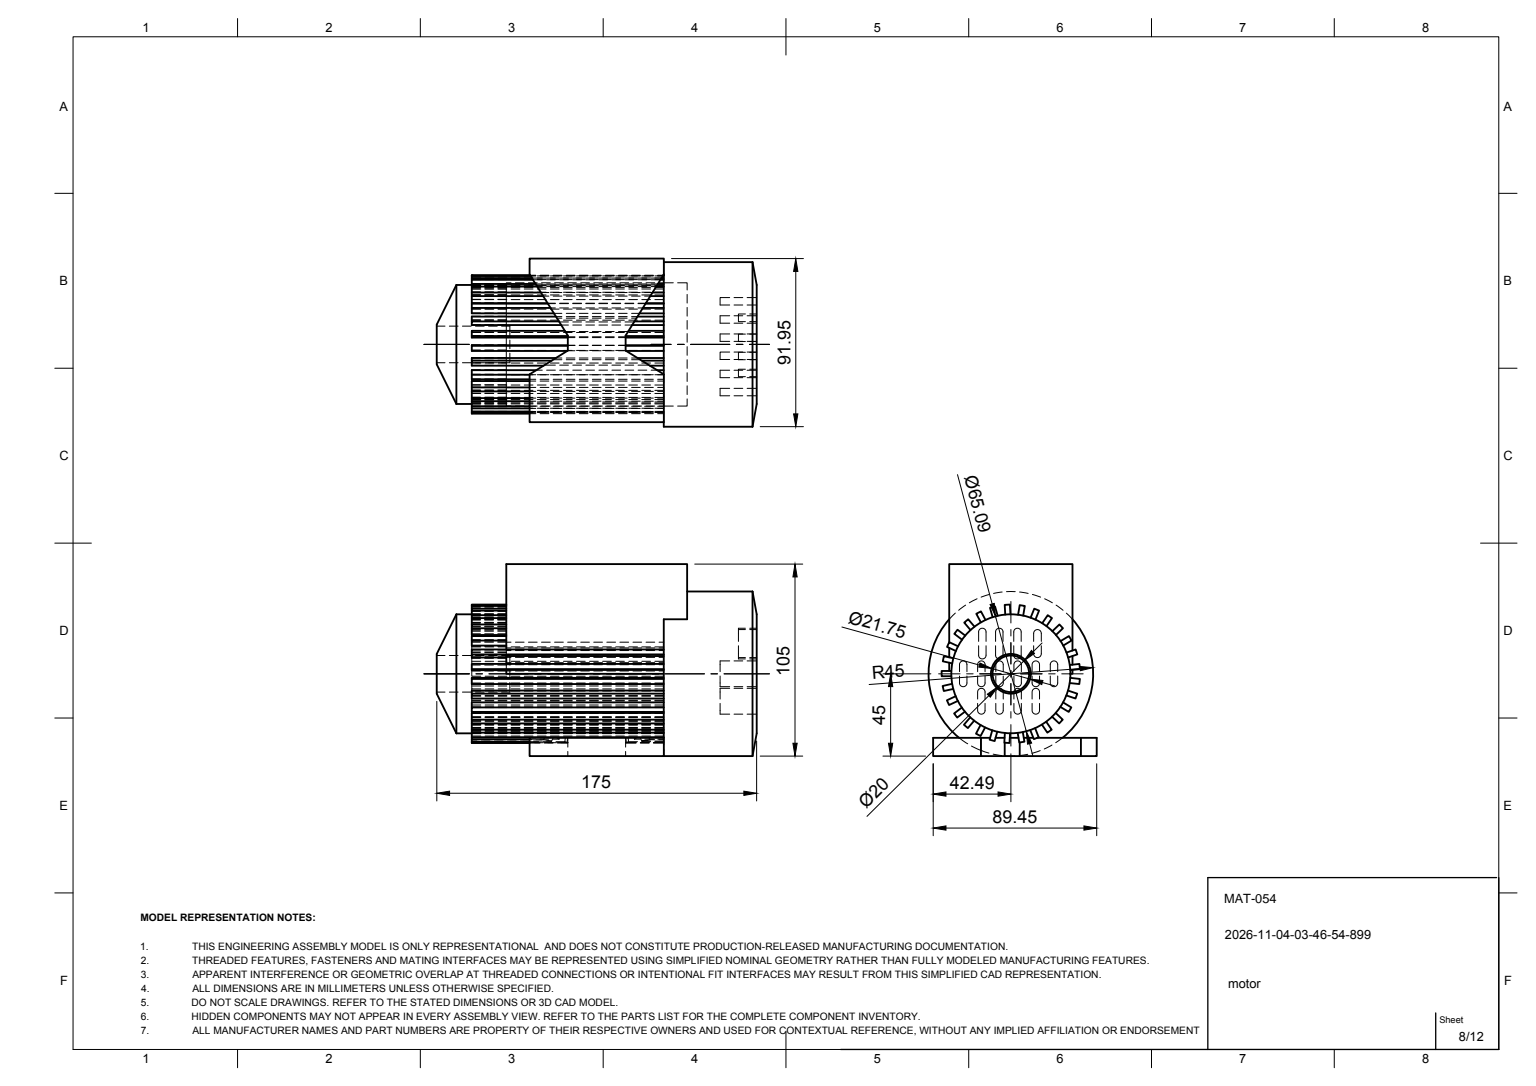
ISO-10303-21;
HEADER;
FILE_DESCRIPTION (('STEP AP214'),
    '1' );
FILE_NAME ('motor.step',
    '2026-10-21T17:50:41',
    ( '' ),
    ( '' ),
    'SwSTEP 2.0',
    'SolidWorks 2026',
    '' );
FILE_SCHEMA (( 'AUTOMOTIVE_DESIGN' ));
ENDSEC;

DATA;
#2=ORIENTED_EDGE ( 'NONE', *, *, #27963, .F. ) ;
#5=CARTESIAN_POINT ( 'NONE',  ( 15.44711578872680846, -28.64595934308655956, 68.31122994652405112 ) ) ;
#24=ADVANCED_FACE ( 'NONE', ( #3974 ), #8982, .F. ) ;
#30=CARTESIAN_POINT ( 'NONE',  ( -23.78520691327551972, 22.21414650552148728, 68.31122994652405112 ) ) ;
#31=EDGE_CURVE ( 'NONE', #27481, #20981, #20374, .T. ) ;
#32=LINE ( 'NONE', #10895, #9078 ) ;
#36=DIRECTION ( 'NONE',  ( -0.4198891015602645438, 0.9075754196709571175, 0.000000000000000000 ) ) ;
#44=CARTESIAN_POINT ( 'NONE',  ( -5.021133111225092982, -15.68591377522703745, -67.50000000000000000 ) ) ;
#46=LINE ( 'NONE', #29597, #32142 ) ;
#59=ORIENTED_EDGE ( 'NONE', *, *, #18290, .T. ) ;
#62=ORIENTED_EDGE ( 'NONE', *, *, #19345, .T. ) ;
#65=PLANE ( 'NONE',  #4223 ) ;
#67=AXIS2_PLACEMENT_3D ( 'NONE', #32973, #22315, #1132 ) ;
#69=ADVANCED_FACE ( 'NONE', ( #20027 ), #30867, .F. ) ;
#70=DIRECTION ( 'NONE',  ( -0.9766205557100867685, 0.2149704402110236834, 3.948942922735914076E-17 ) ) ;
#75=FACE_OUTER_BOUND ( 'NONE', #24485, .T. ) ;
#77=CARTESIAN_POINT ( 'NONE',  ( 3.235562306570555532E-30, -1.691831803474588058, -87.50000000000000000 ) ) ;
#85=AXIS2_PLACEMENT_3D ( 'NONE', #752, #27973, #1103 ) ;
#86=CARTESIAN_POINT ( 'NONE',  ( -20.02113311122498729, -5.758675521474015291, -67.50000000000000000 ) ) ;
#92=ORIENTED_EDGE ( 'NONE', *, *, #10815, .F. ) ;
#99=CARTESIAN_POINT ( 'NONE',  ( -45.00000000000000000, 16.36947364650383818, 36.69637551990492597 ) ) ;
#110=VECTOR ( 'NONE', #12286, 1000.000000000000227 ) ;
#121=EDGE_CURVE ( 'NONE', #19542, #7373, #4262, .T. ) ;
#122=CARTESIAN_POINT ( 'NONE',  ( -35.00000000000000000, -46.95407462254104303, -36.69637551990492597 ) ) ;
#126=LINE ( 'NONE', #30027, #31126 ) ;
#133=ORIENTED_EDGE ( 'NONE', *, *, #21122, .F. ) ;
#136=EDGE_LOOP ( 'NONE', ( #10690, #4855, #133, #33486, #30185, #13307, #10749, #25225 ) ) ;
#141=CARTESIAN_POINT ( 'NONE',  ( 28.11866956577618382, 16.38733641342591696, 68.31122994652405112 ) ) ;
#142=DIRECTION ( 'NONE',  ( 0.05413890858541774848, -0.9985334138511239299, -1.834276123671687566E-16 ) ) ;
#146=CARTESIAN_POINT ( 'NONE',  ( -9.978866888775527855, 8.235406450278430768, -87.50000000000000000 ) ) ;
#149=CARTESIAN_POINT ( 'NONE',  ( 3.235562306570555532E-30, 28.08988295778447508, -67.50000000000000000 ) ) ;
#150=EDGE_CURVE ( 'NONE', #25913, #33864, #29280, .T. ) ;
#158=VECTOR ( 'NONE', #14520, 1000.000000000000000 ) ;
#167=DIRECTION ( 'NONE',  ( 0.000000000000000000, 1.000000000000000000, 0.000000000000000000 ) ) ;
#177=ORIENTED_EDGE ( 'NONE', *, *, #24168, .F. ) ;
#180=FACE_OUTER_BOUND ( 'NONE', #24704, .T. ) ;
#189=AXIS2_PLACEMENT_3D ( 'NONE', #223, #13410, #11088 ) ;
#197=VECTOR ( 'NONE', #17016, 1000.000000000000000 ) ;
#200=CARTESIAN_POINT ( 'NONE',  ( -35.71762877834949990, -12.58147180936565057, -36.68877005347593467 ) ) ;
#214=CARTESIAN_POINT ( 'NONE',  ( -20.02113311122498729, -3.725253662474303784, -67.50000000000000000 ) ) ;
#215=LINE ( 'NONE', #29415, #4585 ) ;
#222=EDGE_CURVE ( 'NONE', #22062, #30310, #29769, .T. ) ;
#223=CARTESIAN_POINT ( 'NONE',  ( 0.000000000000000000, 3.524919873834583163E-15, 68.31122994652405112 ) ) ;
#232=EDGE_CURVE ( 'NONE', #29036, #32413, #15921, .T. ) ;
#243=CARTESIAN_POINT ( 'NONE',  ( 22.89764159710611224, 17.63622956525712127, -77.50000000000000000 ) ) ;
#244=ORIENTED_EDGE ( 'NONE', *, *, #13986, .T. ) ;
#252=ORIENTED_EDGE ( 'NONE', *, *, #16950, .T. ) ;
#253=EDGE_CURVE ( 'NONE', #5102, #23161, #21417, .T. ) ;
#254=CARTESIAN_POINT ( 'NONE',  ( 32.30227131129396412, -3.970848902647437395, 68.31122994652405112 ) ) ;
#255=DIRECTION ( 'NONE',  ( -0.3701381553399132329, -0.9289767198167918627, 0.000000000000000000 ) ) ;
#261=LINE ( 'NONE', #33170, #9980 ) ;
#268=CARTESIAN_POINT ( 'NONE',  ( 5.021133111224369117, -1.691831803474588058, -87.50000000000000000 ) ) ;
#269=CARTESIAN_POINT ( 'NONE',  ( 0.000000000000000000, 6.992329373473909019E-15, 49.43553178847298568 ) ) ;
#271=FACE_OUTER_BOUND ( 'NONE', #6766, .T. ) ;
#282=CARTESIAN_POINT ( 'NONE',  ( -35.00000000000000000, 0.000000000000000000, 0.000000000000000000 ) ) ;
#286=ORIENTED_EDGE ( 'NONE', *, *, #4793, .F. ) ;
#288=AXIS2_PLACEMENT_3D ( 'NONE', #34150, #4414, #26138 ) ;
#298=ORIENTED_EDGE ( 'NONE', *, *, #4872, .T. ) ;
#303=DIRECTION ( 'NONE',  ( -0.9985334138511239299, -0.05413890858541774848, -0.000000000000000000 ) ) ;
#308=ORIENTED_EDGE ( 'NONE', *, *, #21108, .F. ) ;
#311=DIRECTION ( 'NONE',  ( 0.000000000000000000, -0.000000000000000000, -1.000000000000000000 ) ) ;
#318=CARTESIAN_POINT ( 'NONE',  ( 32.40067729534749219, 3.066020821660472517, 68.31122994652405112 ) ) ;
#319=VERTEX_POINT ( 'NONE', #27272 ) ;
#323=EDGE_CURVE ( 'NONE', #17531, #2097, #46, .T. ) ;
#324=EDGE_CURVE ( 'NONE', #31410, #8890, #5192, .T. ) ;
#327=DIRECTION ( 'NONE',  ( -0.000000000000000000, -1.000000000000000000, -0.000000000000000000 ) ) ;
#331=ORIENTED_EDGE ( 'NONE', *, *, #24983, .F. ) ;
#336=ORIENTED_EDGE ( 'NONE', *, *, #6534, .F. ) ;
#340=CARTESIAN_POINT ( 'NONE',  ( 3.235562306570555532E-30, -1.691831803474591833, -67.50000000000000000 ) ) ;
#346=ORIENTED_EDGE ( 'NONE', *, *, #29604, .F. ) ;
#353=CARTESIAN_POINT ( 'NONE',  ( 5.021133111224679091, 26.05646109878476224, -67.50000000000000000 ) ) ;
#357=ORIENTED_EDGE ( 'NONE', *, *, #28689, .F. ) ;
#360=CYLINDRICAL_SURFACE ( 'NONE', #25416, 2.033421858999710619 ) ;
#361=EDGE_CURVE ( 'NONE', #12124, #30243, #11090, .T. ) ;
#363=ORIENTED_EDGE ( 'NONE', *, *, #34633, .T. ) ;
#369=CARTESIAN_POINT ( 'NONE',  ( 22.89764159710613001, 8.346743312457581609, -87.50000000000000000 ) ) ;
#371=PLANE ( 'NONE',  #32639 ) ;
#374=AXIS2_PLACEMENT_3D ( 'NONE', #31781, #29476, #5070 ) ;
#383=VECTOR ( 'NONE', #16250, 1000.000000000000114 ) ;
#394=CARTESIAN_POINT ( 'NONE',  ( -36.80830595996284416, 8.862931941313791029, -36.68877005347593467 ) ) ;
#399=DIRECTION ( 'NONE',  ( 0.000000000000000000, 1.836970198721029934E-16, -1.000000000000000000 ) ) ;
#409=CARTESIAN_POINT ( 'NONE',  ( -2.216215597024039141, -32.46987467335852529, 68.31122994652405112 ) ) ;
#410=AXIS2_PLACEMENT_3D ( 'NONE', #353, #702, #3357 ) ;
#412=ORIENTED_EDGE ( 'NONE', *, *, #6672, .F. ) ;
#415=EDGE_CURVE ( 'NONE', #2863, #31849, #8577, .T. ) ;
#419=VECTOR ( 'NONE', #14183, 1000.000000000000000 ) ;
#420=ORIENTED_EDGE ( 'NONE', *, *, #12622, .F. ) ;
#424=ORIENTED_EDGE ( 'NONE', *, *, #23285, .T. ) ;
#425=CARTESIAN_POINT ( 'NONE',  ( -18.45373714011839539, 26.80790850550480897, 68.31122994652405112 ) ) ;
#427=CIRCLE ( 'NONE', #22026, 10.00000000000000000 ) ;
#431=ORIENTED_EDGE ( 'NONE', *, *, #25232, .F. ) ;
#433=LINE ( 'NONE', #254, #17985 ) ;
#434=DIRECTION ( 'NONE',  ( 0.000000000000000000, 1.836970198721029441E-16, -1.000000000000000000 ) ) ;
#436=DIRECTION ( 'NONE',  ( -1.000000000000000000, 0.000000000000000000, 0.000000000000000000 ) ) ;
#439=VECTOR ( 'NONE', #21313, 1000.000000000000000 ) ;
#442=EDGE_CURVE ( 'NONE', #2071, #22576, #14652, .T. ) ;
#444=ORIENTED_EDGE ( 'NONE', *, *, #6797, .F. ) ;
#446=EDGE_CURVE ( 'NONE', #17949, #8883, #28157, .T. ) ;
#449=DIRECTION ( 'NONE',  ( 0.4198891015602635446, -0.9075754196709575616, -1.667188999027280528E-16 ) ) ;
#452=FACE_OUTER_BOUND ( 'NONE', #26260, .T. ) ;
#456=AXIS2_PLACEMENT_3D ( 'NONE', #31514, #16040, #10517 ) ;
#479=PLANE ( 'NONE',  #16043 ) ;
#484=DIRECTION ( 'NONE',  ( -1.000000000000000000, 0.000000000000000000, 0.000000000000000000 ) ) ;
#488=CARTESIAN_POINT ( 'NONE',  ( -32.54223829851967764, 0.4550817492056100644, 68.31122994652405112 ) ) ;
#489=ADVANCED_FACE ( 'NONE', ( #1969 ), #7124, .F. ) ;
#494=EDGE_CURVE ( 'NONE', #32940, #29402, #33851, .T. ) ;
#504=PLANE ( 'NONE',  #30798 ) ;
#511=AXIS2_PLACEMENT_3D ( 'NONE', #21319, #32167, #30028 ) ;
#522=EDGE_CURVE ( 'NONE', #24257, #22309, #20328, .T. ) ;
#523=ADVANCED_FACE ( 'NONE', ( #31345 ), #4279, .F. ) ;
#532=ORIENTED_EDGE ( 'NONE', *, *, #11905, .T. ) ;
#538=CARTESIAN_POINT ( 'NONE',  ( -10.84269519964070305, -36.27449394610876965, -36.68877005347593467 ) ) ;
#539=CARTESIAN_POINT ( 'NONE',  ( 14.14940496480368104, 33.69708579775584667, -36.68877005347592757 ) ) ;
#544=CARTESIAN_POINT ( 'NONE',  ( -9.144464960067640646, -31.23432620483743705, -36.68877005347593467 ) ) ;
#548=ORIENTED_EDGE ( 'NONE', *, *, #30977, .T. ) ;
#552=PRODUCT_CONTEXT ( 'NONE', #11461, 'mechanical' ) ;
#557=EDGE_CURVE ( 'NONE', #31368, #17595, #13969, .T. ) ;
#562=EDGE_LOOP ( 'NONE', ( #7226, #23075, #30348, #6330 ) ) ;
#565=EDGE_CURVE ( 'NONE', #34117, #30722, #12848, .T. ) ;
#572=PLANE ( 'NONE',  #2099 ) ;
#578=DIRECTION ( 'NONE',  ( 0.000000000000000000, 0.000000000000000000, 1.000000000000000000 ) ) ;
#584=VECTOR ( 'NONE', #33294, 1000.000000000000000 ) ;
#585=ORIENTED_EDGE ( 'NONE', *, *, #9500, .F. ) ;
#590=EDGE_LOOP ( 'NONE', ( #5300, #9615, #21290, #22102 ) ) ;
#592=LINE ( 'NONE', #30312, #24116 ) ;
#593=EDGE_CURVE ( 'NONE', #33757, #32360, #20496, .T. ) ;
#594=VERTEX_POINT ( 'NONE', #20673 ) ;
#609=DIRECTION ( 'NONE',  ( -0.000000000000000000, 1.836970198721029934E-16, -1.000000000000000000 ) ) ;
#611=ADVANCED_FACE ( 'NONE', ( #2493 ), #8368, .F. ) ;
#614=PLANE ( 'NONE',  #25375 ) ;
#616=LINE ( 'NONE', #2922, #2449 ) ;
#619=AXIS2_PLACEMENT_3D ( 'NONE', #1312, #12183, #23029 ) ;
#624=LINE ( 'NONE', #9159, #6292 ) ;
#631=EDGE_LOOP ( 'NONE', ( #17739, #3820, #7539, #1701 ) ) ;
#633=EDGE_LOOP ( 'NONE', ( #9077, #27367, #24881, #22906, #2998 ) ) ;
#634=EDGE_CURVE ( 'NONE', #13940, #4555, #21191, .T. ) ;
#635=EDGE_CURVE ( 'NONE', #21072, #3784, #32561, .T. ) ;
#640=VERTEX_POINT ( 'NONE', #13541 ) ;
#641=DIRECTION ( 'NONE',  ( -0.000000000000000000, 1.836970198721029934E-16, -1.000000000000000000 ) ) ;
#646=ORIENTED_EDGE ( 'NONE', *, *, #2039, .T. ) ;
#653=LINE ( 'NONE', #18869, #7882 ) ;
#659=ORIENTED_EDGE ( 'NONE', *, *, #951, .T. ) ;
#661=LINE ( 'NONE', #835, #20287 ) ;
#662=DIRECTION ( 'NONE',  ( 0.000000000000000000, 1.000000000000000000, 0.000000000000000000 ) ) ;
#663=AXIS2_PLACEMENT_3D ( 'NONE', #15533, #26376, #17867 ) ;
#675=VECTOR ( 'NONE', #22343, 1000.000000000000114 ) ;
#679=EDGE_CURVE ( 'NONE', #33018, #4776, #8184, .T. ) ;
#685=ORIENTED_EDGE ( 'NONE', *, *, #27268, .F. ) ;
#700=ORIENTED_EDGE ( 'NONE', *, *, #24646, .F. ) ;
#702=DIRECTION ( 'NONE',  ( -0.000000000000000000, 1.836970198721029934E-16, -1.000000000000000000 ) ) ;
#708=EDGE_LOOP ( 'NONE', ( #10396, #12384, #6662, #7529 ) ) ;
#712=DIRECTION ( 'NONE',  ( -0.000000000000000000, 1.836970198721029688E-16, -1.000000000000000000 ) ) ;
#725=AXIS2_PLACEMENT_3D ( 'NONE', #32125, #31776, #7740 ) ;
#732=CARTESIAN_POINT ( 'NONE',  ( 3.985664461616345376E-15, 32.54542015209057837, -87.50000000000000000 ) ) ;
#736=VERTEX_POINT ( 'NONE', #13710 ) ;
#738=DIRECTION ( 'NONE',  ( -0.8568571761675883858, 0.5155538571770231782, 9.470570714698694973E-17 ) ) ;
#741=FACE_OUTER_BOUND ( 'NONE', #26082, .T. ) ;
#749=VECTOR ( 'NONE', #31002, 1000.000000000000000 ) ;
#750=VERTEX_POINT ( 'NONE', #16577 ) ;
#752=CARTESIAN_POINT ( 'NONE',  ( 10.96230482721425403, -14.55883922869198344, -77.50000000000000000 ) ) ;
#772=ORIENTED_EDGE ( 'NONE', *, *, #29347, .F. ) ;
#786=CIRCLE ( 'NONE', #28069, 2.033421858999711507 ) ;
#787=DIRECTION ( 'NONE',  ( 0.000000000000000000, 1.836970198721029441E-16, -1.000000000000000000 ) ) ;
#790=FACE_OUTER_BOUND ( 'NONE', #10832, .T. ) ;
#791=LINE ( 'NONE', #11664, #19521 ) ;
#796=CARTESIAN_POINT ( 'NONE',  ( 12.46788440507149964, 30.06253867087536946, 68.31122994652405112 ) ) ;
#799=FACE_OUTER_BOUND ( 'NONE', #15356, .T. ) ;
#802=VERTEX_POINT ( 'NONE', #25076 ) ;
#804=DIRECTION ( 'NONE',  ( 0.000000000000000000, 1.000000000000000000, 0.000000000000000000 ) ) ;
#805=DIRECTION ( 'NONE',  ( 0.000000000000000000, 0.000000000000000000, 1.000000000000000000 ) ) ;
#806=EDGE_CURVE ( 'NONE', #26021, #12216, #16751, .T. ) ;
#808=AXIS2_PLACEMENT_3D ( 'NONE', #12779, #23621, #34477 ) ;
#810=ORIENTED_EDGE ( 'NONE', *, *, #19374, .T. ) ;
#815=CARTESIAN_POINT ( 'NONE',  ( -35.00000000000000000, -4.831299144296466785, 15.81122994652406355 ) ) ;
#828=LINE ( 'NONE', #27867, #26026 ) ;
#834=ORIENTED_EDGE ( 'NONE', *, *, #5373, .F. ) ;
#835=CARTESIAN_POINT ( 'NONE',  ( -36.04853892210773836, 11.59936550071286376, 68.31122994652405112 ) ) ;
#848=VECTOR ( 'NONE', #31003, 1000.000000000000000 ) ;
#852=LINE ( 'NONE', #22571, #25306 ) ;
#858=EDGE_CURVE ( 'NONE', #7203, #16288, #5854, .T. ) ;
#860=FACE_OUTER_BOUND ( 'NONE', #11273, .T. ) ;
#863=CARTESIAN_POINT ( 'NONE',  ( -28.00450684652667022, 16.58167570419056247, -36.68877005347593467 ) ) ;
#865=DIRECTION ( 'NONE',  ( 0.000000000000000000, -1.000000000000000000, -1.836970198721029934E-16 ) ) ;
#866=FACE_OUTER_BOUND ( 'NONE', #16501, .T. ) ;
#869=ORIENTED_EDGE ( 'NONE', *, *, #27770, .T. ) ;
#870=CARTESIAN_POINT ( 'NONE',  ( 10.62930655775863364, -36.34639295086972766, 68.31122994652405112 ) ) ;
#872=EDGE_CURVE ( 'NONE', #17833, #17981, #14432, .T. ) ;
#880=ORIENTED_EDGE ( 'NONE', *, *, #150, .F. ) ;
#885=ORIENTED_EDGE ( 'NONE', *, *, #10951, .F. ) ;
#891=CARTESIAN_POINT ( 'NONE',  ( 22.89764159710615132, -1.579009122040562207, -77.50000000000000000 ) ) ;
#893=EDGE_CURVE ( 'NONE', #25849, #6490, #16930, .T. ) ;
#894=LINE ( 'NONE', #11935, #25790 ) ;
#902=EDGE_CURVE ( 'NONE', #26131, #14276, #11579, .T. ) ;
#906=ORIENTED_EDGE ( 'NONE', *, *, #16042, .T. ) ;
#913=VECTOR ( 'NONE', #9835, 1000.000000000000000 ) ;
#917=ORIENTED_EDGE ( 'NONE', *, *, #6958, .T. ) ;
#937=EDGE_CURVE ( 'NONE', #22497, #8202, #34818, .T. ) ;
#943=VECTOR ( 'NONE', #26555, 1000.000000000000000 ) ;
#950=ORIENTED_EDGE ( 'NONE', *, *, #18415, .F. ) ;
#951=EDGE_CURVE ( 'NONE', #29695, #26014, #34640, .T. ) ;
#952=FACE_OUTER_BOUND ( 'NONE', #1655, .T. ) ;
#960=CARTESIAN_POINT ( 'NONE',  ( 15.44711578872682267, -28.64595934308655600, 68.31122994652405112 ) ) ;
#963=EDGE_CURVE ( 'NONE', #18812, #2924, #2407, .T. ) ;
#976=DIRECTION ( 'NONE',  ( 0.000000000000000000, -1.000000000000000000, -1.836970198721029934E-16 ) ) ;
#979=DIRECTION ( 'NONE',  ( -0.000000000000000000, -0.000000000000000000, -1.000000000000000000 ) ) ;
#996=CARTESIAN_POINT ( 'NONE',  ( -9.978866888775426602, 14.09580098603202458, -67.50000000000000000 ) ) ;
#997=AXIS2_PLACEMENT_3D ( 'NONE', #20960, #9749, #4739 ) ;
#999=CARTESIAN_POINT ( 'NONE',  ( 0.000000000000000000, -33.69708579775584667, 49.43553178847298568 ) ) ;
#1003=EDGE_CURVE ( 'NONE', #17724, #17949, #11737, .T. ) ;
#1004=CARTESIAN_POINT ( 'NONE',  ( 8.986540508143580297, 33.69708579775584667, 68.31122994652405112 ) ) ;
#1012=AXIS2_PLACEMENT_3D ( 'NONE', #21639, #26986, #3122 ) ;
#1015=EDGE_CURVE ( 'NONE', #2086, #14870, #28769, .T. ) ;
#1022=CARTESIAN_POINT ( 'NONE',  ( 22.89764159710611224, 17.63622956525712482, -87.50000000000000000 ) ) ;
#1024=DIRECTION ( 'NONE',  ( 0.000000000000000000, 1.836970198721029441E-16, -1.000000000000000000 ) ) ;
#1029=DIRECTION ( 'NONE',  ( -0.000000000000000000, -0.000000000000000000, -1.000000000000000000 ) ) ;
#1037=AXIS2_PLACEMENT_3D ( 'NONE', #21545, #32381, #7826 ) ;
#1040=DIRECTION ( 'NONE',  ( 0.8835120444460231592, -0.4684084406997896521, -0.000000000000000000 ) ) ;
#1041=VERTEX_POINT ( 'NONE', #2236 ) ;
#1043=AXIS2_PLACEMENT_3D ( 'NONE', #2995, #22054, #19392 ) ;
#1045=DIRECTION ( 'NONE',  ( 0.000000000000000000, 1.000000000000000000, 0.000000000000000000 ) ) ;
#1050=CARTESIAN_POINT ( 'NONE',  ( -11.83261234297099662, -30.31820670846268229, 68.31122994652405112 ) ) ;
#1053=CARTESIAN_POINT ( 'NONE',  ( 32.81769769215652133, 18.87860345536237006, 49.43553178847298568 ) ) ;
#1063=ADVANCED_FACE ( 'NONE', ( #13287 ), #10427, .F. ) ;
#1074=ORIENTED_EDGE ( 'NONE', *, *, #12659, .T. ) ;
#1075=ADVANCED_FACE ( 'NONE', ( #32306 ), #1883, .T. ) ;
#1079=DIRECTION ( 'NONE',  ( 0.000000000000000000, 1.836970198721029441E-16, -1.000000000000000000 ) ) ;
#1081=VECTOR ( 'NONE', #9547, 1000.000000000000000 ) ;
#1083=CARTESIAN_POINT ( 'NONE',  ( -31.48191842954600617, 28.04684603917314334, 55.43429723762557870 ) ) ;
#1085=ORIENTED_EDGE ( 'NONE', *, *, #12660, .T. ) ;
#1090=ORIENTED_EDGE ( 'NONE', *, *, #16252, .F. ) ;
#1091=CARTESIAN_POINT ( 'NONE',  ( 18.63894936814906700, 26.67946662374790279, 68.31122994652405112 ) ) ;
#1098=DIRECTION ( 'NONE',  ( 0.000000000000000000, 1.000000000000000000, 0.000000000000000000 ) ) ;
#1101=VERTEX_POINT ( 'NONE', #8456 ) ;
#1103=DIRECTION ( 'NONE',  ( 0.000000000000000000, 1.000000000000000000, 0.000000000000000000 ) ) ;
#1104=EDGE_CURVE ( 'NONE', #20048, #7819, #2582, .T. ) ;
#1110=DIRECTION ( 'NONE',  ( -1.000000000000000000, 6.792721752314501023E-48, -3.697785493223492838E-32 ) ) ;
#1121=EDGE_CURVE ( 'NONE', #18879, #2754, #13627, .T. ) ;
#1123=DIRECTION ( 'NONE',  ( 0.000000000000000000, -1.000000000000000000, -1.541976423090495633E-16 ) ) ;
#1126=CARTESIAN_POINT ( 'NONE',  ( 22.89764159710613001, 8.346743312457579833, -77.50000000000000000 ) ) ;
#1132=DIRECTION ( 'NONE',  ( 0.000000000000000000, 1.000000000000000000, 0.000000000000000000 ) ) ;
#1134=VERTEX_POINT ( 'NONE', #8277 ) ;
#1137=DIRECTION ( 'NONE',  ( 0.000000000000000000, 0.000000000000000000, 1.000000000000000000 ) ) ;
#1143=DIRECTION ( 'NONE',  ( -0.000000000000000000, 1.836970198721029934E-16, -1.000000000000000000 ) ) ;
#1152=DIRECTION ( 'NONE',  ( -0.5155538571770220679, -0.8568571761675890519, 0.000000000000000000 ) ) ;
#1153=CARTESIAN_POINT ( 'NONE',  ( -45.00000000000000000, 16.36947364650383818, -36.69637551990492597 ) ) ;
#1156=CARTESIAN_POINT ( 'NONE',  ( -9.978866888775426602, 16.12922284503173742, -67.50000000000000000 ) ) ;
#1165=VERTEX_POINT ( 'NONE', #28559 ) ;
#1172=VERTEX_POINT ( 'NONE', #8805 ) ;
#1194=VERTEX_POINT ( 'NONE', #6123 ) ;
#1197=DIRECTION ( 'NONE',  ( 0.000000000000000000, 1.836970198721029934E-16, -1.000000000000000000 ) ) ;
#1204=AXIS2_PLACEMENT_3D ( 'NONE', #9772, #34683, #18511 ) ;
#1216=ORIENTED_EDGE ( 'NONE', *, *, #1754, .T. ) ;
#1237=DIRECTION ( 'NONE',  ( -1.000000000000000000, -0.000000000000000000, -0.000000000000000000 ) ) ;
#1241=DIRECTION ( 'NONE',  ( 1.000000000000000000, 0.000000000000000000, -0.000000000000000000 ) ) ;
#1249=ORIENTED_EDGE ( 'NONE', *, *, #11405, .T. ) ;
#1259=VECTOR ( 'NONE', #25566, 1000.000000000000000 ) ;
#1262=EDGE_CURVE ( 'NONE', #12124, #6786, #12904, .T. ) ;
#1263=DIRECTION ( 'NONE',  ( 1.000000000000000000, 0.000000000000000000, 0.000000000000000000 ) ) ;
#1267=DIRECTION ( 'NONE',  ( 0.000000000000000000, 1.836970198721029441E-16, -1.000000000000000000 ) ) ;
#1268=DIRECTION ( 'NONE',  ( 0.000000000000000000, 1.000000000000000000, 1.836970198721029688E-16 ) ) ;
#1269=DIRECTION ( 'NONE',  ( -0.000000000000000000, 1.836970198721029688E-16, -1.000000000000000000 ) ) ;
#1270=ORIENTED_EDGE ( 'NONE', *, *, #9403, .T. ) ;
#1272=DIRECTION ( 'NONE',  ( 1.000000000000000000, 0.000000000000000000, 0.000000000000000000 ) ) ;
#1275=DIRECTION ( 'NONE',  ( 0.000000000000000000, 1.836970198721029688E-16, -1.000000000000000000 ) ) ;
#1276=CARTESIAN_POINT ( 'NONE',  ( -32.32899628990713126, -3.747048406849335045, -36.68877005347593467 ) ) ;
#1291=ORIENTED_EDGE ( 'NONE', *, *, #6612, .T. ) ;
#1292=EDGE_CURVE ( 'NONE', #7906, #11190, #17556, .T. ) ;
#1301=ORIENTED_EDGE ( 'NONE', *, *, #28459, .F. ) ;
#1308=AXIS2_PLACEMENT_3D ( 'NONE', #23598, #4889, #7035 ) ;
#1312=CARTESIAN_POINT ( 'NONE',  ( 5.021133111224162171, -21.54630831098063837, -67.50000000000000000 ) ) ;
#1316=CARTESIAN_POINT ( 'NONE',  ( 0.000000000000000000, 6.992329373473909019E-15, 49.43553178847298568 ) ) ;
#1327=ADVANCED_FACE ( 'NONE', ( #34422 ), #4667, .F. ) ;
#1343=ORIENTED_EDGE ( 'NONE', *, *, #33236, .F. ) ;
#1356=CARTESIAN_POINT ( 'NONE',  ( 13.32059394339353986, -35.43959265050634144, 68.31122994652405112 ) ) ;
#1357=CARTESIAN_POINT ( 'NONE',  ( -35.00000000000000000, -12.29554237047778997, 68.31122994652405112 ) ) ;
#1363=DIRECTION ( 'NONE',  ( -0.7960930657056428661, 0.6051742151937663516, -0.000000000000000000 ) ) ;
#1365=FACE_OUTER_BOUND ( 'NONE', #7788, .T. ) ;
#1368=CARTESIAN_POINT ( 'NONE',  ( 26.04754872656010889, -19.51229300245305964, 68.31122994652405112 ) ) ;
#1376=VERTEX_POINT ( 'NONE', #2023 ) ;
#1383=CARTESIAN_POINT ( 'NONE',  ( 5.021133111224369117, -3.725253662474303784, -67.50000000000000000 ) ) ;
#1386=VECTOR ( 'NONE', #1768, 1000.000000000000000 ) ;
#1405=EDGE_CURVE ( 'NONE', #18566, #13343, #4853, .T. ) ;
#1418=UNCERTAINTY_MEASURE_WITH_UNIT (LENGTH_MEASURE( 1.000000000000000082E-05 ), #3776, 'distance_accuracy_value', 'NONE');
#1422=ORIENTED_EDGE ( 'NONE', *, *, #4993, .T. ) ;
#1425=DIRECTION ( 'NONE',  ( -1.000000000000000000, 6.792721752314501023E-48, -3.697785493223492838E-32 ) ) ;
#1426=VECTOR ( 'NONE', #28156, 1000.000000000000000 ) ;
#1429=AXIS2_PLACEMENT_3D ( 'NONE', #14786, #26313, #23469 ) ;
#1431=CARTESIAN_POINT ( 'NONE',  ( 24.11848021413632992, 29.19488569250028220, 68.31122994652405112 ) ) ;
#1434=CARTESIAN_POINT ( 'NONE',  ( -35.00000000000000000, 3.353962854566122864, -15.81122994652406355 ) ) ;
#1440=CARTESIAN_POINT ( 'NONE',  ( 5.713835024271039842, 32.03991982186465748, 68.31122994652405112 ) ) ;
#1441=DIRECTION ( 'NONE',  ( 0.000000000000000000, 1.000000000000000000, 0.000000000000000000 ) ) ;
#1442=ORIENTED_EDGE ( 'NONE', *, *, #2873, .F. ) ;
#1443=VECTOR ( 'NONE', #16868, 1000.000000000000000 ) ;
#1444=DIRECTION ( 'NONE',  ( -0.1081190184239417262, -0.9941379571543595972, 0.000000000000000000 ) ) ;
#1445=VECTOR ( 'NONE', #24810, 1000.000000000000227 ) ;
#1452=CARTESIAN_POINT ( 'NONE',  ( 29.44023756548696369, 13.87360028845404969, 68.31122994652405112 ) ) ;
#1453=DIRECTION ( 'NONE',  ( 1.000000000000000000, -0.000000000000000000, -0.000000000000000000 ) ) ;
#1455=AXIS2_PLACEMENT_3D ( 'NONE', #33240, #1029, #22384 ) ;
#1485=CARTESIAN_POINT ( 'NONE',  ( 22.89764159710611224, 13.56412600238610366, -77.50000000000000000 ) ) ;
#1491=ORIENTED_EDGE ( 'NONE', *, *, #27268, .T. ) ;
#1500=ADVANCED_FACE ( 'NONE', ( #24072 ), #21425, .T. ) ;
#1504=DIRECTION ( 'NONE',  ( 0.7960930657056439763, -0.6051742151937649083, -1.111686998345333706E-16 ) ) ;
#1506=ORIENTED_EDGE ( 'NONE', *, *, #19153, .T. ) ;
#1523=CARTESIAN_POINT ( 'NONE',  ( -45.00000000000000000, -46.95407462254104303, -36.69637551990492597 ) ) ;
#1525=CARTESIAN_POINT ( 'NONE',  ( -5.021133111224782120, 18.16264470403145381, -87.50000000000000000 ) ) ;
#1526=EDGE_LOOP ( 'NONE', ( #14624, #22210, #8293, #29863 ) ) ;
#1528=LINE ( 'NONE', #26245, #13393 ) ;
#1530=DIRECTION ( 'NONE',  ( 0.1081190184239421009, -0.9941379571543595972, 0.000000000000000000 ) ) ;
#1533=VERTEX_POINT ( 'NONE', #6134 ) ;
#1536=ORIENTED_EDGE ( 'NONE', *, *, #13345, .F. ) ;
#1547=VECTOR ( 'NONE', #10685, 1000.000000000000000 ) ;
#1555=ORIENTED_EDGE ( 'NONE', *, *, #18031, .F. ) ;
#1559=ADVANCED_FACE ( 'NONE', ( #27856 ), #3466, .F. ) ;
#1561=ADVANCED_FACE ( 'NONE', ( #6668 ), #17563, .T. ) ;
#1565=VERTEX_POINT ( 'NONE', #25179 ) ;
#1577=ORIENTED_EDGE ( 'NONE', *, *, #13570, .F. ) ;
#1585=DIRECTION ( 'NONE',  ( 0.9766205557100867685, 0.2149704402110236834, 3.948942922735914076E-17 ) ) ;
#1587=DIRECTION ( 'NONE',  ( 0.000000000000000000, 1.000000000000000000, 0.000000000000000000 ) ) ;
#1589=EDGE_CURVE ( 'NONE', #5237, #5316, #28038, .T. ) ;
#1593=VECTOR ( 'NONE', #14428, 1000.000000000000000 ) ;
#1597=ADVANCED_FACE ( 'NONE', ( #34432 ), #28911, .F. ) ;
#1598=CIRCLE ( 'NONE', #5542, 32.54542015209055705 ) ;
#1600=LINE ( 'NONE', #23659, #4417 ) ;
#1606=DIRECTION ( 'NONE',  ( -0.4198891015602640997, -0.9075754196709572286, 0.000000000000000000 ) ) ;
#1607=CIRCLE ( 'NONE', #3885, 32.54542015209054995 ) ;
#1615=AXIS2_PLACEMENT_3D ( 'NONE', #9963, #23157, #20822 ) ;
#1620=CARTESIAN_POINT ( 'NONE',  ( 2.567399184519788768, -37.78162119159484433, -36.68877005347593467 ) ) ;
#1623=CARTESIAN_POINT ( 'NONE',  ( -5.021133111225092982, -11.61907005722761532, -67.50000000000000000 ) ) ;
#1639=VERTEX_POINT ( 'NONE', #1853 ) ;
#1645=FACE_OUTER_BOUND ( 'NONE', #15064, .T. ) ;
#1654=DIRECTION ( 'NONE',  ( 0.8835120444460229372, 0.4684084406997900407, -0.000000000000000000 ) ) ;
#1655=EDGE_LOOP ( 'NONE', ( #29027, #28886, #34662, #16670 ) ) ;
#1658=AXIS2_PLACEMENT_3D ( 'NONE', #31039, #31375, #3613 ) ;
#1660=ORIENTED_EDGE ( 'NONE', *, *, #33278, .F. ) ;
#1661=DIRECTION ( 'NONE',  ( 0.000000000000000000, 0.000000000000000000, -1.000000000000000000 ) ) ;
#1674=ORIENTED_EDGE ( 'NONE', *, *, #937, .F. ) ;
#1678=VECTOR ( 'NONE', #2137, 1000.000000000000000 ) ;
#1684=EDGE_CURVE ( 'NONE', #12202, #22339, #4337, .T. ) ;
#1701=ORIENTED_EDGE ( 'NONE', *, *, #32394, .F. ) ;
#1704=VERTEX_POINT ( 'NONE', #20733 ) ;
#1711=DIRECTION ( 'NONE',  ( 0.000000000000000000, 1.000000000000000000, 0.000000000000000000 ) ) ;
#1731=ADVANCED_FACE ( 'NONE', ( #23905, #34783, #32098, #7714, #18599, #29443, #5209, #10756, #16815, #24081, #24427, #7896, #8069, #19127, #8423 ), #13955, .F. ) ;
#1737=DIRECTION ( 'NONE',  ( 3.697785493223492838E-32, 1.934419779023891545E-16, -1.000000000000000000 ) ) ;
#1740=DIRECTION ( 'NONE',  ( -1.000000000000000000, 6.792721752314501023E-48, -3.697785493223492838E-32 ) ) ;
#1741=DIRECTION ( 'NONE',  ( 0.000000000000000000, -0.000000000000000000, -1.000000000000000000 ) ) ;
#1742=VERTEX_POINT ( 'NONE', #22131 ) ;
#1747=ORIENTED_EDGE ( 'NONE', *, *, #21577, .F. ) ;
#1752=FACE_OUTER_BOUND ( 'NONE', #33427, .T. ) ;
#1753=ADVANCED_FACE ( 'NONE', ( #18774 ), #29613, .F. ) ;
#1754=EDGE_CURVE ( 'NONE', #26155, #22562, #14485, .T. ) ;
#1755=VECTOR ( 'NONE', #29586, 1000.000000000000000 ) ;
#1756=CIRCLE ( 'NONE', #21651, 44.99999999999998579 ) ;
#1767=LINE ( 'NONE', #14967, #32858 ) ;
#1768=DIRECTION ( 'NONE',  ( 0.000000000000000000, 1.836970198721029441E-16, -1.000000000000000000 ) ) ;
#1775=CIRCLE ( 'NONE', #26215, 32.54542015209055705 ) ;
#1776=ORIENTED_EDGE ( 'NONE', *, *, #17601, .F. ) ;
#1777=ORIENTED_EDGE ( 'NONE', *, *, #16323, .F. ) ;
#1778=LINE ( 'NONE', #4964, #24830 ) ;
#1779=AXIS2_PLACEMENT_3D ( 'NONE', #30254, #8011, #30087 ) ;
#1781=VECTOR ( 'NONE', #20154, 1000.000000000000000 ) ;
#1788=DIRECTION ( 'NONE',  ( 0.000000000000000000, -1.000000000000000000, 0.000000000000000000 ) ) ;
#1791=ADVANCED_FACE ( 'NONE', ( #8591 ), #32443, .F. ) ;
#1806=ORIENTED_EDGE ( 'NONE', *, *, #16042, .F. ) ;
#1807=ORIENTED_EDGE ( 'NONE', *, *, #6445, .F. ) ;
#1813=DIRECTION ( 'NONE',  ( 0.2675283385292216987, -0.9635499925192227977, 0.000000000000000000 ) ) ;
#1815=CARTESIAN_POINT ( 'NONE',  ( -27.84632068199329780, 25.66368763279034226, 68.31122994652405112 ) ) ;
#1825=VECTOR ( 'NONE', #18332, 1000.000000000000114 ) ;
#1829=DIRECTION ( 'NONE',  ( 3.697785493223492838E-32, 1.934419779023891545E-16, -1.000000000000000000 ) ) ;
#1853=CARTESIAN_POINT ( 'NONE',  ( 60.00000000000000000, 33.69708579775584667, -49.43553178847298568 ) ) ;
#1855=ORIENTED_EDGE ( 'NONE', *, *, #15617, .T. ) ;
#1857=CARTESIAN_POINT ( 'NONE',  ( 0.000000000000000000, -32.54542015209054995, -36.68877005347592757 ) ) ;
#1863=DIRECTION ( 'NONE',  ( 1.000000000000000000, 0.000000000000000000, 0.000000000000000000 ) ) ;
#1873=EDGE_CURVE ( 'NONE', #8552, #23988, #13891, .T. ) ;
#1876=VERTEX_POINT ( 'NONE', #33680 ) ;
#1880=ORIENTED_EDGE ( 'NONE', *, *, #20443, .F. ) ;
#1881=EDGE_CURVE ( 'NONE', #1134, #13484, #14128, .T. ) ;
#1883=PLANE ( 'NONE',  #374 ) ;
#1886=EDGE_CURVE ( 'NONE', #29036, #3883, #21854, .T. ) ;
#1890=VERTEX_POINT ( 'NONE', #28998 ) ;
#1895=ORIENTED_EDGE ( 'NONE', *, *, #26937, .F. ) ;
#1896=PLANE ( 'NONE',  #808 ) ;
#1904=ORIENTED_EDGE ( 'NONE', *, *, #11177, .F. ) ;
#1910=CARTESIAN_POINT ( 'NONE',  ( -33.45384370633241389, -29.82153911781839994, 31.38501356826949618 ) ) ;
#1918=AXIS2_PLACEMENT_3D ( 'NONE', #33594, #9217, #16543 ) ;
#1920=ORIENTED_EDGE ( 'NONE', *, *, #7383, .F. ) ;
#1925=VECTOR ( 'NONE', #4663, 1000.000000000000000 ) ;
#1926=EDGE_CURVE ( 'NONE', #22879, #32966, #31662, .T. ) ;
#1937=VERTEX_POINT ( 'NONE', #8953 ) ;
#1940=CIRCLE ( 'NONE', #9901, 32.54542015209057126 ) ;
#1945=LINE ( 'NONE', #6931, #34649 ) ;
#1954=ORIENTED_EDGE ( 'NONE', *, *, #14723, .F. ) ;
#1955=VECTOR ( 'NONE', #34547, 1000.000000000000000 ) ;
#1961=LINE ( 'NONE', #18878, #10317 ) ;
#1968=DIRECTION ( 'NONE',  ( -1.000000000000000000, 0.000000000000000000, 0.000000000000000000 ) ) ;
#1969=FACE_OUTER_BOUND ( 'NONE', #30427, .T. ) ;
#1971=ADVANCED_FACE ( 'NONE', ( #30496 ), #4424, .T. ) ;
#1972=EDGE_CURVE ( 'NONE', #7819, #30998, #34340, .T. ) ;
#1973=DIRECTION ( 'NONE',  ( -0.1081190184239419622, 0.9941379571543595972, 0.000000000000000000 ) ) ;
#1976=DIRECTION ( 'NONE',  ( -0.9635499925192230197, 0.2675283385292205329, 0.000000000000000000 ) ) ;
#1978=ORIENTED_EDGE ( 'NONE', *, *, #20074, .T. ) ;
#1987=ORIENTED_EDGE ( 'NONE', *, *, #29412, .T. ) ;
#1993=AXIS2_PLACEMENT_3D ( 'NONE', #12689, #29576, #10002 ) ;
#1994=ORIENTED_EDGE ( 'NONE', *, *, #19502, .T. ) ;
#1995=DIRECTION ( 'NONE',  ( 0.3193015301359802827, 0.9476531711828023452, 0.000000000000000000 ) ) ;
#1998=ORIENTED_EDGE ( 'NONE', *, *, #14607, .F. ) ;
#2002=CARTESIAN_POINT ( 'NONE',  ( -5.491809612354312087, 32.07872192057775607, -36.68877005347593467 ) ) ;
#2004=CARTESIAN_POINT ( 'NONE',  ( -8.267476927982274404, 31.47782073335738673, 68.31122994652405112 ) ) ;
#2005=ORIENTED_EDGE ( 'NONE', *, *, #446, .F. ) ;
#2007=CARTESIAN_POINT ( 'NONE',  ( -35.71762877834949990, -12.58147180936567011, 68.31122994652405112 ) ) ;
#2008=VECTOR ( 'NONE', #30745, 1000.000000000000227 ) ;
#2009=ORIENTED_EDGE ( 'NONE', *, *, #7383, .T. ) ;
#2011=AXIS2_PLACEMENT_3D ( 'NONE', #23063, #33908, #20391 ) ;
#2016=CARTESIAN_POINT ( 'NONE',  ( 22.89764159710613001, 4.274639749586560455, -77.50000000000000000 ) ) ;
#2019=LINE ( 'NONE', #26054, #20664 ) ;
#2022=PLANE ( 'NONE',  #23453 ) ;
#2023=CARTESIAN_POINT ( 'NONE',  ( -35.00000000000000000, 11.30824010203865271, -28.57494248152495331 ) ) ;
#2027=EDGE_CURVE ( 'NONE', #17138, #4598, #10484, .T. ) ;
#2035=AXIS2_PLACEMENT_3D ( 'NONE', #23508, #6950, #9472 ) ;
#2039=EDGE_CURVE ( 'NONE', #17702, #15632, #27034, .T. ) ;
#2044=DIRECTION ( 'NONE',  ( -0.000000000000000000, 1.836970198721029688E-16, -1.000000000000000000 ) ) ;
#2046=DIRECTION ( 'NONE',  ( 0.000000000000000000, 0.000000000000000000, 1.000000000000000000 ) ) ;
#2051=EDGE_LOOP ( 'NONE', ( #4526, #33909, #32838, #13816 ) ) ;
#2071=VERTEX_POINT ( 'NONE', #2465 ) ;
#2078=AXIS2_PLACEMENT_3D ( 'NONE', #14512, #5581, #19673 ) ;
#2086=VERTEX_POINT ( 'NONE', #10135 ) ;
#2089=EDGE_CURVE ( 'NONE', #20006, #22497, #10840, .T. ) ;
#2093=CARTESIAN_POINT ( 'NONE',  ( -23.46927268871045058, -22.54767421130284077, 68.31122994652405112 ) ) ;
#2096=FACE_OUTER_BOUND ( 'NONE', #14350, .T. ) ;
#2097=VERTEX_POINT ( 'NONE', #21686 ) ;
#2099=AXIS2_PLACEMENT_3D ( 'NONE', #20150, #16970, #22465 ) ;
#2100=DIRECTION ( 'NONE',  ( 1.000000000000000000, 0.000000000000000000, -0.000000000000000000 ) ) ;
#2102=DIRECTION ( 'NONE',  ( 0.4198891015602645438, -0.9075754196709570065, -0.000000000000000000 ) ) ;
#2109=CARTESIAN_POINT ( 'NONE',  ( 0.000000000000000000, 33.69708579775584667, -49.43553178847298568 ) ) ;
#2113=CARTESIAN_POINT ( 'NONE',  ( 0.000000000000000000, 2.515464910414410839E-14, -49.43553178847298568 ) ) ;
#2114=ORIENTED_EDGE ( 'NONE', *, *, #34192, .F. ) ;
#2115=VERTEX_POINT ( 'NONE', #26503 ) ;
#2118=FACE_OUTER_BOUND ( 'NONE', #32218, .T. ) ;
#2119=DIRECTION ( 'NONE',  ( -0.000000000000000000, -0.000000000000000000, -1.000000000000000000 ) ) ;
#2129=DIRECTION ( 'NONE',  ( 0.000000000000000000, 1.836970198721029441E-16, -1.000000000000000000 ) ) ;
#2130=CARTESIAN_POINT ( 'NONE',  ( -20.02113311122498729, -1.691831803474591833, -67.50000000000000000 ) ) ;
#2137=DIRECTION ( 'NONE',  ( -0.000000000000000000, -0.000000000000000000, 1.000000000000000000 ) ) ;
#2143=DIRECTION ( 'NONE',  ( 0.000000000000000000, 1.000000000000000000, 0.000000000000000000 ) ) ;
#2149=VECTOR ( 'NONE', #5904, 1000.000000000000000 ) ;
#2153=LINE ( 'NONE', #34370, #8765 ) ;
#2157=ORIENTED_EDGE ( 'NONE', *, *, #1003, .F. ) ;
#2170=LINE ( 'NONE', #17866, #19258 ) ;
#2175=ADVANCED_FACE ( 'NONE', ( #27731 ), #30407, .F. ) ;
#2186=AXIS2_PLACEMENT_3D ( 'NONE', #8358, #32550, #24193 ) ;
#2190=AXIS2_PLACEMENT_3D ( 'NONE', #27959, #9270, #6407 ) ;
#2200=DIRECTION ( 'NONE',  ( 0.000000000000000000, 0.000000000000000000, 1.000000000000000000 ) ) ;
#2202=EDGE_CURVE ( 'NONE', #9416, #13484, #32718, .T. ) ;
#2206=VERTEX_POINT ( 'NONE', #27554 ) ;
#2211=CIRCLE ( 'NONE', #17010, 32.54542015209056416 ) ;
#2222=CIRCLE ( 'NONE', #19876, 32.54542015209055705 ) ;
#2224=LINE ( 'NONE', #23927, #4468 ) ;
#2236=CARTESIAN_POINT ( 'NONE',  ( 23.31255882915079880, -22.70966696615090896, 68.31122994652405112 ) ) ;
#2237=DIRECTION ( 'NONE',  ( -0.000000000000000000, 1.836970198721029688E-16, -1.000000000000000000 ) ) ;
#2238=EDGE_CURVE ( 'NONE', #19731, #10008, #8685, .T. ) ;
#2242=DIRECTION ( 'NONE',  ( 0.000000000000000000, 0.000000000000000000, -1.000000000000000000 ) ) ;
#2244=EDGE_LOOP ( 'NONE', ( #4738, #4058, #9492, #10473 ) ) ;
#2247=DIRECTION ( 'NONE',  ( 0.000000000000000000, 0.000000000000000000, 1.000000000000000000 ) ) ;
#2250=AXIS2_PLACEMENT_3D ( 'NONE', #28082, #22575, #33416 ) ;
#2260=CARTESIAN_POINT ( 'NONE',  ( -35.00000000000000000, 11.30824010203864205, 68.31122994652405112 ) ) ;
#2263=LINE ( 'NONE', #10985, #15880 ) ;
#2268=ORIENTED_EDGE ( 'NONE', *, *, #1972, .T. ) ;
#2277=CARTESIAN_POINT ( 'NONE',  ( -5.021133111225092982, -11.61907005722761532, -67.50000000000000000 ) ) ;
#2278=LINE ( 'NONE', #2978, #14533 ) ;
#2284=ORIENTED_EDGE ( 'NONE', *, *, #8508, .F. ) ;
#2293=DIRECTION ( 'NONE',  ( 0.8568571761675893850, 0.5155538571770216238, 9.470570714698666623E-17 ) ) ;
#2296=ORIENTED_EDGE ( 'NONE', *, *, #9919, .T. ) ;
#2298=ORIENTED_EDGE ( 'NONE', *, *, #7538, .F. ) ;
#2303=AXIS2_PLACEMENT_3D ( 'NONE', #214, #8563, #11077 ) ;
#2307=DIRECTION ( 'NONE',  ( 3.697785493223492838E-32, 1.934419779023891545E-16, -1.000000000000000000 ) ) ;
#2309=EDGE_CURVE ( 'NONE', #10302, #15568, #13862, .T. ) ;
#2317=ADVANCED_FACE ( 'NONE', ( #3517 ), #25228, .T. ) ;
#2321=EDGE_CURVE ( 'NONE', #29803, #12309, #28615, .T. ) ;
#2324=VERTEX_POINT ( 'NONE', #31282 ) ;
#2334=LINE ( 'NONE', #29039, #5391 ) ;
#2335=DIRECTION ( 'NONE',  ( -0.000000000000000000, 1.836970198721029934E-16, -1.000000000000000000 ) ) ;
#2342=DIRECTION ( 'NONE',  ( 1.000000000000000000, 0.000000000000000000, 0.000000000000000000 ) ) ;
#2343=LINE ( 'NONE', #9837, #2794 ) ;
#2348=PLANE ( 'NONE',  #23173 ) ;
#2355=FACE_OUTER_BOUND ( 'NONE', #25633, .T. ) ;
#2357=AXIS2_PLACEMENT_3D ( 'NONE', #5981, #25023, #662 ) ;
#2371=AXIS2_PLACEMENT_3D ( 'NONE', #4558, #7413, #5096 ) ;
#2375=ORIENTED_EDGE ( 'NONE', *, *, #7992, .T. ) ;
#2384=AXIS2_PLACEMENT_3D ( 'NONE', #23820, #10289, #31645 ) ;
#2385=CARTESIAN_POINT ( 'NONE',  ( 29.63313772848250238, -13.45665341906703816, 68.31122994652405112 ) ) ;
#2396=ADVANCED_FACE ( 'NONE', ( #9578 ), #23281, .F. ) ;
#2401=ORIENTED_EDGE ( 'NONE', *, *, #25438, .T. ) ;
#2404=CLOSED_SHELL ( 'NONE', ( #25394, #6924, #14172, #22095, #26228, #1731, #26540, #35035, #16608, #25299, #15205, #28724, #4289, #27001, #15151, #12148, #4929, #13693, #19058, #9481, #69, #34512, #16321, #14599, #31413, #11999, #19753, #32002, #23004, #15411, #3055, #26923, #26580, #33122, #3737, #31038, #1597, #10619, #18090, #8504, #33967, #11825, #8830, #26343, #22220, #9244, #16707, #31653, #1327, #17147, #8281, #18299, #5634, #5038, #29346, #14743, #34920, #10964, #3643, #1559, #24262, #7948, #25910, #11961, #11353, #9081, #14970, #8783, #19657, #12688, #19176, #33886, #1753, #9168, #6251, #2396, #25890, #11558, #9926, #19309, #2175, #27307, #32739, #23784, #11667, #3280, #22028, #8960, #25190, #25750, #3283, #1063, #30967, #1075, #27714, #11131, #19733, #7599, #18549, #8235, #523, #22645, #16829, #11553, #28897, #4609, #26023, #13580, #30168, #30537, #8458, #7412, #28021, #24, #27454, #31101, #6903, #17190, #26176, #8507, #14921, #12349, #17341, #4362, #25437, #20901, #18359, #24684, #15878, #26423, #5232, #4276, #17015, #22345, #3765, #11585, #23068, #30736, #28292, #33036, #4332, #10171, #18311, #12474, #34073, #16706, #12234, #11446, #1500, #28458, #8074, #3417, #28373, #11709, #20681, #24566, #24063, #33436, #31962, #30889, #2731, #28259, #34780, #29251, #8678, #16855, #32424, #1971, #16854, #33835, #11663, #24099, #14656, #23861, #489, #8182, #23741, #5633, #33094, #11877, #23059, #7790, #1561, #28167, #13438, #2317, #15700, #14265, #10614, #33470, #21911, #22302, #17644, #18518, #13423, #22863, #25679, #6470, #4395, #5168, #7610, #29450, #26872, #29566, #17474, #28960, #32016, #22344, #27871, #20196, #21145, #30311, #29891, #28410, #22616, #611, #6254, #22651, #9199, #21506, #32209, #6368, #33953, #5418, #9286, #29538, #18206, #19793, #9041, #4879, #19196, #1791, #28531, #33477, #15175 ) ) ;
#2407=LINE ( 'NONE', #15607, #27062 ) ;
#2412=EDGE_CURVE ( 'NONE', #6259, #3630, #12436, .T. ) ;
#2415=PLANE ( 'NONE',  #26807 ) ;
#2425=VERTEX_POINT ( 'NONE', #7061 ) ;
#2432=EDGE_CURVE ( 'NONE', #21158, #16944, #20268, .T. ) ;
#2434=FACE_OUTER_BOUND ( 'NONE', #31762, .T. ) ;
#2437=VECTOR ( 'NONE', #14111, 1000.000000000000114 ) ;
#2449=VECTOR ( 'NONE', #29989, 1000.000000000000000 ) ;
#2452=DIRECTION ( 'NONE',  ( -1.000000000000000000, 6.792721752314501023E-48, -3.697785493223492838E-32 ) ) ;
#2453=LINE ( 'NONE', #32185, #1825 ) ;
#2459=VECTOR ( 'NONE', #23170, 1000.000000000000114 ) ;
#2465=CARTESIAN_POINT ( 'NONE',  ( 60.00000000000000000, 33.69708579775584667, 49.43553178847298568 ) ) ;
#2469=LINE ( 'NONE', #33603, #10130 ) ;
#2474=CARTESIAN_POINT ( 'NONE',  ( 0.000000000000000000, 33.69708579775584667, -36.68877005347592757 ) ) ;
#2478=CARTESIAN_POINT ( 'NONE',  ( 17.27856612038524631, 33.69708579775584667, 68.31122994652405112 ) ) ;
#2479=EDGE_LOOP ( 'NONE', ( #29551, #31827, #32049, #16985 ) ) ;
#2486=VECTOR ( 'NONE', #4152, 1000.000000000000000 ) ;
#2493=FACE_OUTER_BOUND ( 'NONE', #4348, .T. ) ;
#2494=CARTESIAN_POINT ( 'NONE',  ( 22.89764159710613001, 4.274639749586560455, -77.50000000000000000 ) ) ;
#2498=CARTESIAN_POINT ( 'NONE',  ( 22.89764159710615132, -3.615060903476078114, -87.50000000000000000 ) ) ;
#2501=ORIENTED_EDGE ( 'NONE', *, *, #18732, .T. ) ;
#2503=ORIENTED_EDGE ( 'NONE', *, *, #2089, .F. ) ;
#2508=ORIENTED_EDGE ( 'NONE', *, *, #18257, .T. ) ;
#2511=AXIS2_PLACEMENT_3D ( 'NONE', #13425, #16104, #24258 ) ;
#2516=ORIENTED_EDGE ( 'NONE', *, *, #361, .T. ) ;
#2523=FACE_OUTER_BOUND ( 'NONE', #18954, .T. ) ;
#2524=VERTEX_POINT ( 'NONE', #13643 ) ;
#2525=DIRECTION ( 'NONE',  ( 0.9075754196709571175, 0.4198891015602645438, 7.713237663339539704E-17 ) ) ;
#2526=FACE_OUTER_BOUND ( 'NONE', #25809, .T. ) ;
#2530=PLANE ( 'NONE',  #32804 ) ;
#2532=EDGE_CURVE ( 'NONE', #9716, #34419, #22007, .T. ) ;
#2548=VECTOR ( 'NONE', #21211, 1000.000000000000000 ) ;
#2550=DIRECTION ( 'NONE',  ( 0.6876994588534233177, -0.7259954919231308423, 0.000000000000000000 ) ) ;
#2554=DIRECTION ( 'NONE',  ( 0.3701381553399133995, -0.9289767198167917517, -0.000000000000000000 ) ) ;
#2556=ORIENTED_EDGE ( 'NONE', *, *, #6456, .T. ) ;
#2564=DIRECTION ( 'NONE',  ( -1.000000000000000000, 6.792721752314501023E-48, -3.697785493223492838E-32 ) ) ;
#2568=EDGE_CURVE ( 'NONE', #14276, #22576, #24657, .T. ) ;
#2573=CARTESIAN_POINT ( 'NONE',  ( 0.000000000000000000, 0.000000000000000000, 87.50000000000000000 ) ) ;
#2575=DIRECTION ( 'NONE',  ( 1.000000000000000000, 0.000000000000000000, 0.000000000000000000 ) ) ;
#2576=ORIENTED_EDGE ( 'NONE', *, *, #9965, .F. ) ;
#2582=LINE ( 'NONE', #30161, #11766 ) ;
#2584=CARTESIAN_POINT ( 'NONE',  ( -45.00000000000000000, 3.353962854566122864, 15.81122994652406355 ) ) ;
#2594=DIRECTION ( 'NONE',  ( 0.000000000000000000, 1.836970198721029688E-16, -1.000000000000000000 ) ) ;
#2596=ORIENTED_EDGE ( 'NONE', *, *, #4717, .F. ) ;
#2599=VECTOR ( 'NONE', #29093, 1000.000000000000000 ) ;
#2603=EDGE_LOOP ( 'NONE', ( #8262, #17852, #24670, #10697 ) ) ;
#2605=CARTESIAN_POINT ( 'NONE',  ( 0.000000000000000000, -33.69708579775584667, -49.43553178847298568 ) ) ;
#2614=CARTESIAN_POINT ( 'NONE',  ( 0.000000000000000000, 2.296212748401288367E-15, 87.50000000000000000 ) ) ;
#2616=ORIENTED_EDGE ( 'NONE', *, *, #26320, .T. ) ;
#2618=PLANE ( 'NONE',  #35048 ) ;
#2619=CARTESIAN_POINT ( 'NONE',  ( -2.216215597024040029, -32.46987467335853239, 68.31122994652405112 ) ) ;
#2622=ORIENTED_EDGE ( 'NONE', *, *, #22348, .T. ) ;
#2636=EDGE_CURVE ( 'NONE', #25782, #11484, #3306, .T. ) ;
#2637=EDGE_CURVE ( 'NONE', #25524, #21875, #5442, .T. ) ;
#2643=CARTESIAN_POINT ( 'NONE',  ( -35.00000000000000000, 42.49491490430484220, -36.69637551990492597 ) ) ;
#2651=EDGE_CURVE ( 'NONE', #33917, #12803, #19177, .T. ) ;
#2654=AXIS2_PLACEMENT_3D ( 'NONE', #18704, #29372, #15864 ) ;
#2655=LINE ( 'NONE', #11023, #8782 ) ;
#2656=DIRECTION ( 'NONE',  ( 0.000000000000000000, 1.000000000000000000, 0.000000000000000000 ) ) ;
#2658=ORIENTED_EDGE ( 'NONE', *, *, #679, .T. ) ;
#2661=CARTESIAN_POINT ( 'NONE',  ( -45.00000000000000000, 16.36947364650383818, -36.69637551990492597 ) ) ;
#2664=ORIENTED_EDGE ( 'NONE', *, *, #23750, .F. ) ;
#2670=LINE ( 'NONE', #21375, #25694 ) ;
#2672=DIRECTION ( 'NONE',  ( 0.5611870653623813876, -0.8276889981568911203, -0.000000000000000000 ) ) ;
#2675=CARTESIAN_POINT ( 'NONE',  ( -31.68358972719163091, 7.440061483287530919, 68.31122994652405112 ) ) ;
#2682=ORIENTED_EDGE ( 'NONE', *, *, #30425, .F. ) ;
#2687=AXIS2_PLACEMENT_3D ( 'NONE', #122, #4917, #15984 ) ;
#2693=CARTESIAN_POINT ( 'NONE',  ( -21.67835495107042476, 31.04982069277122747, 68.31122994652405112 ) ) ;
#2708=DIRECTION ( 'NONE',  ( 1.000000000000000000, 0.000000000000000000, 0.000000000000000000 ) ) ;
#2709=PLANE ( 'NONE',  #189 ) ;
#2714=EDGE_LOOP ( 'NONE', ( #10883, #4586, #4670, #12603, #27163 ) ) ;
#2724=ORIENTED_EDGE ( 'NONE', *, *, #15400, .T. ) ;
#2725=CIRCLE ( 'NONE', #6149, 2.033421858999711951 ) ;
#2727=DIRECTION ( 'NONE',  ( -0.7259954919231308423, -0.6876994588534233177, -1.263283411590317421E-16 ) ) ;
#2730=DIRECTION ( 'NONE',  ( -1.000000000000000000, 0.000000000000000000, 0.000000000000000000 ) ) ;
#2731=ADVANCED_FACE ( 'NONE', ( #23240 ), #9176, .T. ) ;
#2749=CYLINDRICAL_SURFACE ( 'NONE', #3235, 32.54542015209057126 ) ;
#2751=VERTEX_POINT ( 'NONE', #3824 ) ;
#2754=VERTEX_POINT ( 'NONE', #33915 ) ;
#2760=CARTESIAN_POINT ( 'NONE',  ( -5.491809612354312087, 32.07872192057773475, 68.31122994652405112 ) ) ;
#2764=VERTEX_POINT ( 'NONE', #1523 ) ;
#2769=CARTESIAN_POINT ( 'NONE',  ( 3.235562306570555532E-30, 4.168562732279004202, -67.50000000000000000 ) ) ;
#2775=CARTESIAN_POINT ( 'NONE',  ( 23.31255882915078814, -22.70966696615089830, 49.43553178847298568 ) ) ;
#2779=ORIENTED_EDGE ( 'NONE', *, *, #29449, .F. ) ;
#2791=CARTESIAN_POINT ( 'NONE',  ( -10.84269519964070305, -36.27449394610879096, 68.31122994652405112 ) ) ;
#2794=VECTOR ( 'NONE', #13223, 1000.000000000000114 ) ;
#2805=CIRCLE ( 'NONE', #27250, 2.033421858999711951 ) ;
#2812=CARTESIAN_POINT ( 'NONE',  ( 30.98406361983693103, 9.959526819984924728, 49.43553178847298568 ) ) ;
#2814=AXIS2_PLACEMENT_3D ( 'NONE', #29009, #29375, #7461 ) ;
#2823=EDGE_CURVE ( 'NONE', #25524, #24033, #15234, .T. ) ;
#2826=ORIENTED_EDGE ( 'NONE', *, *, #29090, .T. ) ;
#2830=EDGE_CURVE ( 'NONE', #11221, #1041, #7904, .T. ) ;
#2835=VERTEX_POINT ( 'NONE', #31752 ) ;
#2838=CARTESIAN_POINT ( 'NONE',  ( 1.532562817202168137, 32.50931595846690669, 68.31122994652405112 ) ) ;
#2841=FACE_OUTER_BOUND ( 'NONE', #22149, .T. ) ;
#2850=DIRECTION ( 'NONE',  ( 0.000000000000000000, 1.000000000000000000, 0.000000000000000000 ) ) ;
#2856=VERTEX_POINT ( 'NONE', #10224 ) ;
#2858=LINE ( 'NONE', #11241, #10205 ) ;
#2863=VERTEX_POINT ( 'NONE', #9874 ) ;
#2864=CARTESIAN_POINT ( 'NONE',  ( -5.491809612354312975, 32.07872192057773475, 68.31122994652405112 ) ) ;
#2866=DIRECTION ( 'NONE',  ( -0.000000000000000000, 1.836970198721029934E-16, -1.000000000000000000 ) ) ;
#2867=CARTESIAN_POINT ( 'NONE',  ( 10.96230482721425403, -12.47301499840864025, -77.50000000000000000 ) ) ;
#2872=CARTESIAN_POINT ( 'NONE',  ( 30.98406361983693103, 9.959526819984924728, 49.43553178847298568 ) ) ;
#2873=EDGE_CURVE ( 'NONE', #18186, #23654, #34258, .T. ) ;
#2875=VECTOR ( 'NONE', #24618, 1000.000000000000000 ) ;
#2880=DIRECTION ( 'NONE',  ( 0.000000000000000000, 1.836970198721029934E-16, -1.000000000000000000 ) ) ;
#2888=VECTOR ( 'NONE', #6809, 1000.000000000000227 ) ;
#2890=VECTOR ( 'NONE', #1110, 1000.000000000000000 ) ;
#2892=ORIENTED_EDGE ( 'NONE', *, *, #25388, .T. ) ;
#2900=AXIS2_PLACEMENT_3D ( 'NONE', #28578, #15236, #29087 ) ;
#2901=CARTESIAN_POINT ( 'NONE',  ( 8.927936315454010341, -31.29690601358701940, 68.31122994652405112 ) ) ;
#2905=DIRECTION ( 'NONE',  ( -0.9868265225415261410, 0.1617819965527647341, -0.000000000000000000 ) ) ;
#2908=PLANE ( 'NONE',  #26679 ) ;
#2910=ORIENTED_EDGE ( 'NONE', *, *, #16125, .F. ) ;
#2918=VECTOR ( 'NONE', #10255, 1000.000000000000114 ) ;
#2919=EDGE_CURVE ( 'NONE', #2856, #3550, #16287, .T. ) ;
#2920=CARTESIAN_POINT ( 'NONE',  ( 31.73435513276359643, 7.220462394039754095, 49.43553178847298568 ) ) ;
#2922=CARTESIAN_POINT ( 'NONE',  ( -35.00000000000000000, 42.49491490430484220, 36.69637551990492597 ) ) ;
#2924=VERTEX_POINT ( 'NONE', #1857 ) ;
#2926=ORIENTED_EDGE ( 'NONE', *, *, #34135, .F. ) ;
#2927=CARTESIAN_POINT ( 'NONE',  ( 0.000000000000000000, -32.54542015209051442, -87.50000000000000000 ) ) ;
#2934=DIRECTION ( 'NONE',  ( -0.000000000000000000, 1.000000000000000000, -0.000000000000000000 ) ) ;
#2948=DIRECTION ( 'NONE',  ( 0.000000000000000000, -1.000000000000000000, 0.000000000000000000 ) ) ;
#2949=ORIENTED_EDGE ( 'NONE', *, *, #10436, .T. ) ;
#2951=EDGE_CURVE ( 'NONE', #28825, #11793, #26768, .T. ) ;
#2953=DIRECTION ( 'NONE',  ( -0.000000000000000000, -0.000000000000000000, -1.000000000000000000 ) ) ;
#2954=CARTESIAN_POINT ( 'NONE',  ( 6.857172176539690689, 37.23415287044793587, 68.31122994652405112 ) ) ;
#2958=DIRECTION ( 'NONE',  ( 0.000000000000000000, 1.836970198721029441E-16, -1.000000000000000000 ) ) ;
#2959=CARTESIAN_POINT ( 'NONE',  ( -2.791255079241054649, -37.75727539589166071, 68.31122994652405112 ) ) ;
#2961=EDGE_CURVE ( 'NONE', #22052, #26665, #20817, .T. ) ;
#2962=CARTESIAN_POINT ( 'NONE',  ( -9.978866888775527855, 4.168562732279005090, -67.50000000000000000 ) ) ;
#2971=VERTEX_POINT ( 'NONE', #11456 ) ;
#2976=ORIENTED_EDGE ( 'NONE', *, *, #34307, .T. ) ;
#2978=CARTESIAN_POINT ( 'NONE',  ( 23.93847777447631131, 22.04889236939138186, 68.31122994652405112 ) ) ;
#2994=ORIENTED_EDGE ( 'NONE', *, *, #20017, .F. ) ;
#2995=CARTESIAN_POINT ( 'NONE',  ( -18.38714294329533416, -33.09555747561021377, 68.31122994652405112 ) ) ;
#2998=ORIENTED_EDGE ( 'NONE', *, *, #22626, .F. ) ;
#2999=VERTEX_POINT ( 'NONE', #8075 ) ;
#3002=DIRECTION ( 'NONE',  ( 0.000000000000000000, -0.5288966977476834419, -0.8486862100397269959 ) ) ;
#3006=ORIENTED_EDGE ( 'NONE', *, *, #30583, .F. ) ;
#3011=CARTESIAN_POINT ( 'NONE',  ( 14.70109753509668948, 34.88954974633765005, 68.31122994652405112 ) ) ;
#3029=VERTEX_POINT ( 'NONE', #5215 ) ;
#3030=EDGE_CURVE ( 'NONE', #18432, #23654, #16637, .T. ) ;
#3036=CARTESIAN_POINT ( 'NONE',  ( -9.978866888775426602, 18.16264470403145381, -87.50000000000000000 ) ) ;
#3046=CARTESIAN_POINT ( 'NONE',  ( 3.235562306570555532E-30, -11.61907005722761177, -87.50000000000000000 ) ) ;
#3047=PLANE ( 'NONE',  #8427 ) ;
#3048=CARTESIAN_POINT ( 'NONE',  ( 0.000000000000000000, 2.281310696040539424E-14, -36.68877005347592757 ) ) ;
#3050=DIRECTION ( 'NONE',  ( 3.697785493223492838E-32, 1.934419779023891545E-16, -1.000000000000000000 ) ) ;
#3051=ORIENTED_EDGE ( 'NONE', *, *, #31324, .T. ) ;
#3052=LINE ( 'NONE', #16966, #8400 ) ;
#3053=CARTESIAN_POINT ( 'NONE',  ( -1.307386931792819285, 37.83772838912469894, 68.31122994652405112 ) ) ;
#3055=ADVANCED_FACE ( 'NONE', ( #27118 ), #24654, .F. ) ;
#3062=VECTOR ( 'NONE', #25003, 1000.000000000000114 ) ;
#3066=DIRECTION ( 'NONE',  ( 0.000000000000000000, 0.000000000000000000, 1.000000000000000000 ) ) ;
#3073=EDGE_CURVE ( 'NONE', #16921, #18651, #10761, .T. ) ;
#3078=VERTEX_POINT ( 'NONE', #2901 ) ;
#3085=ORIENTED_EDGE ( 'NONE', *, *, #6533, .T. ) ;
#3087=LINE ( 'NONE', #22682, #24196 ) ;
#3088=EDGE_CURVE ( 'NONE', #21431, #20048, #33512, .T. ) ;
#3089=DIRECTION ( 'NONE',  ( 0.000000000000000000, 1.000000000000000000, 1.836970198721029688E-16 ) ) ;
#3102=DIRECTION ( 'NONE',  ( 0.000000000000000000, -1.000000000000000000, 0.000000000000000000 ) ) ;
#3113=FACE_OUTER_BOUND ( 'NONE', #16213, .T. ) ;
#3114=VECTOR ( 'NONE', #34487, 1000.000000000000000 ) ;
#3116=ORIENTED_EDGE ( 'NONE', *, *, #9237, .F. ) ;
#3122=DIRECTION ( 'NONE',  ( 0.000000000000000000, 1.836970198721029688E-16, -1.000000000000000000 ) ) ;
#3126=CARTESIAN_POINT ( 'NONE',  ( 26.04754872656010889, -19.51229300245305964, 68.31122994652405112 ) ) ;
#3130=CARTESIAN_POINT ( 'NONE',  ( -20.02113311122488781, 4.168562732279004202, -67.50000000000000000 ) ) ;
#3131=ORIENTED_EDGE ( 'NONE', *, *, #28641, .F. ) ;
#3139=PLANE ( 'NONE',  #17507 ) ;
#3144=DIRECTION ( 'NONE',  ( 0.000000000000000000, 1.836970198721029441E-16, -1.000000000000000000 ) ) ;
#3146=DIRECTION ( 'NONE',  ( 0.000000000000000000, 1.836970198721029441E-16, -1.000000000000000000 ) ) ;
#3157=CARTESIAN_POINT ( 'NONE',  ( 18.19419936998243870, -33.21164777187627237, 68.31122994652405112 ) ) ;
#3158=CARTESIAN_POINT ( 'NONE',  ( -9.410814080250917257, 36.67205378194064735, 68.31122994652405112 ) ) ;
#3161=AXIS2_PLACEMENT_3D ( 'NONE', #30807, #3907, #14799 ) ;
#3162=EDGE_CURVE ( 'NONE', #11635, #11447, #12343, .T. ) ;
#3168=CARTESIAN_POINT ( 'NONE',  ( 0.000000000000000000, 3.524919873834583163E-15, 68.31122994652405112 ) ) ;
#3169=LINE ( 'NONE', #19382, #26083 ) ;
#3176=CARTESIAN_POINT ( 'NONE',  ( 26.97014235612466493, -26.57093094961043889, 68.31122994652405112 ) ) ;
#3179=PLANE ( 'NONE',  #9751 ) ;
#3182=AXIS2_PLACEMENT_3D ( 'NONE', #21257, #29272, #29085 ) ;
#3185=ORIENTED_EDGE ( 'NONE', *, *, #4085, .T. ) ;
#3193=VECTOR ( 'NONE', #12968, 1000.000000000000000 ) ;
#3203=ORIENTED_EDGE ( 'NONE', *, *, #26828, .T. ) ;
#3205=EDGE_CURVE ( 'NONE', #3784, #32269, #3859, .T. ) ;
#3209=CARTESIAN_POINT ( 'NONE',  ( -36.04853892210773836, 11.59936550071286376, 68.31122994652405112 ) ) ;
#3210=VECTOR ( 'NONE', #25103, 1000.000000000000000 ) ;
#3225=EDGE_CURVE ( 'NONE', #32722, #29816, #4124, .T. ) ;
#3227=EDGE_LOOP ( 'NONE', ( #10350, #22448, #6055, #15690 ) ) ;
#3228=DIRECTION ( 'NONE',  ( 0.000000000000000000, 1.000000000000000000, 0.000000000000000000 ) ) ;
#3235=AXIS2_PLACEMENT_3D ( 'NONE', #2573, #32990, #3102 ) ;
#3241=VECTOR ( 'NONE', #28099, 1000.000000000000000 ) ;
#3250=EDGE_LOOP ( 'NONE', ( #12103, #32729, #8584, #24155 ) ) ;
#3251=VECTOR ( 'NONE', #10058, 1000.000000000000000 ) ;
#3261=ORIENTED_EDGE ( 'NONE', *, *, #20133, .F. ) ;
#3263=FACE_OUTER_BOUND ( 'NONE', #6795, .T. ) ;
#3268=FACE_OUTER_BOUND ( 'NONE', #26016, .T. ) ;
#3272=AXIS2_PLACEMENT_3D ( 'NONE', #33391, #32855, #16686 ) ;
#3273=CARTESIAN_POINT ( 'NONE',  ( -29.68486519896224962, 23.49918569563710946, 68.31122994652405112 ) ) ;
#3276=DIRECTION ( 'NONE',  ( 0.8568571761675893850, 0.5155538571770214018, -0.000000000000000000 ) ) ;
#3280=ADVANCED_FACE ( 'NONE', ( #23875 ), #18571, .T. ) ;
#3283=ADVANCED_FACE ( 'NONE', ( #26193 ), #15720, .F. ) ;
#3294=CARTESIAN_POINT ( 'NONE',  ( -29.72561944762171393, -13.25111019240557475, -36.68877005347593467 ) ) ;
#3296=ORIENTED_EDGE ( 'NONE', *, *, #5264, .F. ) ;
#3297=VECTOR ( 'NONE', #31084, 1000.000000000000000 ) ;
#3298=ORIENTED_EDGE ( 'NONE', *, *, #31333, .T. ) ;
#3305=CIRCLE ( 'NONE', #9008, 2.036051781435517682 ) ;
#3306=LINE ( 'NONE', #8116, #419 ) ;
#3307=DIRECTION ( 'NONE',  ( 1.000000000000000000, 0.000000000000000000, 0.000000000000000000 ) ) ;
#3309=ORIENTED_EDGE ( 'NONE', *, *, #25659, .F. ) ;
#3313=DIRECTION ( 'NONE',  ( 1.000000000000000000, 0.000000000000000000, 0.000000000000000000 ) ) ;
#3314=CARTESIAN_POINT ( 'NONE',  ( 32.40067729534749219, 3.066020821660472517, 68.31122994652405112 ) ) ;
#3320=ORIENTED_EDGE ( 'NONE', *, *, #3030, .F. ) ;
#3326=ORIENTED_EDGE ( 'NONE', *, *, #21570, .F. ) ;
#3335=CARTESIAN_POINT ( 'NONE',  ( 11.62236370382047745, -30.39942490923500884, 68.31122994652405112 ) ) ;
#3341=ORIENTED_EDGE ( 'NONE', *, *, #14771, .T. ) ;
#3350=ORIENTED_EDGE ( 'NONE', *, *, #9971, .F. ) ;
#3353=DIRECTION ( 'NONE',  ( 0.000000000000000000, 1.000000000000000000, 1.836970198721029688E-16 ) ) ;
#3357=DIRECTION ( 'NONE',  ( 0.000000000000000000, 1.000000000000000000, 0.000000000000000000 ) ) ;
#3362=ORIENTED_EDGE ( 'NONE', *, *, #17017, .F. ) ;
#3365=CARTESIAN_POINT ( 'NONE',  ( 0.000000000000000000, -44.99999999999997868, 87.49999999999998579 ) ) ;
#3369=EDGE_CURVE ( 'NONE', #22969, #31238, #2170, .T. ) ;
#3370=CARTESIAN_POINT ( 'NONE',  ( 0.000000000000000000, 2.281310696040539424E-14, -36.68877005347592757 ) ) ;
#3385=LINE ( 'NONE', #16238, #19929 ) ;
#3396=CARTESIAN_POINT ( 'NONE',  ( 27.64943126350854286, -17.16721653852534146, 68.31122994652405112 ) ) ;
#3398=FACE_OUTER_BOUND ( 'NONE', #19137, .T. ) ;
#3400=ORIENTED_EDGE ( 'NONE', *, *, #10997, .F. ) ;
#3401=LINE ( 'NONE', #16434, #15225 ) ;
#3402=DIRECTION ( 'NONE',  ( 0.000000000000000000, -1.000000000000000000, -1.836970198721029934E-16 ) ) ;
#3404=VERTEX_POINT ( 'NONE', #1815 ) ;
#3406=FACE_OUTER_BOUND ( 'NONE', #2479, .T. ) ;
#3409=CARTESIAN_POINT ( 'NONE',  ( -37.12776225901827587, -7.411627343331159246, 68.31122994652405112 ) ) ;
#3410=LINE ( 'NONE', #5716, #12773 ) ;
#3412=EDGE_CURVE ( 'NONE', #2971, #25849, #34931, .T. ) ;
#3413=CARTESIAN_POINT ( 'NONE',  ( -5.021133111224886036, 6.201984591278717041, -67.50000000000000000 ) ) ;
#3417=ADVANCED_FACE ( 'NONE', ( #1645 ), #23356, .T. ) ;
#3420=ORIENTED_EDGE ( 'NONE', *, *, #4352, .F. ) ;
#3428=CARTESIAN_POINT ( 'NONE',  ( 32.81769769215652133, 18.87860345536237006, 68.31122994652405112 ) ) ;
#3429=LINE ( 'NONE', #27821, #6305 ) ;
#3430=VERTEX_POINT ( 'NONE', #2693 ) ;
#3432=DIRECTION ( 'NONE',  ( 0.5155538571770215128, -0.8568571761675892740, 0.000000000000000000 ) ) ;
#3435=DIRECTION ( 'NONE',  ( 0.9868265225415266961, 0.1617819965527614590, 2.971887063570111902E-17 ) ) ;
#3436=DIRECTION ( 'NONE',  ( 0.000000000000000000, 1.836970198721029934E-16, -1.000000000000000000 ) ) ;
#3437=LINE ( 'NONE', #31041, #31881 ) ;
#3438=ORIENTED_EDGE ( 'NONE', *, *, #28604, .T. ) ;
#3445=DIRECTION ( 'NONE',  ( 0.6473862847818279143, -0.7621620551276363509, -1.400068981865442877E-16 ) ) ;
#3450=EDGE_CURVE ( 'NONE', #1565, #1194, #1607, .T. ) ;
#3455=DIRECTION ( 'NONE',  ( 0.000000000000000000, 1.836970198721029688E-16, -1.000000000000000000 ) ) ;
#3459=LINE ( 'NONE', #33191, #30237 ) ;
#3460=CARTESIAN_POINT ( 'NONE',  ( 0.000000000000000000, 3.524919873834583163E-15, 68.31122994652405112 ) ) ;
#3465=ORIENTED_EDGE ( 'NONE', *, *, #10528, .F. ) ;
#3466=PLANE ( 'NONE',  #28161 ) ;
#3467=ORIENTED_EDGE ( 'NONE', *, *, #9872, .T. ) ;
#3468=VERTEX_POINT ( 'NONE', #10890 ) ;
#3471=EDGE_CURVE ( 'NONE', #17629, #7314, #13735, .T. ) ;
#3472=CARTESIAN_POINT ( 'NONE',  ( -6.637260778198712075, 37.28255902965928215, 68.31122994652405112 ) ) ;
#3476=CARTESIAN_POINT ( 'NONE',  ( 32.40067729534750640, 3.066020821660472961, 68.31122994652405112 ) ) ;
#3478=ORIENTED_EDGE ( 'NONE', *, *, #32543, .F. ) ;
#3479=AXIS2_PLACEMENT_3D ( 'NONE', #31481, #7085, #23468 ) ;
#3483=CIRCLE ( 'NONE', #31905, 32.54542015209057126 ) ;
#3484=LINE ( 'NONE', #14370, #15207 ) ;
#3485=EDGE_CURVE ( 'NONE', #16627, #22969, #8207, .T. ) ;
#3490=VERTEX_POINT ( 'NONE', #14094 ) ;
#3506=AXIS2_PLACEMENT_3D ( 'NONE', #27240, #10710, #21560 ) ;
#3514=AXIS2_PLACEMENT_3D ( 'NONE', #12608, #23450, #15455 ) ;
#3517=FACE_OUTER_BOUND ( 'NONE', #29201, .T. ) ;
#3518=LINE ( 'NONE', #22580, #5134 ) ;
#3521=ORIENTED_EDGE ( 'NONE', *, *, #16292, .F. ) ;
#3529=ORIENTED_EDGE ( 'NONE', *, *, #2873, .T. ) ;
#3530=ORIENTED_EDGE ( 'NONE', *, *, #9151, .T. ) ;
#3535=CARTESIAN_POINT ( 'NONE',  ( 4.815661544189684840, -32.18716788982705168, 68.31122994652405112 ) ) ;
#3540=FACE_OUTER_BOUND ( 'NONE', #25135, .T. ) ;
#3542=LINE ( 'NONE', #20288, #1593 ) ;
#3543=DIRECTION ( 'NONE',  ( -0.000000000000000000, 1.836970198721029934E-16, -1.000000000000000000 ) ) ;
#3549=CARTESIAN_POINT ( 'NONE',  ( 5.021133111224576062, 16.12922284503173742, -67.50000000000000000 ) ) ;
#3550=VERTEX_POINT ( 'NONE', #32241 ) ;
#3555=VERTEX_POINT ( 'NONE', #5173 ) ;
#3556=EDGE_CURVE ( 'NONE', #3555, #32705, #3305, .T. ) ;
#3562=ORIENTED_EDGE ( 'NONE', *, *, #9483, .F. ) ;
#3578=ORIENTED_EDGE ( 'NONE', *, *, #902, .F. ) ;
#3581=CARTESIAN_POINT ( 'NONE',  ( 17.88561705399011714, -27.19023860642122514, 68.31122994652405112 ) ) ;
#3587=ORIENTED_EDGE ( 'NONE', *, *, #22055, .T. ) ;
#3589=CARTESIAN_POINT ( 'NONE',  ( -36.94452915644502866, -7.381587800927575493, 17.40055616961943485 ) ) ;
#3601=EDGE_LOOP ( 'NONE', ( #10568, #22999, #7765, #906 ) ) ;
#3608=ORIENTED_EDGE ( 'NONE', *, *, #33137, .T. ) ;
#3610=CARTESIAN_POINT ( 'NONE',  ( 0.000000000000000000, 6.992329373473909019E-15, 49.43553178847298568 ) ) ;
#3613=DIRECTION ( 'NONE',  ( 0.4198891015602652099, -0.9075754196709567845, 0.000000000000000000 ) ) ;
#3614=CARTESIAN_POINT ( 'NONE',  ( -9.978866888775527855, 4.168562732279004202, -67.50000000000000000 ) ) ;
#3618=AXIS2_PLACEMENT_3D ( 'NONE', #3168, #11544, #30404 ) ;
#3623=CARTESIAN_POINT ( 'NONE',  ( -20.02113311122488781, 6.201984591278717041, -67.50000000000000000 ) ) ;
#3630=VERTEX_POINT ( 'NONE', #22632 ) ;
#3632=DIRECTION ( 'NONE',  ( 0.000000000000000000, 1.836970198721029441E-16, -1.000000000000000000 ) ) ;
#3634=ORIENTED_EDGE ( 'NONE', *, *, #24897, .T. ) ;
#3635=PLANE ( 'NONE',  #13728 ) ;
#3641=ORIENTED_EDGE ( 'NONE', *, *, #1684, .F. ) ;
#3643=ADVANCED_FACE ( 'NONE', ( #28139 ), #17124, .F. ) ;
#3654=EDGE_CURVE ( 'NONE', #34419, #7314, #17489, .T. ) ;
#3655=EDGE_LOOP ( 'NONE', ( #19290, #9366, #26074, #21593 ) ) ;
#3656=AXIS2_PLACEMENT_3D ( 'NONE', #9476, #6248, #33672 ) ;
#3658=CARTESIAN_POINT ( 'NONE',  ( 30.45781707305797070, -22.50252913745434924, 68.31122994652405112 ) ) ;
#3666=LINE ( 'NONE', #11172, #30491 ) ;
#3669=DIRECTION ( 'NONE',  ( -0.9941379571543595972, 0.1081190184239420177, 1.986114147597514287E-17 ) ) ;
#3670=ORIENTED_EDGE ( 'NONE', *, *, #2432, .F. ) ;
#3679=VECTOR ( 'NONE', #10160, 1000.000000000000000 ) ;
#3682=CIRCLE ( 'NONE', #1429, 2.036051781435510577 ) ;
#3683=CARTESIAN_POINT ( 'NONE',  ( -31.68358972719163091, 7.440061483287550459, -36.68877005347593467 ) ) ;
#3685=CARTESIAN_POINT ( 'NONE',  ( 0.000000000000000000, 0.000000000000000000, 87.50000000000000000 ) ) ;
#3691=FACE_OUTER_BOUND ( 'NONE', #5204, .T. ) ;
#3697=ORIENTED_EDGE ( 'NONE', *, *, #19548, .F. ) ;
#3702=CARTESIAN_POINT ( 'NONE',  ( -5.021133111224989953, -1.691831803474588058, -87.50000000000000000 ) ) ;
#3705=LINE ( 'NONE', #7589, #34756 ) ;
#3712=ORIENTED_EDGE ( 'NONE', *, *, #14723, .T. ) ;
#3713=VECTOR ( 'NONE', #34609, 1000.000000000000114 ) ;
#3723=LINE ( 'NONE', #30786, #22860 ) ;
#3724=DIRECTION ( 'NONE',  ( 0.6473862847818285804, -0.7621620551276356847, 0.000000000000000000 ) ) ;
#3733=ORIENTED_EDGE ( 'NONE', *, *, #5463, .T. ) ;
#3737=ADVANCED_FACE ( 'NONE', ( #29368 ), #23669, .F. ) ;
#3745=FACE_OUTER_BOUND ( 'NONE', #3935, .T. ) ;
#3747=CARTESIAN_POINT ( 'NONE',  ( 11.62236370382048101, -30.39942490923501950, 68.31122994652405112 ) ) ;
#3751=DIRECTION ( 'NONE',  ( 0.1081190184239419622, -0.9941379571543595972, 0.000000000000000000 ) ) ;
#3762=CARTESIAN_POINT ( 'NONE',  ( 5.021133111224369117, -5.758675521474015291, -67.50000000000000000 ) ) ;
#3765=ADVANCED_FACE ( 'NONE', ( #26333 ), #7108, .F. ) ;
#3770=LINE ( 'NONE', #17511, #16540 ) ;
#3776=( LENGTH_UNIT ( ) NAMED_UNIT ( * ) SI_UNIT ( .MILLI., .METRE. ) );
#3784=VERTEX_POINT ( 'NONE', #20826 ) ;
#3786=PLANE ( 'NONE',  #22840 ) ;
#3787=ORIENTED_EDGE ( 'NONE', *, *, #4872, .F. ) ;
#3794=ORIENTED_EDGE ( 'NONE', *, *, #4288, .F. ) ;
#3802=DIRECTION ( 'NONE',  ( 1.000000000000000000, -0.000000000000000000, -0.000000000000000000 ) ) ;
#3805=EDGE_CURVE ( 'NONE', #5316, #12202, #4264, .T. ) ;
#3810=CYLINDRICAL_SURFACE ( 'NONE', #22806, 2.033421858999711951 ) ;
#3813=LINE ( 'NONE', #18895, #17158 ) ;
#3820=ORIENTED_EDGE ( 'NONE', *, *, #5576, .T. ) ;
#3822=CIRCLE ( 'NONE', #997, 2.033421858999711951 ) ;
#3823=DIRECTION ( 'NONE',  ( 0.000000000000000000, 1.000000000000000000, 0.000000000000000000 ) ) ;
#3824=CARTESIAN_POINT ( 'NONE',  ( -9.978866888775426602, 14.09580098603202458, -67.50000000000000000 ) ) ;
#3826=ORIENTED_EDGE ( 'NONE', *, *, #121, .F. ) ;
#3828=LINE ( 'NONE', #9878, #4854 ) ;
#3829=FACE_OUTER_BOUND ( 'NONE', #21839, .T. ) ;
#3836=VERTEX_POINT ( 'NONE', #9792 ) ;
#3838=DIRECTION ( 'NONE',  ( -0.7960930657056428661, 0.6051742151937663516, 0.000000000000000000 ) ) ;
#3840=DIRECTION ( 'NONE',  ( 0.000000000000000000, 1.836970198721029441E-16, -1.000000000000000000 ) ) ;
#3843=AXIS2_PLACEMENT_3D ( 'NONE', #15336, #2307, #2143 ) ;
#3845=ORIENTED_EDGE ( 'NONE', *, *, #21690, .F. ) ;
#3846=EDGE_CURVE ( 'NONE', #21178, #21158, #17569, .T. ) ;
#3849=EDGE_CURVE ( 'NONE', #23988, #5983, #18007, .T. ) ;
#3851=ORIENTED_EDGE ( 'NONE', *, *, #16696, .T. ) ;
#3857=EDGE_CURVE ( 'NONE', #10848, #29430, #653, .T. ) ;
#3859=CIRCLE ( 'NONE', #23186, 32.54542015209056416 ) ;
#3861=DIRECTION ( 'NONE',  ( 1.000000000000000000, 0.000000000000000000, 0.000000000000000000 ) ) ;
#3863=DIRECTION ( 'NONE',  ( 0.3701381553399133995, -0.9289767198167917517, -0.000000000000000000 ) ) ;
#3883=VERTEX_POINT ( 'NONE', #27041 ) ;
#3885=AXIS2_PLACEMENT_3D ( 'NONE', #5525, #13565, #24398 ) ;
#3886=CARTESIAN_POINT ( 'NONE',  ( 10.17231796313411429, 15.60017778382161424, -87.50000000000000000 ) ) ;
#3889=DIRECTION ( 'NONE',  ( -0.000000000000000000, -1.836970198721029688E-16, 1.000000000000000000 ) ) ;
#3893=EDGE_CURVE ( 'NONE', #22752, #25215, #8164, .T. ) ;
#3900=VERTEX_POINT ( 'NONE', #10682 ) ;
#3906=ORIENTED_EDGE ( 'NONE', *, *, #9824, .T. ) ;
#3907=DIRECTION ( 'NONE',  ( -0.000000000000000000, -0.000000000000000000, -1.000000000000000000 ) ) ;
#3912=EDGE_CURVE ( 'NONE', #32615, #1165, #9030, .T. ) ;
#3915=ORIENTED_EDGE ( 'NONE', *, *, #22996, .T. ) ;
#3918=EDGE_CURVE ( 'NONE', #23287, #15452, #10847, .T. ) ;
#3920=CYLINDRICAL_SURFACE ( 'NONE', #10879, 2.036051781435508801 ) ;
#3934=CARTESIAN_POINT ( 'NONE',  ( -5.021133111224989953, -5.758675521474012626, -87.50000000000000000 ) ) ;
#3935=EDGE_LOOP ( 'NONE', ( #5498, #20270, #10714, #11543 ) ) ;
#3942=CARTESIAN_POINT ( 'NONE',  ( -32.54223829851967764, 0.4550817492056100644, 68.31122994652405112 ) ) ;
#3945=EDGE_LOOP ( 'NONE', ( #13217, #1920, #12817, #16106 ) ) ;
#3946=EDGE_CURVE ( 'NONE', #14788, #10055, #12454, .T. ) ;
#3957=CARTESIAN_POINT ( 'NONE',  ( -32.37866696771086339, 3.290334066652099043, -36.68877005347593467 ) ) ;
#3960=LINE ( 'NONE', #9502, #32993 ) ;
#3962=ORIENTED_EDGE ( 'NONE', *, *, #25842, .T. ) ;
#3964=LINE ( 'NONE', #6280, #15132 ) ;
#3966=EDGE_LOOP ( 'NONE', ( #9619, #10632, #14603, #27494 ) ) ;
#3971=VECTOR ( 'NONE', #30981, 1000.000000000000000 ) ;
#3973=DIRECTION ( 'NONE',  ( -1.000000000000000000, 0.000000000000000000, 0.000000000000000000 ) ) ;
#3974=FACE_OUTER_BOUND ( 'NONE', #16629, .T. ) ;
#3976=ORIENTED_EDGE ( 'NONE', *, *, #17509, .F. ) ;
#3991=LINE ( 'NONE', #25902, #4493 ) ;
#3992=EDGE_CURVE ( 'NONE', #35091, #6717, #2211, .T. ) ;
#3998=CARTESIAN_POINT ( 'NONE',  ( -5.491809612354312975, 32.07872192057773475, 68.31122994652405112 ) ) ;
#3999=CARTESIAN_POINT ( 'NONE',  ( 30.98406361983693103, 9.959526819984921175, 68.31122994652405112 ) ) ;
#4001=DIRECTION ( 'NONE',  ( 0.000000000000000000, -1.000000000000000000, -1.836970198721029934E-16 ) ) ;
#4009=CARTESIAN_POINT ( 'NONE',  ( -25.07182831876307105, -28.36910952062234870, 68.31122994652405112 ) ) ;
#4012=EDGE_LOOP ( 'NONE', ( #17001, #28215, #12911, #33865 ) ) ;
#4016=DIRECTION ( 'NONE',  ( 0.000000000000000000, -1.000000000000000000, -1.836970198721029688E-16 ) ) ;
#4022=EDGE_LOOP ( 'NONE', ( #17268, #15743, #11741, #8505 ) ) ;
#4025=VECTOR ( 'NONE', #7127, 1000.000000000000000 ) ;
#4042=CARTESIAN_POINT ( 'NONE',  ( 37.71145559917817280, 3.353962854566119756, 68.31122994652405112 ) ) ;
#4045=CARTESIAN_POINT ( 'NONE',  ( 27.99209646187092559, 25.49206711720156093, 68.31122994652405112 ) ) ;
#4053=CARTESIAN_POINT ( 'NONE',  ( -11.83261234297099662, -30.31820670846267873, 68.31122994652405112 ) ) ;
#4058=ORIENTED_EDGE ( 'NONE', *, *, #2636, .F. ) ;
#4064=PLANE ( 'NONE',  #33823 ) ;
#4067=AXIS2_PLACEMENT_3D ( 'NONE', #17048, #33924, #17578 ) ;
#4085=EDGE_CURVE ( 'NONE', #31849, #24798, #25731, .T. ) ;
#4089=DIRECTION ( 'NONE',  ( -0.000000000000000000, -0.000000000000000000, -1.000000000000000000 ) ) ;
#4103=VECTOR ( 'NONE', #24815, 1000.000000000000000 ) ;
#4107=CARTESIAN_POINT ( 'NONE',  ( -20.72055270933793736, 25.09707290294331017, -36.68877005347593467 ) ) ;
#4111=ORIENTED_EDGE ( 'NONE', *, *, #29540, .T. ) ;
#4112=EDGE_CURVE ( 'NONE', #3404, #26014, #31422, .T. ) ;
#4114=ORIENTED_EDGE ( 'NONE', *, *, #26760, .T. ) ;
#4124=LINE ( 'NONE', #3428, #5550 ) ;
#4127=EDGE_LOOP ( 'NONE', ( #32481, #23594, #22478, #16867, #7810, #26595, #31123, #34648, #27327, #23765, #12078, #4724, #5224, #25178, #13103, #22141, #24551, #15238, #7465, #29829, #5738, #32556, #19334, #18094, #9765, #3350, #16939, #30858, #29724, #3826, #25721, #1216, #25840, #12950, #6136, #26942, #22900, #1806, #30887, #27683, #26779, #32432, #27506, #10943, #412, #7981, #18433, #5744, #28230, #33496, #14248, #28777, #26789, #12760, #33737, #7662, #33550, #22826, #33219, #34049, #4114, #34964, #19370 ) ) ;
#4136=CARTESIAN_POINT ( 'NONE',  ( -20.02113311122498729, -5.758675521474015291, -67.50000000000000000 ) ) ;
#4140=DIRECTION ( 'NONE',  ( 0.6876994588534225405, -0.7259954919231316195, 0.000000000000000000 ) ) ;
#4144=CARTESIAN_POINT ( 'NONE',  ( -37.12776225901827587, -7.411627343331159246, 68.31122994652405112 ) ) ;
#4145=CARTESIAN_POINT ( 'NONE',  ( 23.93847777447631131, 22.04889236939138186, 68.31122994652405112 ) ) ;
#4149=VECTOR ( 'NONE', #15379, 999.9999999999998863 ) ;
#4150=LINE ( 'NONE', #28203, #25789 ) ;
#4152=DIRECTION ( 'NONE',  ( -0.000000000000000000, -1.836970198721029688E-16, 1.000000000000000000 ) ) ;
#4160=AXIS2_PLACEMENT_3D ( 'NONE', #11042, #5674, #30084 ) ;
#4169=ORIENTED_EDGE ( 'NONE', *, *, #30950, .F. ) ;
#4171=FACE_OUTER_BOUND ( 'NONE', #27782, .T. ) ;
#4178=PLANE ( 'NONE',  #15808 ) ;
#4179=DIRECTION ( 'NONE',  ( 0.000000000000000000, 1.836970198721029934E-16, -1.000000000000000000 ) ) ;
#4181=CARTESIAN_POINT ( 'NONE',  ( 0.000000000000000000, 3.524919873834583163E-15, 68.31122994652405112 ) ) ;
#4182=VERTEX_POINT ( 'NONE', #15946 ) ;
#4189=CARTESIAN_POINT ( 'NONE',  ( 9.736651044630752594, -33.69708579775585378, -36.68877005347594178 ) ) ;
#4193=DIRECTION ( 'NONE',  ( -1.000000000000000000, -0.000000000000000000, -0.000000000000000000 ) ) ;
#4202=DIRECTION ( 'NONE',  ( -0.9289767198167914186, -0.3701381553399144542, 0.000000000000000000 ) ) ;
#4210=ORIENTED_EDGE ( 'NONE', *, *, #12447, .T. ) ;
#4220=VERTEX_POINT ( 'NONE', #5052 ) ;
#4221=CARTESIAN_POINT ( 'NONE',  ( 5.510910596163086400E-15, 44.99999999999997868, 87.50000000000001421 ) ) ;
#4223=AXIS2_PLACEMENT_3D ( 'NONE', #32623, #19130, #13775 ) ;
#4224=DIRECTION ( 'NONE',  ( 0.000000000000000000, -1.836970198721029688E-16, 1.000000000000000000 ) ) ;
#4225=CARTESIAN_POINT ( 'NONE',  ( 3.235562306570555532E-30, 28.08988295778447508, -67.50000000000000000 ) ) ;
#4227=DIRECTION ( 'NONE',  ( 0.7259954919231307313, -0.6876994588534234287, -0.000000000000000000 ) ) ;
#4229=AXIS2_PLACEMENT_3D ( 'NONE', #21360, #7815, #16024 ) ;
#4233=VECTOR ( 'NONE', #16266, 1000.000000000000000 ) ;
#4234=AXIS2_PLACEMENT_3D ( 'NONE', #32610, #13415, #8580 ) ;
#4250=EDGE_LOOP ( 'NONE', ( #16563, #28610, #3845, #11351 ) ) ;
#4259=VERTEX_POINT ( 'NONE', #18258 ) ;
#4260=CARTESIAN_POINT ( 'NONE',  ( -32.17792593279633451, -19.96555837188923022, 68.31122994652405112 ) ) ;
#4261=CARTESIAN_POINT ( 'NONE',  ( -9.978866888775527855, 8.235406450278430768, -87.50000000000000000 ) ) ;
#4262=CIRCLE ( 'NONE', #8820, 32.54542015209054995 ) ;
#4264=LINE ( 'NONE', #25987, #4434 ) ;
#4265=ORIENTED_EDGE ( 'NONE', *, *, #2309, .F. ) ;
#4269=CARTESIAN_POINT ( 'NONE',  ( 8.986540508143578521, 33.69708579775584667, 49.43553178847298568 ) ) ;
#4273=ORIENTED_EDGE ( 'NONE', *, *, #4986, .F. ) ;
#4276=ADVANCED_FACE ( 'NONE', ( #26250 ), #10595, .F. ) ;
#4278=CARTESIAN_POINT ( 'NONE',  ( -35.00000000000000000, -4.831299144296466785, -15.81122994652406355 ) ) ;
#4279=PLANE ( 'NONE',  #11712 ) ;
#4284=EDGE_CURVE ( 'NONE', #30712, #2971, #34800, .T. ) ;
#4288=EDGE_CURVE ( 'NONE', #12838, #28732, #5222, .T. ) ;
#4289=ADVANCED_FACE ( 'NONE', ( #29281 ), #4873, .F. ) ;
#4292=AXIS2_PLACEMENT_3D ( 'NONE', #4869, #2044, #15768 ) ;
#4294=ORIENTED_EDGE ( 'NONE', *, *, #6081, .T. ) ;
#4313=DIRECTION ( 'NONE',  ( 0.000000000000000000, -1.836970198721029934E-16, 1.000000000000000000 ) ) ;
#4316=VERTEX_POINT ( 'NONE', #13970 ) ;
#4317=LINE ( 'NONE', #15202, #15106 ) ;
#4324=CARTESIAN_POINT ( 'NONE',  ( -1.307386931792819285, 32.51914993179678959, 68.31122994652405112 ) ) ;
#4325=ORIENTED_EDGE ( 'NONE', *, *, #324, .F. ) ;
#4332=ADVANCED_FACE ( 'NONE', ( #3268 ), #2908, .F. ) ;
#4333=DIRECTION ( 'NONE',  ( 1.000000000000000000, 0.000000000000000000, -0.000000000000000000 ) ) ;
#4337=LINE ( 'NONE', #26232, #24741 ) ;
#4343=EDGE_CURVE ( 'NONE', #3555, #18475, #16832, .T. ) ;
#4344=AXIS2_PLACEMENT_3D ( 'NONE', #31130, #25423, #11744 ) ;
#4348=EDGE_LOOP ( 'NONE', ( #21678, #3670, #12559, #13536 ) ) ;
#4352=EDGE_CURVE ( 'NONE', #5869, #3078, #14204, .T. ) ;
#4355=ORIENTED_EDGE ( 'NONE', *, *, #22212, .F. ) ;
#4362=ADVANCED_FACE ( 'NONE', ( #6984 ), #33696, .F. ) ;
#4371=VECTOR ( 'NONE', #6199, 1000.000000000000000 ) ;
#4389=ORIENTED_EDGE ( 'NONE', *, *, #25837, .T. ) ;
#4395=ADVANCED_FACE ( 'NONE', ( #14501 ), #19841, .F. ) ;
#4405=VECTOR ( 'NONE', #7544, 1000.000000000000000 ) ;
#4408=ORIENTED_EDGE ( 'NONE', *, *, #23641, .F. ) ;
#4409=FACE_OUTER_BOUND ( 'NONE', #21454, .T. ) ;
#4414=DIRECTION ( 'NONE',  ( 0.000000000000000000, 0.000000000000000000, 1.000000000000000000 ) ) ;
#4417=VECTOR ( 'NONE', #1425, 1000.000000000000000 ) ;
#4424=PLANE ( 'NONE',  #21276 ) ;
#4428=CARTESIAN_POINT ( 'NONE',  ( -18.07349068442144358, -27.06572199953719604, -36.68877005347593467 ) ) ;
#4430=AXIS2_PLACEMENT_3D ( 'NONE', #14459, #6231, #1268 ) ;
#4434=VECTOR ( 'NONE', #10142, 1000.000000000000000 ) ;
#4442=EDGE_LOOP ( 'NONE', ( #8413, #4726, #24882, #34079 ) ) ;
#4452=CARTESIAN_POINT ( 'NONE',  ( 12.46788440507149964, 30.06253867087539078, -36.68877005347593467 ) ) ;
#4457=ORIENTED_EDGE ( 'NONE', *, *, #3918, .T. ) ;
#4463=ORIENTED_EDGE ( 'NONE', *, *, #29097, .T. ) ;
#4466=CARTESIAN_POINT ( 'NONE',  ( -35.00000000000000000, 16.36947364650383818, -36.69637551990492597 ) ) ;
#4468=VECTOR ( 'NONE', #16474, 1000.000000000000000 ) ;
#4473=ORIENTED_EDGE ( 'NONE', *, *, #8466, .T. ) ;
#4493=VECTOR ( 'NONE', #23707, 1000.000000000000114 ) ;
#4494=CARTESIAN_POINT ( 'NONE',  ( 22.89764159710615132, -1.579009122040560431, -87.50000000000000000 ) ) ;
#4495=ORIENTED_EDGE ( 'NONE', *, *, #20466, .F. ) ;
#4498=DIRECTION ( 'NONE',  ( 0.8835120444460224931, 0.4684084406997908179, 0.000000000000000000 ) ) ;
#4500=VERTEX_POINT ( 'NONE', #12002 ) ;
#4506=EDGE_LOOP ( 'NONE', ( #11278, #34670, #29150, #31565, #17856, #4597, #6221, #336 ) ) ;
#4515=DIRECTION ( 'NONE',  ( 0.000000000000000000, 1.000000000000000000, 0.000000000000000000 ) ) ;
#4521=ORIENTED_EDGE ( 'NONE', *, *, #22881, .F. ) ;
#4522=LINE ( 'NONE', #15416, #17942 ) ;
#4526=ORIENTED_EDGE ( 'NONE', *, *, #9720, .T. ) ;
#4527=PLANE ( 'NONE',  #26440 ) ;
#4530=ORIENTED_EDGE ( 'NONE', *, *, #18901, .F. ) ;
#4531=LINE ( 'NONE', #24111, #11546 ) ;
#4547=ORIENTED_EDGE ( 'NONE', *, *, #19257, .T. ) ;
#4548=FACE_OUTER_BOUND ( 'NONE', #26726, .T. ) ;
#4552=AXIS2_PLACEMENT_3D ( 'NONE', #3614, #35028, #3436 ) ;
#4555=VERTEX_POINT ( 'NONE', #4832 ) ;
#4558=CARTESIAN_POINT ( 'NONE',  ( -5.021133111224989953, -3.725253662474303784, -67.50000000000000000 ) ) ;
#4560=CARTESIAN_POINT ( 'NONE',  ( 29.82459402470852083, 33.69708579775584667, 87.50000000000000000 ) ) ;
#4574=DIRECTION ( 'NONE',  ( -1.000000000000000000, 6.792721752314501023E-48, -3.697785493223492838E-32 ) ) ;
#4575=DIRECTION ( 'NONE',  ( -0.2149704402110236556, 0.9766205557100866574, 0.000000000000000000 ) ) ;
#4585=VECTOR ( 'NONE', #19274, 1000.000000000000000 ) ;
#4586=ORIENTED_EDGE ( 'NONE', *, *, #30932, .T. ) ;
#4590=DIRECTION ( 'NONE',  ( -0.000000000000000000, -1.836970198721029688E-16, 1.000000000000000000 ) ) ;
#4591=ORIENTED_EDGE ( 'NONE', *, *, #23547, .F. ) ;
#4592=EDGE_CURVE ( 'NONE', #27567, #27216, #23881, .T. ) ;
#4597=ORIENTED_EDGE ( 'NONE', *, *, #8046, .F. ) ;
#4598=VERTEX_POINT ( 'NONE', #5179 ) ;
#4609=ADVANCED_FACE ( 'NONE', ( #7503 ), #10364, .T. ) ;
#4620=DIRECTION ( 'NONE',  ( 0.000000000000000000, 1.836970198721029688E-16, -1.000000000000000000 ) ) ;
#4625=EDGE_CURVE ( 'NONE', #26014, #11706, #2343, .T. ) ;
#4628=VECTOR ( 'NONE', #23985, 1000.000000000000000 ) ;
#4637=ORIENTED_EDGE ( 'NONE', *, *, #10693, .F. ) ;
#4638=DIRECTION ( 'NONE',  ( -0.9635499925192227977, -0.2675283385292216987, -4.914415851915313010E-17 ) ) ;
#4640=VERTEX_POINT ( 'NONE', #31548 ) ;
#4646=PLANE ( 'NONE',  #12993 ) ;
#4649=CARTESIAN_POINT ( 'NONE',  ( 5.021133111224162171, -21.54630831098063481, -87.50000000000000000 ) ) ;
#4653=CARTESIAN_POINT ( 'NONE',  ( -47.73029880539744596, 11.89540832764809508, 29.51713323100467434 ) ) ;
#4654=CIRCLE ( 'NONE', #21723, 32.54542015209056416 ) ;
#4663=DIRECTION ( 'NONE',  ( 0.000000000000000000, 1.836970198721029441E-16, -1.000000000000000000 ) ) ;
#4667=PLANE ( 'NONE',  #15751 ) ;
#4670=ORIENTED_EDGE ( 'NONE', *, *, #28427, .T. ) ;
#4671=DIRECTION ( 'NONE',  ( -1.000000000000000000, 6.792721752314501023E-48, -3.697785493223492838E-32 ) ) ;
#4683=EDGE_CURVE ( 'NONE', #28732, #18315, #21742, .T. ) ;
#4684=DIRECTION ( 'NONE',  ( -0.1452892791026231256, -0.5232846903699686081, 0.8396809859716046764 ) ) ;
#4688=PLANE ( 'NONE',  #33896 ) ;
#4690=CARTESIAN_POINT ( 'NONE',  ( -35.00000000000000000, 16.36947364650383818, -36.69637551990492597 ) ) ;
#4711=DIRECTION ( 'NONE',  ( 6.189473249308360462E-17, 0.000000000000000000, -1.000000000000000000 ) ) ;
#4714=ORIENTED_EDGE ( 'NONE', *, *, #4625, .T. ) ;
#4717=EDGE_CURVE ( 'NONE', #28240, #29230, #22278, .T. ) ;
#4720=AXIS2_PLACEMENT_3D ( 'NONE', #3623, #11846, #31049 ) ;
#4722=EDGE_CURVE ( 'NONE', #5918, #31132, #24385, .T. ) ;
#4724=ORIENTED_EDGE ( 'NONE', *, *, #28459, .T. ) ;
#4726=ORIENTED_EDGE ( 'NONE', *, *, #30913, .T. ) ;
#4729=DIRECTION ( 'NONE',  ( -1.000000000000000000, 0.000000000000000000, 0.000000000000000000 ) ) ;
#4734=ORIENTED_EDGE ( 'NONE', *, *, #6971, .T. ) ;
#4738=ORIENTED_EDGE ( 'NONE', *, *, #27574, .T. ) ;
#4739=DIRECTION ( 'NONE',  ( 0.000000000000000000, 1.000000000000000000, 0.000000000000000000 ) ) ;
#4742=CARTESIAN_POINT ( 'NONE',  ( 31.73435513276359643, 7.220462394039750542, 68.31122994652405112 ) ) ;
#4743=FACE_OUTER_BOUND ( 'NONE', #27107, .T. ) ;
#4747=DIRECTION ( 'NONE',  ( 0.000000000000000000, 1.000000000000000000, 0.000000000000000000 ) ) ;
#4751=EDGE_CURVE ( 'NONE', #4890, #29871, #30279, .T. ) ;
#4760=AXIS2_PLACEMENT_3D ( 'NONE', #27845, #28205, #9518 ) ;
#4762=DIRECTION ( 'NONE',  ( 0.5155538571770220679, 0.8568571761675890519, 0.000000000000000000 ) ) ;
#4763=LINE ( 'NONE', #23652, #8632 ) ;
#4766=VERTEX_POINT ( 'NONE', #11076 ) ;
#4776=VERTEX_POINT ( 'NONE', #8562 ) ;
#4777=DIRECTION ( 'NONE',  ( 1.000000000000000000, 0.000000000000000000, 0.000000000000000000 ) ) ;
#4780=LINE ( 'NONE', #34888, #5369 ) ;
#4781=DIRECTION ( 'NONE',  ( 0.000000000000000000, 1.000000000000000000, 0.000000000000000000 ) ) ;
#4783=ORIENTED_EDGE ( 'NONE', *, *, #34768, .F. ) ;
#4784=ORIENTED_EDGE ( 'NONE', *, *, #16537, .T. ) ;
#4785=AXIS2_PLACEMENT_3D ( 'NONE', #33326, #11812, #11979 ) ;
#4792=EDGE_CURVE ( 'NONE', #14584, #14420, #32, .T. ) ;
#4793=EDGE_CURVE ( 'NONE', #10803, #2924, #9006, .T. ) ;
#4796=FACE_OUTER_BOUND ( 'NONE', #19514, .T. ) ;
#4807=LINE ( 'NONE', #23341, #1955 ) ;
#4817=ORIENTED_EDGE ( 'NONE', *, *, #1873, .F. ) ;
#4828=LINE ( 'NONE', #29410, #9479 ) ;
#4832=CARTESIAN_POINT ( 'NONE',  ( -30.58418286738120884, -22.31615353445078043, -36.68877005347593467 ) ) ;
#4853=LINE ( 'NONE', #31907, #26523 ) ;
#4854=VECTOR ( 'NONE', #33919, 1000.000000000000227 ) ;
#4855=ORIENTED_EDGE ( 'NONE', *, *, #28938, .F. ) ;
#4861=EDGE_LOOP ( 'NONE', ( #12941, #33600, #3787, #3261, #11105, #7387 ) ) ;
#4869=CARTESIAN_POINT ( 'NONE',  ( 22.89764159710611224, 15.60017778382161246, -77.50000000000000000 ) ) ;
#4870=DIRECTION ( 'NONE',  ( 0.7259954919231307313, -0.6876994588534234287, -0.000000000000000000 ) ) ;
#4872=EDGE_CURVE ( 'NONE', #24340, #8764, #22637, .T. ) ;
#4873=PLANE ( 'NONE',  #24965 ) ;
#4876=EDGE_LOOP ( 'NONE', ( #28780, #33434, #12387, #9377 ) ) ;
#4878=DIRECTION ( 'NONE',  ( 0.1378075576670459712, -0.8405889147755769564, -0.5238505067347569710 ) ) ;
#4879=ADVANCED_FACE ( 'NONE', ( #3398 ), #11963, .T. ) ;
#4880=CARTESIAN_POINT ( 'NONE',  ( 22.89764159710611224, 15.60017778382161246, -77.50000000000000000 ) ) ;
#4885=DIRECTION ( 'NONE',  ( -0.000000000000000000, 1.836970198721029688E-16, -1.000000000000000000 ) ) ;
#4886=DIRECTION ( 'NONE',  ( 0.000000000000000000, -1.000000000000000000, -2.132064625830773463E-16 ) ) ;
#4887=CARTESIAN_POINT ( 'NONE',  ( -5.038454199367317976, -32.15304576796696523, 68.31122994652405112 ) ) ;
#4889=DIRECTION ( 'NONE',  ( 0.9289767198167918627, 0.3701381553399134550, 6.799327607689963350E-17 ) ) ;
#4890=VERTEX_POINT ( 'NONE', #9276 ) ;
#4895=DIRECTION ( 'NONE',  ( -0.000000000000000000, 1.836970198721029934E-16, -1.000000000000000000 ) ) ;
#4900=CARTESIAN_POINT ( 'NONE',  ( 0.000000000000000000, 33.69708579775584667, 49.43553178847298568 ) ) ;
#4902=VECTOR ( 'NONE', #30465, 1000.000000000000227 ) ;
#4906=ORIENTED_EDGE ( 'NONE', *, *, #13949, .T. ) ;
#4908=CYLINDRICAL_SURFACE ( 'NONE', #9349, 2.033421858999711507 ) ;
#4915=ORIENTED_EDGE ( 'NONE', *, *, #26478, .T. ) ;
#4917=DIRECTION ( 'NONE',  ( 0.000000000000000000, 0.000000000000000000, 1.000000000000000000 ) ) ;
#4925=ORIENTED_EDGE ( 'NONE', *, *, #5213, .F. ) ;
#4929=ADVANCED_FACE ( 'NONE', ( #17661 ), #19965, .F. ) ;
#4944=VECTOR ( 'NONE', #10971, 1000.000000000000000 ) ;
#4949=CIRCLE ( 'NONE', #12376, 32.54542015209056416 ) ;
#4960=FACE_OUTER_BOUND ( 'NONE', #17112, .T. ) ;
#4962=ORIENTED_EDGE ( 'NONE', *, *, #18553, .T. ) ;
#4964=CARTESIAN_POINT ( 'NONE',  ( 2.567399184519788768, -37.78162119159486565, 68.31122994652405112 ) ) ;
#4978=DIRECTION ( 'NONE',  ( 0.000000000000000000, -1.000000000000000000, -3.083952846180991760E-16 ) ) ;
#4979=CARTESIAN_POINT ( 'NONE',  ( 22.89764159710615132, -5.651112684911595352, -87.50000000000000000 ) ) ;
#4983=CARTESIAN_POINT ( 'NONE',  ( 15.44711578872680846, -28.64595934308655956, 68.31122994652405112 ) ) ;
#4984=CARTESIAN_POINT ( 'NONE',  ( -6.637260778198712075, 37.28255902965930346, -36.68877005347593467 ) ) ;
#4986=EDGE_CURVE ( 'NONE', #21129, #24766, #32025, .T. ) ;
#4991=PRODUCT_DEFINITION_CONTEXT ( 'detailed design', #27146, 'design' ) ;
#4992=EDGE_LOOP ( 'NONE', ( #13882, #8361, #15083, #8795 ) ) ;
#4993=EDGE_CURVE ( 'NONE', #26683, #33608, #23677, .T. ) ;
#4994=ORIENTED_EDGE ( 'NONE', *, *, #17509, .T. ) ;
#4997=DIRECTION ( 'NONE',  ( 0.9868265225415260300, 0.1617819965527650394, -0.000000000000000000 ) ) ;
#5000=LINE ( 'NONE', #13390, #2548 ) ;
#5010=DIRECTION ( 'NONE',  ( 1.000000000000000000, 0.000000000000000000, -0.000000000000000000 ) ) ;
#5012=CARTESIAN_POINT ( 'NONE',  ( -9.144464960067640646, -31.23432620483743705, -36.68877005347593467 ) ) ;
#5016=CARTESIAN_POINT ( 'NONE',  ( 37.71145559917817280, 3.353962854566138851, 49.43553178847298568 ) ) ;
#5029=CARTESIAN_POINT ( 'NONE',  ( -45.00000000000000000, -4.831299144296466785, -15.81122994652406355 ) ) ;
#5035=ORIENTED_EDGE ( 'NONE', *, *, #20099, .T. ) ;
#5037=EDGE_CURVE ( 'NONE', #32385, #34696, #18195, .T. ) ;
#5038=ADVANCED_FACE ( 'NONE', ( #10148 ), #23495, .T. ) ;
#5040=DIRECTION ( 'NONE',  ( 0.9075754196709571175, -0.4198891015602644883, -7.713237663339537239E-17 ) ) ;
#5052=CARTESIAN_POINT ( 'NONE',  ( -26.18205399241665177, -19.33143609808334418, -36.68877005347593467 ) ) ;
#5054=ORIENTED_EDGE ( 'NONE', *, *, #5438, .T. ) ;
#5055=VECTOR ( 'NONE', #4729, 1000.000000000000000 ) ;
#5070=DIRECTION ( 'NONE',  ( 1.000000000000000000, 0.000000000000000000, -0.000000000000000000 ) ) ;
#5081=VERTEX_POINT ( 'NONE', #25993 ) ;
#5082=CARTESIAN_POINT ( 'NONE',  ( 0.000000000000000000, 3.670182593897650235E-31, 87.50000000000000000 ) ) ;
#5090=LINE ( 'NONE', #14002, #18231 ) ;
#5095=LINE ( 'NONE', #5615, #34525 ) ;
#5096=DIRECTION ( 'NONE',  ( 0.000000000000000000, 1.000000000000000000, 0.000000000000000000 ) ) ;
#5097=DIRECTION ( 'NONE',  ( 0.000000000000000000, 1.836970198721029688E-16, -1.000000000000000000 ) ) ;
#5100=CARTESIAN_POINT ( 'NONE',  ( 3.235562306570555532E-30, -5.758675521474015291, -67.50000000000000000 ) ) ;
#5102=VERTEX_POINT ( 'NONE', #21181 ) ;
#5103=CARTESIAN_POINT ( 'NONE',  ( 22.89764159710613001, 6.310691531022070144, -77.50000000000000000 ) ) ;
#5115=DIRECTION ( 'NONE',  ( 0.9868265225415260300, -0.1617819965527647341, 0.000000000000000000 ) ) ;
#5118=EDGE_CURVE ( 'NONE', #29579, #31238, #5664, .T. ) ;
#5119=ORIENTED_EDGE ( 'NONE', *, *, #18466, .T. ) ;
#5120=ORIENTED_EDGE ( 'NONE', *, *, #21973, .F. ) ;
#5122=CARTESIAN_POINT ( 'NONE',  ( -35.00000000000000000, -4.831299144296466785, -15.81122994652406355 ) ) ;
#5124=ORIENTED_EDGE ( 'NONE', *, *, #11905, .F. ) ;
#5134=VECTOR ( 'NONE', #20438, 1000.000000000000000 ) ;
#5136=LINE ( 'NONE', #2474, #31524 ) ;
#5141=ORIENTED_EDGE ( 'NONE', *, *, #10617, .T. ) ;
#5146=VECTOR ( 'NONE', #21224, 1000.000000000000000 ) ;
#5147=VECTOR ( 'NONE', #13455, 1000.000000000000000 ) ;
#5148=DIRECTION ( 'NONE',  ( 1.000000000000000000, 0.000000000000000000, 0.000000000000000000 ) ) ;
#5150=CARTESIAN_POINT ( 'NONE',  ( -32.37866696771086339, 3.290334066652097267, -36.68877005347593467 ) ) ;
#5154=FACE_OUTER_BOUND ( 'NONE', #27045, .T. ) ;
#5156=VECTOR ( 'NONE', #16117, 1000.000000000000114 ) ;
#5159=ORIENTED_EDGE ( 'NONE', *, *, #253, .T. ) ;
#5160=DIRECTION ( 'NONE',  ( 0.000000000000000000, 1.836970198721029441E-16, -1.000000000000000000 ) ) ;
#5168=ADVANCED_FACE ( 'NONE', ( #16392 ), #27573, .F. ) ;
#5171=VERTEX_POINT ( 'NONE', #27046 ) ;
#5173=CARTESIAN_POINT ( 'NONE',  ( 10.17231796313407344, -5.651112684911598016, -77.50000000000000000 ) ) ;
#5176=CARTESIAN_POINT ( 'NONE',  ( -9.978866888775632660, -1.691831803474591833, -67.50000000000000000 ) ) ;
#5177=CIRCLE ( 'NONE', #24486, 2.033421858999710619 ) ;
#5179=CARTESIAN_POINT ( 'NONE',  ( 3.985664461616346953E-15, 32.54542015209056416, 68.31122994652405112 ) ) ;
#5181=EDGE_CURVE ( 'NONE', #29231, #27481, #13529, .T. ) ;
#5192=LINE ( 'NONE', #16087, #24187 ) ;
#5196=FACE_OUTER_BOUND ( 'NONE', #11018, .T. ) ;
#5197=CIRCLE ( 'NONE', #29631, 32.54542015209056416 ) ;
#5204=EDGE_LOOP ( 'NONE', ( #23392, #8814, #21848, #26233 ) ) ;
#5209=FACE_OUTER_BOUND ( 'NONE', #31791, .T. ) ;
#5212=CARTESIAN_POINT ( 'NONE',  ( 31.73435513276359643, 7.220462394039750542, 68.31122994652405112 ) ) ;
#5213=EDGE_CURVE ( 'NONE', #23118, #27049, #32375, .T. ) ;
#5215=CARTESIAN_POINT ( 'NONE',  ( -14.49673343639653744, 34.98409864655523904, -36.68877005347593467 ) ) ;
#5217=CARTESIAN_POINT ( 'NONE',  ( 26.04754872656010178, -19.51229300245306320, 68.31122994652405112 ) ) ;
#5218=ORIENTED_EDGE ( 'NONE', *, *, #31065, .F. ) ;
#5220=VECTOR ( 'NONE', #27147, 1000.000000000000000 ) ;
#5222=LINE ( 'NONE', #23763, #15916 ) ;
#5224=ORIENTED_EDGE ( 'NONE', *, *, #18035, .F. ) ;
#5231=ORIENTED_EDGE ( 'NONE', *, *, #20853, .F. ) ;
#5232=ADVANCED_FACE ( 'NONE', ( #13362 ), #13879, .T. ) ;
#5233=PLANE ( 'NONE',  #19482 ) ;
#5236=DIRECTION ( 'NONE',  ( 0.000000000000000000, 0.000000000000000000, -1.000000000000000000 ) ) ;
#5237=VERTEX_POINT ( 'NONE', #16919 ) ;
#5238=CARTESIAN_POINT ( 'NONE',  ( 10.17231796313407344, -1.579009122040560431, -87.50000000000000000 ) ) ;
#5240=DIRECTION ( 'NONE',  ( -0.000000000000000000, -1.836970198721029688E-16, 1.000000000000000000 ) ) ;
#5248=LINE ( 'NONE', #13112, #5220 ) ;
#5250=DIRECTION ( 'NONE',  ( 0.000000000000000000, -1.000000000000000000, -1.836970198721029934E-16 ) ) ;
#5251=EDGE_LOOP ( 'NONE', ( #20390, #31552, #25028, #22486 ) ) ;
#5262=VERTEX_POINT ( 'NONE', #17274 ) ;
#5264=EDGE_CURVE ( 'NONE', #25766, #24257, #9596, .T. ) ;
#5271=VECTOR ( 'NONE', #31778, 1000.000000000000000 ) ;
#5274=AXIS2_PLACEMENT_3D ( 'NONE', #3581, #28336, #24943 ) ;
#5279=LINE ( 'NONE', #8659, #19460 ) ;
#5280=EDGE_CURVE ( 'NONE', #1101, #12035, #25598, .T. ) ;
#5283=EDGE_CURVE ( 'NONE', #12803, #16672, #14600, .T. ) ;
#5299=DIRECTION ( 'NONE',  ( 0.000000000000000000, 1.000000000000000000, 0.000000000000000000 ) ) ;
#5300=ORIENTED_EDGE ( 'NONE', *, *, #29781, .T. ) ;
#5301=LINE ( 'NONE', #19212, #28303 ) ;
#5310=VECTOR ( 'NONE', #27370, 1000.000000000000000 ) ;
#5315=FACE_OUTER_BOUND ( 'NONE', #9021, .T. ) ;
#5316=VERTEX_POINT ( 'NONE', #11565 ) ;
#5320=ORIENTED_EDGE ( 'NONE', *, *, #19424, .T. ) ;
#5325=AXIS2_PLACEMENT_3D ( 'NONE', #32608, #32263, #7883 ) ;
#5326=AXIS2_PLACEMENT_3D ( 'NONE', #18160, #1585, #4575 ) ;
#5339=VECTOR ( 'NONE', #17607, 1000.000000000000114 ) ;
#5347=AXIS2_PLACEMENT_3D ( 'NONE', #24775, #8576, #2880 ) ;
#5368=EDGE_CURVE ( 'NONE', #27865, #19356, #17456, .T. ) ;
#5369=VECTOR ( 'NONE', #2129, 1000.000000000000000 ) ;
#5373=EDGE_CURVE ( 'NONE', #29370, #31410, #26756, .T. ) ;
#5375=LINE ( 'NONE', #26395, #4233 ) ;
#5380=VECTOR ( 'NONE', #28814, 1000.000000000000114 ) ;
#5388=CARTESIAN_POINT ( 'NONE',  ( -37.58721499952019940, -4.609089608337754385, 68.31122994652405112 ) ) ;
#5390=EDGE_CURVE ( 'NONE', #25766, #1742, #8110, .T. ) ;
#5391=VECTOR ( 'NONE', #29403, 1000.000000000000000 ) ;
#5401=EDGE_LOOP ( 'NONE', ( #20859, #16425, #11828, #26068 ) ) ;
#5403=CARTESIAN_POINT ( 'NONE',  ( 21.24400529595486020, -24.65555945140047811, 68.31122994652405112 ) ) ;
#5407=CARTESIAN_POINT ( 'NONE',  ( -35.00000000000000000, 16.36947364650383818, -36.69637551990492597 ) ) ;
#5408=EDGE_LOOP ( 'NONE', ( #26039, #23272, #28643, #17954 ) ) ;
#5409=CARTESIAN_POINT ( 'NONE',  ( -35.00000000000000000, -14.38258422898375066, 68.31122994652405112 ) ) ;
#5411=ORIENTED_EDGE ( 'NONE', *, *, #4592, .T. ) ;
#5418=ADVANCED_FACE ( 'NONE', ( #33007 ), #32669, .F. ) ;
#5419=EDGE_CURVE ( 'NONE', #14420, #16320, #7231, .T. ) ;
#5427=LINE ( 'NONE', #16318, #2918 ) ;
#5429=EDGE_LOOP ( 'NONE', ( #11822, #19601, #33767, #9833 ) ) ;
#5432=LINE ( 'NONE', #10794, #20343 ) ;
#5438=EDGE_CURVE ( 'NONE', #14972, #26158, #5526, .T. ) ;
#5442=LINE ( 'NONE', #16331, #4944 ) ;
#5446=CARTESIAN_POINT ( 'NONE',  ( 3.985664461616347742E-15, 32.54542015209057126, 87.50000000000000000 ) ) ;
#5458=CARTESIAN_POINT ( 'NONE',  ( 29.82459402470852083, -33.69708579775584667, 87.50000000000000000 ) ) ;
#5462=AXIS2_PLACEMENT_3D ( 'NONE', #999, #17398, #9009 ) ;
#5463=EDGE_CURVE ( 'NONE', #24766, #23118, #5432, .T. ) ;
#5467=CARTESIAN_POINT ( 'NONE',  ( 5.713835024271039842, 32.03991982186465748, 68.31122994652405112 ) ) ;
#5468=VECTOR ( 'NONE', #1267, 1000.000000000000000 ) ;
#5469=EDGE_LOOP ( 'NONE', ( #19997, #26673, #24979, #2826, #6751, #19896 ) ) ;
#5470=CARTESIAN_POINT ( 'NONE',  ( -36.04853892210773836, 11.59936550071288330, -36.68877005347593467 ) ) ;
#5474=VERTEX_POINT ( 'NONE', #30175 ) ;
#5479=EDGE_CURVE ( 'NONE', #8317, #33041, #27152, .T. ) ;
#5498=ORIENTED_EDGE ( 'NONE', *, *, #28764, .T. ) ;
#5500=DIRECTION ( 'NONE',  ( 4.043477172016626614E-17, 0.000000000000000000, 1.000000000000000000 ) ) ;
#5525=CARTESIAN_POINT ( 'NONE',  ( 0.000000000000000000, 3.524919873834583163E-15, 68.31122994652405112 ) ) ;
#5526=CIRCLE ( 'NONE', #32823, 2.033421858999711951 ) ;
#5528=ORIENTED_EDGE ( 'NONE', *, *, #24153, .F. ) ;
#5529=CYLINDRICAL_SURFACE ( 'NONE', #28778, 2.036051781435508801 ) ;
#5533=PLANE ( 'NONE',  #18277 ) ;
#5542=AXIS2_PLACEMENT_3D ( 'NONE', #15582, #28924, #1863 ) ;
#5550=VECTOR ( 'NONE', #14317, 1000.000000000000227 ) ;
#5551=VERTEX_POINT ( 'NONE', #3658 ) ;
#5553=ORIENTED_EDGE ( 'NONE', *, *, #15657, .F. ) ;
#5570=DIRECTION ( 'NONE',  ( -0.9476531711828030113, -0.3193015301359780622, 0.000000000000000000 ) ) ;
#5576=EDGE_CURVE ( 'NONE', #12309, #23161, #6681, .T. ) ;
#5581=DIRECTION ( 'NONE',  ( -0.7960930657056438653, -0.6051742151937650194, -1.111686998345334199E-16 ) ) ;
#5583=DIRECTION ( 'NONE',  ( -0.000000000000000000, 1.836970198721029934E-16, -1.000000000000000000 ) ) ;
#5584=CARTESIAN_POINT ( 'NONE',  ( -17.07420202168509604, 33.79163469797341435, 68.31122994652405112 ) ) ;
#5587=PLANE ( 'NONE',  #24074 ) ;
#5606=VECTOR ( 'NONE', #19875, 1000.000000000000000 ) ;
#5607=CARTESIAN_POINT ( 'NONE',  ( 4.815661544189684840, -32.18716788982705168, 68.31122994652405112 ) ) ;
#5608=DIRECTION ( 'NONE',  ( 3.697785493223492838E-32, 1.934419779023891545E-16, -1.000000000000000000 ) ) ;
#5615=CARTESIAN_POINT ( 'NONE',  ( 20.89386240318430055, 24.95297350523386015, 68.31122994652405112 ) ) ;
#5617=CIRCLE ( 'NONE', #20986, 2.085824230283342740 ) ;
#5618=DIRECTION ( 'NONE',  ( 0.000000000000000000, 1.836970198721029441E-16, -1.000000000000000000 ) ) ;
#5623=DIRECTION ( 'NONE',  ( 0.1081190184239420177, 0.9941379571543595972, -0.000000000000000000 ) ) ;
#5627=AXIS2_PLACEMENT_3D ( 'NONE', #18578, #10553, #5010 ) ;
#5632=EDGE_CURVE ( 'NONE', #15054, #29695, #4949, .T. ) ;
#5633=ADVANCED_FACE ( 'NONE', ( #33560 ), #4178, .T. ) ;
#5634=ADVANCED_FACE ( 'NONE', ( #3829 ), #9183, .F. ) ;
#5637=CARTESIAN_POINT ( 'NONE',  ( 3.235562306570555532E-30, 24.02303923978504940, -67.50000000000000000 ) ) ;
#5644=DIRECTION ( 'NONE',  ( 0.000000000000000000, 1.836970198721029688E-16, -1.000000000000000000 ) ) ;
#5647=CARTESIAN_POINT ( 'NONE',  ( 32.54460952423470133, 0.2297037030477266373, 68.31122994652405112 ) ) ;
#5653=ORIENTED_EDGE ( 'NONE', *, *, #7415, .F. ) ;
#5654=EDGE_CURVE ( 'NONE', #12217, #29695, #28923, .T. ) ;
#5655=EDGE_LOOP ( 'NONE', ( #14366, #24253, #22758, #20656 ) ) ;
#5656=ORIENTED_EDGE ( 'NONE', *, *, #23486, .T. ) ;
#5664=LINE ( 'NONE', #7995, #13629 ) ;
#5667=AXIS2_PLACEMENT_3D ( 'NONE', #26504, #4590, #34162 ) ;
#5671=VERTEX_POINT ( 'NONE', #29456 ) ;
#5674=DIRECTION ( 'NONE',  ( 0.000000000000000000, 0.000000000000000000, 1.000000000000000000 ) ) ;
#5678=LINE ( 'NONE', #2494, #22243 ) ;
#5683=DIRECTION ( 'NONE',  ( 0.000000000000000000, 1.836970198721029688E-16, -1.000000000000000000 ) ) ;
#5691=ORIENTED_EDGE ( 'NONE', *, *, #2202, .T. ) ;
#5694=LINE ( 'NONE', #23407, #24679 ) ;
#5696=CIRCLE ( 'NONE', #15472, 2.036051781435517682 ) ;
#5697=ORIENTED_EDGE ( 'NONE', *, *, #24499, .T. ) ;
#5699=DIRECTION ( 'NONE',  ( 3.697785493223492838E-32, 1.934419779023891545E-16, -1.000000000000000000 ) ) ;
#5703=DIRECTION ( 'NONE',  ( -0.9985334138511239299, 0.05413890858541753337, 0.000000000000000000 ) ) ;
#5704=CARTESIAN_POINT ( 'NONE',  ( 5.021133111224265200, -11.61907005722761532, -67.50000000000000000 ) ) ;
#5709=CIRCLE ( 'NONE', #6863, 2.033421858999711951 ) ;
#5713=AXIS2_PLACEMENT_3D ( 'NONE', #20228, #30549, #3307 ) ;
#5716=CARTESIAN_POINT ( 'NONE',  ( 20.62763069236413926, -31.74750072459299588, 68.31122994652405112 ) ) ;
#5718=EDGE_CURVE ( 'NONE', #4776, #3490, #5694, .T. ) ;
#5728=VERTEX_POINT ( 'NONE', #34797 ) ;
#5730=DIRECTION ( 'NONE',  ( 0.000000000000000000, -1.000000000000000000, -1.836970198721029688E-16 ) ) ;
#5737=LINE ( 'NONE', #16639, #22790 ) ;
#5738=ORIENTED_EDGE ( 'NONE', *, *, #30830, .F. ) ;
#5739=EDGE_LOOP ( 'NONE', ( #21856, #23526, #12653, #15325 ) ) ;
#5740=CARTESIAN_POINT ( 'NONE',  ( 13.32059394339353986, -35.43959265050634144, 68.31122994652405112 ) ) ;
#5741=CARTESIAN_POINT ( 'NONE',  ( -9.978866888775527855, 4.168562732279005090, -67.50000000000000000 ) ) ;
#5744=ORIENTED_EDGE ( 'NONE', *, *, #24115, .T. ) ;
#5748=ORIENTED_EDGE ( 'NONE', *, *, #17601, .T. ) ;
#5751=AXIS2_PLACEMENT_3D ( 'NONE', #4900, #15796, #10432 ) ;
#5754=DIRECTION ( 'NONE',  ( -0.000000000000000000, 1.836970198721029688E-16, -1.000000000000000000 ) ) ;
#5763=DIRECTION ( 'NONE',  ( -0.7259954919231307313, -0.6876994588534234287, 0.000000000000000000 ) ) ;
#5767=DIRECTION ( 'NONE',  ( -0.9985334138511239299, 0.05413890858541762358, 0.000000000000000000 ) ) ;
#5778=ORIENTED_EDGE ( 'NONE', *, *, #6154, .T. ) ;
#5789=DIRECTION ( 'NONE',  ( 0.000000000000000000, 0.000000000000000000, 1.000000000000000000 ) ) ;
#5802=AXIS2_PLACEMENT_3D ( 'NONE', #15032, #34901, #5148 ) ;
#5806=ORIENTED_EDGE ( 'NONE', *, *, #32929, .T. ) ;
#5816=DIRECTION ( 'NONE',  ( 0.000000000000000000, 1.000000000000000000, 0.000000000000000000 ) ) ;
#5820=VERTEX_POINT ( 'NONE', #14272 ) ;
#5822=EDGE_CURVE ( 'NONE', #3430, #14410, #6588, .T. ) ;
#5826=DIRECTION ( 'NONE',  ( -0.9476531711828025673, -0.3193015301359797831, -5.865473952658197586E-17 ) ) ;
#5843=PLANE ( 'NONE',  #31327 ) ;
#5848=LINE ( 'NONE', #2838, #15513 ) ;
#5850=LINE ( 'NONE', #16747, #33987 ) ;
#5854=LINE ( 'NONE', #369, #24771 ) ;
#5861=LINE ( 'NONE', #22255, #29679 ) ;
#5867=CARTESIAN_POINT ( 'NONE',  ( 10.96230482721425403, -16.64466345897533017, -77.50000000000000000 ) ) ;
#5869=VERTEX_POINT ( 'NONE', #3747 ) ;
#5886=DIRECTION ( 'NONE',  ( 0.000000000000000000, -1.000000000000000000, -1.836970198721029934E-16 ) ) ;
#5887=ORIENTED_EDGE ( 'NONE', *, *, #31119, .T. ) ;
#5893=CARTESIAN_POINT ( 'NONE',  ( 29.83064097883987742, 23.32756518004833168, 49.43553178847298568 ) ) ;
#5897=DIRECTION ( 'NONE',  ( -0.000000000000000000, -1.000000000000000000, -0.000000000000000000 ) ) ;
#5898=VECTOR ( 'NONE', #23066, 1000.000000000000000 ) ;
#5904=DIRECTION ( 'NONE',  ( -0.000000000000000000, 1.836970198721029934E-16, -1.000000000000000000 ) ) ;
#5910=ORIENTED_EDGE ( 'NONE', *, *, #13345, .T. ) ;
#5911=DIRECTION ( 'NONE',  ( 0.000000000000000000, -1.836970198721029688E-16, 1.000000000000000000 ) ) ;
#5913=EDGE_LOOP ( 'NONE', ( #10686, #15179, #10113, #25814 ) ) ;
#5914=DIRECTION ( 'NONE',  ( 0.000000000000000000, 1.836970198721029441E-16, -1.000000000000000000 ) ) ;
#5918=VERTEX_POINT ( 'NONE', #34347 ) ;
#5925=FACE_OUTER_BOUND ( 'NONE', #26464, .T. ) ;
#5932=VECTOR ( 'NONE', #26570, 1000.000000000000114 ) ;
#5933=VECTOR ( 'NONE', #23858, 1000.000000000000000 ) ;
#5935=ORIENTED_EDGE ( 'NONE', *, *, #32961, .T. ) ;
#5940=CARTESIAN_POINT ( 'NONE',  ( 0.000000000000000000, 2.296212748401288367E-15, 47.49999999999999289 ) ) ;
#5945=AXIS2_PLACEMENT_3D ( 'NONE', #13214, #4638, #1813 ) ;
#5952=AXIS2_PLACEMENT_3D ( 'NONE', #18193, #26704, #7833 ) ;
#5959=CARTESIAN_POINT ( 'NONE',  ( 0.000000000000000000, 6.992329373473909019E-15, 49.43553178847298568 ) ) ;
#5960=AXIS2_PLACEMENT_3D ( 'NONE', #11666, #27842, #11482 ) ;
#5965=PLANE ( 'NONE',  #8015 ) ;
#5967=ORIENTED_EDGE ( 'NONE', *, *, #14279, .T. ) ;
#5969=DIRECTION ( 'NONE',  ( -0.000000000000000000, 1.836970198721029934E-16, -1.000000000000000000 ) ) ;
#5976=LINE ( 'NONE', #16876, #14165 ) ;
#5981=CARTESIAN_POINT ( 'NONE',  ( -5.021133111224679091, 26.05646109878476224, -67.50000000000000000 ) ) ;
#5983=VERTEX_POINT ( 'NONE', #12650 ) ;
#6010=DIRECTION ( 'NONE',  ( 3.697785493223492838E-32, 1.934419779023891545E-16, -1.000000000000000000 ) ) ;
#6012=EDGE_CURVE ( 'NONE', #3630, #2071, #31163, .T. ) ;
#6016=VERTEX_POINT ( 'NONE', #9791 ) ;
#6025=ORIENTED_EDGE ( 'NONE', *, *, #8679, .F. ) ;
#6029=ORIENTED_EDGE ( 'NONE', *, *, #31658, .T. ) ;
#6039=ORIENTED_EDGE ( 'NONE', *, *, #3918, .F. ) ;
#6042=ORIENTED_EDGE ( 'NONE', *, *, #1262, .F. ) ;
#6043=EDGE_LOOP ( 'NONE', ( #23638, #30071, #13864, #31060 ) ) ;
#6048=ORIENTED_EDGE ( 'NONE', *, *, #27311, .F. ) ;
#6054=ORIENTED_EDGE ( 'NONE', *, *, #21261, .F. ) ;
#6055=ORIENTED_EDGE ( 'NONE', *, *, #25131, .F. ) ;
#6056=EDGE_CURVE ( 'NONE', #5551, #11743, #6763, .T. ) ;
#6067=ORIENTED_EDGE ( 'NONE', *, *, #22211, .F. ) ;
#6069=FACE_OUTER_BOUND ( 'NONE', #24835, .T. ) ;
#6070=EDGE_CURVE ( 'NONE', #11447, #14721, #22973, .T. ) ;
#6072=DIRECTION ( 'NONE',  ( 1.000000000000000000, 0.000000000000000000, -0.000000000000000000 ) ) ;
#6077=CARTESIAN_POINT ( 'NONE',  ( 10.17231796313407344, -1.579009122040562207, -77.50000000000000000 ) ) ;
#6079=CARTESIAN_POINT ( 'NONE',  ( -20.02113311122478123, 18.16264470403145026, -67.50000000000000000 ) ) ;
#6081=EDGE_CURVE ( 'NONE', #12565, #8883, #23322, .T. ) ;
#6085=VECTOR ( 'NONE', #28786, 1000.000000000000000 ) ;
#6089=EDGE_LOOP ( 'NONE', ( #5411, #29755, #24793, #32754 ) ) ;
#6090=CARTESIAN_POINT ( 'NONE',  ( 14.70109753509668948, 34.88954974633765005, 68.31122994652405112 ) ) ;
#6093=CARTESIAN_POINT ( 'NONE',  ( 36.86854689046325717, 8.645963718612074800, 68.31122994652405112 ) ) ;
#6097=ORIENTED_EDGE ( 'NONE', *, *, #15313, .T. ) ;
#6104=DIRECTION ( 'NONE',  ( 0.000000000000000000, 1.836970198721029688E-16, -1.000000000000000000 ) ) ;
#6111=CARTESIAN_POINT ( 'NONE',  ( 21.85761591200894216, 30.91355005303805825, 68.31122994652405112 ) ) ;
#6114=DIRECTION ( 'NONE',  ( -0.000000000000000000, 1.000000000000000000, 0.000000000000000000 ) ) ;
#6115=CARTESIAN_POINT ( 'NONE',  ( 22.89764159710615132, -5.651112684911597128, -77.50000000000000000 ) ) ;
#6123=CARTESIAN_POINT ( 'NONE',  ( -27.76765758629847980, -16.97532223688792996, 68.31122994652405112 ) ) ;
#6124=EDGE_CURVE ( 'NONE', #29370, #13424, #10681, .T. ) ;
#6131=VECTOR ( 'NONE', #33165, 1000.000000000000000 ) ;
#6134=CARTESIAN_POINT ( 'NONE',  ( -20.02113311122478123, 18.16264470403145026, -67.50000000000000000 ) ) ;
#6136=ORIENTED_EDGE ( 'NONE', *, *, #635, .T. ) ;
#6137=DIRECTION ( 'NONE',  ( -0.000000000000000000, 1.836970198721029934E-16, -1.000000000000000000 ) ) ;
#6149=AXIS2_PLACEMENT_3D ( 'NONE', #32681, #8302, #16685 ) ;
#6150=DIRECTION ( 'NONE',  ( 0.000000000000000000, 1.836970198721029441E-16, -1.000000000000000000 ) ) ;
#6154=EDGE_CURVE ( 'NONE', #19647, #2206, #24091, .T. ) ;
#6156=LINE ( 'NONE', #28590, #30800 ) ;
#6162=LINE ( 'NONE', #17062, #30417 ) ;
#6163=LINE ( 'NONE', #17063, #11476 ) ;
#6175=ORIENTED_EDGE ( 'NONE', *, *, #8693, .T. ) ;
#6180=DIRECTION ( 'NONE',  ( 0.3193015301359797276, -0.9476531711828024562, 0.000000000000000000 ) ) ;
#6181=CARTESIAN_POINT ( 'NONE',  ( 12.73347502555019162, -33.69708579775584667, 49.43553178847298568 ) ) ;
#6191=ORIENTED_EDGE ( 'NONE', *, *, #24749, .F. ) ;
#6199=DIRECTION ( 'NONE',  ( -0.000000000000000000, -1.836970198721029688E-16, 1.000000000000000000 ) ) ;
#6200=EDGE_CURVE ( 'NONE', #14410, #34772, #4780, .T. ) ;
#6203=LINE ( 'NONE', #891, #14674 ) ;
#6204=EDGE_CURVE ( 'NONE', #5237, #20827, #2655, .T. ) ;
#6205=CARTESIAN_POINT ( 'NONE',  ( 27.99209646187092559, 25.49206711720156093, 68.31122994652405112 ) ) ;
#6210=DIRECTION ( 'NONE',  ( 0.000000000000000000, 0.000000000000000000, 1.000000000000000000 ) ) ;
#6212=EDGE_CURVE ( 'NONE', #1742, #22309, #11650, .T. ) ;
#6213=ORIENTED_EDGE ( 'NONE', *, *, #31835, .F. ) ;
#6216=VERTEX_POINT ( 'NONE', #29367 ) ;
#6221=ORIENTED_EDGE ( 'NONE', *, *, #28520, .F. ) ;
#6226=DIRECTION ( 'NONE',  ( -0.7960930657056433102, -0.6051742151937656855, -0.000000000000000000 ) ) ;
#6231=DIRECTION ( 'NONE',  ( 0.000000000000000000, 1.836970198721029688E-16, -1.000000000000000000 ) ) ;
#6233=FACE_OUTER_BOUND ( 'NONE', #14124, .T. ) ;
#6237=CARTESIAN_POINT ( 'NONE',  ( 1.532562817202168803, 32.50931595846692801, 49.43553178847298568 ) ) ;
#6243=LINE ( 'NONE', #11803, #26397 ) ;
#6248=DIRECTION ( 'NONE',  ( -0.000000000000000000, -1.836970198721029688E-16, 1.000000000000000000 ) ) ;
#6250=EDGE_CURVE ( 'NONE', #13120, #15487, #5136, .T. ) ;
#6251=ADVANCED_FACE ( 'NONE', ( #4960 ), #15857, .F. ) ;
#6254=ADVANCED_FACE ( 'NONE', ( #7987 ), #10501, .F. ) ;
#6259=VERTEX_POINT ( 'NONE', #16555 ) ;
#6262=ORIENTED_EDGE ( 'NONE', *, *, #11143, .F. ) ;
#6268=PLANE ( 'NONE',  #6334 ) ;
#6273=DIRECTION ( 'NONE',  ( -1.000000000000000000, 6.792721752314501023E-48, -3.697785493223492838E-32 ) ) ;
#6280=CARTESIAN_POINT ( 'NONE',  ( -14.49673343639653744, 34.98409864655521773, 68.31122994652405112 ) ) ;
#6284=PLANE ( 'NONE',  #2078 ) ;
#6285=CARTESIAN_POINT ( 'NONE',  ( -35.00000000000000000, 0.000000000000000000, 0.000000000000000000 ) ) ;
#6288=DIRECTION ( 'NONE',  ( -0.8835120444460231592, 0.4684084406997895966, 0.000000000000000000 ) ) ;
#6291=LINE ( 'NONE', #796, #8735 ) ;
#6292=VECTOR ( 'NONE', #3632, 1000.000000000000000 ) ;
#6293=ORIENTED_EDGE ( 'NONE', *, *, #5264, .T. ) ;
#6296=CARTESIAN_POINT ( 'NONE',  ( -20.02113311122478123, 14.09580098603202458, -67.50000000000000000 ) ) ;
#6297=EDGE_LOOP ( 'NONE', ( #30395, #7999, #9613, #2501 ) ) ;
#6302=ORIENTED_EDGE ( 'NONE', *, *, #27872, .F. ) ;
#6305=VECTOR ( 'NONE', #24797, 1000.000000000000114 ) ;
#6307=DIRECTION ( 'NONE',  ( -0.1617819965527638459, -0.9868265225415262520, 0.000000000000000000 ) ) ;
#6317=ORIENTED_EDGE ( 'NONE', *, *, #14527, .T. ) ;
#6320=DIRECTION ( 'NONE',  ( 3.697785493223492838E-32, 1.934419779023891545E-16, -1.000000000000000000 ) ) ;
#6321=AXIS2_PLACEMENT_3D ( 'NONE', #24738, #13378, #29567 ) ;
#6330=ORIENTED_EDGE ( 'NONE', *, *, #2919, .T. ) ;
#6334=AXIS2_PLACEMENT_3D ( 'NONE', #11645, #17169, #27999 ) ;
#6350=FACE_OUTER_BOUND ( 'NONE', #28169, .T. ) ;
#6354=CARTESIAN_POINT ( 'NONE',  ( 0.000000000000000000, 3.524919873834583163E-15, 68.31122994652405112 ) ) ;
#6368=ADVANCED_FACE ( 'NONE', ( #19571 ), #30416, .F. ) ;
#6371=LINE ( 'NONE', #1050, #10265 ) ;
#6372=VECTOR ( 'NONE', #16839, 1000.000000000000000 ) ;
#6374=ORIENTED_EDGE ( 'NONE', *, *, #3857, .F. ) ;
#6378=ORIENTED_EDGE ( 'NONE', *, *, #12545, .F. ) ;
#6382=ORIENTED_EDGE ( 'NONE', *, *, #20035, .T. ) ;
#6386=LINE ( 'NONE', #17281, #22618 ) ;
#6387=CARTESIAN_POINT ( 'NONE',  ( -1.307386931792819285, 32.51914993179678959, 68.31122994652405112 ) ) ;
#6395=VECTOR ( 'NONE', #14779, 1000.000000000000000 ) ;
#6399=ORIENTED_EDGE ( 'NONE', *, *, #11262, .F. ) ;
#6401=CARTESIAN_POINT ( 'NONE',  ( 3.235562306570555532E-30, 14.09580098603202636, -87.50000000000000000 ) ) ;
#6407=DIRECTION ( 'NONE',  ( -0.9868265225415260300, 0.1617819965527648174, 0.000000000000000000 ) ) ;
#6413=CARTESIAN_POINT ( 'NONE',  ( -32.32899628990712415, -3.747048406849356361, 15.81122994652406355 ) ) ;
#6414=DIRECTION ( 'NONE',  ( 0.8276889981568901211, 0.5611870653623829419, 0.000000000000000000 ) ) ;
#6415=ORIENTED_EDGE ( 'NONE', *, *, #26079, .T. ) ;
#6417=DIRECTION ( 'NONE',  ( -0.000000000000000000, 1.836970198721029934E-16, -1.000000000000000000 ) ) ;
#6418=CARTESIAN_POINT ( 'NONE',  ( 22.10765473302597073, -14.55883922869198166, -87.50000000000000000 ) ) ;
#6419=VECTOR ( 'NONE', #6518, 1000.000000000000000 ) ;
#6436=ORIENTED_EDGE ( 'NONE', *, *, #19742, .F. ) ;
#6438=AXIS2_PLACEMENT_3D ( 'NONE', #33185, #11311, #22161 ) ;
#6441=DIRECTION ( 'NONE',  ( -0.000000000000000000, -1.836970198721029688E-16, 1.000000000000000000 ) ) ;
#6445=EDGE_CURVE ( 'NONE', #18794, #11635, #6725, .T. ) ;
#6453=LINE ( 'NONE', #3957, #913 ) ;
#6456=EDGE_CURVE ( 'NONE', #32399, #7575, #25591, .T. ) ;
#6469=PLANE ( 'NONE',  #4720 ) ;
#6470=ADVANCED_FACE ( 'NONE', ( #7242 ), #31289, .T. ) ;
#6477=ORIENTED_EDGE ( 'NONE', *, *, #33441, .F. ) ;
#6480=DIRECTION ( 'NONE',  ( 1.000000000000000000, 0.000000000000000000, 0.000000000000000000 ) ) ;
#6483=LINE ( 'NONE', #3294, #8612 ) ;
#6490=VERTEX_POINT ( 'NONE', #6552 ) ;
#6493=CARTESIAN_POINT ( 'NONE',  ( 1.532562817202168137, 32.50931595846690669, 68.31122994652405112 ) ) ;
#6494=CARTESIAN_POINT ( 'NONE',  ( 0.000000000000000000, 3.524919873834583163E-15, 68.31122994652405112 ) ) ;
#6501=LINE ( 'NONE', #1004, #32710 ) ;
#6518=DIRECTION ( 'NONE',  ( 1.000000000000000000, -0.000000000000000000, -0.000000000000000000 ) ) ;
#6519=ORIENTED_EDGE ( 'NONE', *, *, #10665, .T. ) ;
#6522=LINE ( 'NONE', #27887, #22214 ) ;
#6523=EDGE_CURVE ( 'NONE', #20123, #12309, #12610, .T. ) ;
#6527=AXIS2_PLACEMENT_3D ( 'NONE', #17471, #6210, #1241 ) ;
#6532=ORIENTED_EDGE ( 'NONE', *, *, #33927, .T. ) ;
#6533=EDGE_CURVE ( 'NONE', #16288, #6803, #9935, .T. ) ;
#6534=EDGE_CURVE ( 'NONE', #27049, #1376, #7772, .T. ) ;
#6547=AXIS2_PLACEMENT_3D ( 'NONE', #23087, #24278, #7735 ) ;
#6548=CARTESIAN_POINT ( 'NONE',  ( -20.02113311122478123, 14.09580098603202813, -87.50000000000000000 ) ) ;
#6550=CARTESIAN_POINT ( 'NONE',  ( 29.82459402470855281, 33.69708579775584667, -36.68877005347593467 ) ) ;
#6551=ORIENTED_EDGE ( 'NONE', *, *, #17155, .T. ) ;
#6552=CARTESIAN_POINT ( 'NONE',  ( 30.69344702212033127, -10.82204614554912325, 49.43553178847298568 ) ) ;
#6563=ORIENTED_EDGE ( 'NONE', *, *, #15615, .F. ) ;
#6565=EDGE_LOOP ( 'NONE', ( #11510, #6692, #3131, #10627 ) ) ;
#6574=VERTEX_POINT ( 'NONE', #15636 ) ;
#6576=EDGE_CURVE ( 'NONE', #28395, #17757, #19007, .T. ) ;
#6580=VECTOR ( 'NONE', #11975, 1000.000000000000114 ) ;
#6587=AXIS2_PLACEMENT_3D ( 'NONE', #5740, #27652, #5570 ) ;
#6588=LINE ( 'NONE', #20137, #33797 ) ;
#6592=LINE ( 'NONE', #17659, #5468 ) ;
#6596=ORIENTED_EDGE ( 'NONE', *, *, #872, .T. ) ;
#6600=VECTOR ( 'NONE', #17102, 1000.000000000000000 ) ;
#6602=LINE ( 'NONE', #22650, #15444 ) ;
#6612=EDGE_CURVE ( 'NONE', #7619, #20342, #24143, .T. ) ;
#6622=ORIENTED_EDGE ( 'NONE', *, *, #30430, .T. ) ;
#6630=ORIENTED_EDGE ( 'NONE', *, *, #28256, .F. ) ;
#6631=ORIENTED_EDGE ( 'NONE', *, *, #22348, .F. ) ;
#6632=LINE ( 'NONE', #17532, #32202 ) ;
#6633=CARTESIAN_POINT ( 'NONE',  ( -12.25939112814508825, 30.14816249862104058, -36.68877005347593467 ) ) ;
#6637=DIRECTION ( 'NONE',  ( -0.7960930657056433102, -0.6051742151937656855, -0.000000000000000000 ) ) ;
#6640=VECTOR ( 'NONE', #30947, 1000.000000000000114 ) ;
#6641=CARTESIAN_POINT ( 'NONE',  ( -35.00000000000000000, 16.36947364650383818, 36.69637551990492597 ) ) ;
#6642=CARTESIAN_POINT ( 'NONE',  ( -30.58418286738120884, -22.31615353445080174, 68.31122994652405112 ) ) ;
#6645=FACE_OUTER_BOUND ( 'NONE', #12953, .T. ) ;
#6646=PLANE ( 'NONE',  #18380 ) ;
#6651=VECTOR ( 'NONE', #14581, 999.9999999999998863 ) ;
#6660=DIRECTION ( 'NONE',  ( -0.000000000000000000, -0.000000000000000000, -1.000000000000000000 ) ) ;
#6662=ORIENTED_EDGE ( 'NONE', *, *, #2830, .T. ) ;
#6663=CIRCLE ( 'NONE', #22587, 32.54542015209057126 ) ;
#6665=EDGE_CURVE ( 'NONE', #17833, #8779, #7590, .T. ) ;
#6667=ORIENTED_EDGE ( 'NONE', *, *, #28306, .F. ) ;
#6668=FACE_OUTER_BOUND ( 'NONE', #27881, .T. ) ;
#6670=ORIENTED_EDGE ( 'NONE', *, *, #21764, .F. ) ;
#6672=EDGE_CURVE ( 'NONE', #3550, #1172, #21492, .T. ) ;
#6681=LINE ( 'NONE', #25549, #15219 ) ;
#6692=ORIENTED_EDGE ( 'NONE', *, *, #5280, .F. ) ;
#6694=AXIS2_PLACEMENT_3D ( 'NONE', #3370, #19239, #19588 ) ;
#6695=DIRECTION ( 'NONE',  ( -0.8835120444460227151, -0.4684084406997905403, -8.604523463949019211E-17 ) ) ;
#6702=LINE ( 'NONE', #23434, #12275 ) ;
#6717=VERTEX_POINT ( 'NONE', #22017 ) ;
#6725=LINE ( 'NONE', #17618, #8220 ) ;
#6729=ORIENTED_EDGE ( 'NONE', *, *, #5576, .F. ) ;
#6737=EDGE_CURVE ( 'NONE', #19775, #3490, #14195, .T. ) ;
#6748=CARTESIAN_POINT ( 'NONE',  ( -9.978866888775733912, -15.68591377522703745, -67.50000000000000000 ) ) ;
#6751=ORIENTED_EDGE ( 'NONE', *, *, #4751, .F. ) ;
#6760=CARTESIAN_POINT ( 'NONE',  ( 3.235562306570555532E-30, -15.68591377522703745, -67.50000000000000000 ) ) ;
#6763=LINE ( 'NONE', #25810, #11057 ) ;
#6766=EDGE_LOOP ( 'NONE', ( #13472, #19921, #33190, #17211, #8108, #18893 ) ) ;
#6771=VECTOR ( 'NONE', #14334, 1000.000000000000114 ) ;
#6772=EDGE_CURVE ( 'NONE', #16556, #6917, #16874, .T. ) ;
#6773=EDGE_CURVE ( 'NONE', #33264, #31774, #24482, .T. ) ;
#6776=CARTESIAN_POINT ( 'NONE',  ( -14.84098889165989377, 28.96462362251113376, -36.68877005347593467 ) ) ;
#6777=FACE_OUTER_BOUND ( 'NONE', #13202, .T. ) ;
#6781=DIRECTION ( 'NONE',  ( 0.5155538571770231782, 0.8568571761675883858, -0.000000000000000000 ) ) ;
#6786=VERTEX_POINT ( 'NONE', #21829 ) ;
#6795=EDGE_LOOP ( 'NONE', ( #1895, #13308, #6191, #10098, #5320, #31122, #7485, #14753 ) ) ;
#6797=EDGE_CURVE ( 'NONE', #34550, #8996, #27698, .T. ) ;
#6803=VERTEX_POINT ( 'NONE', #16515 ) ;
#6806=CARTESIAN_POINT ( 'NONE',  ( 32.30227131129397833, -3.970848902647440060, 68.31122994652405112 ) ) ;
#6809=DIRECTION ( 'NONE',  ( -0.2149704402110243773, -0.9766205557100865464, -0.000000000000000000 ) ) ;
#6813=LINE ( 'NONE', #28543, #21465 ) ;
#6827=CARTESIAN_POINT ( 'NONE',  ( 10.17231796313411429, 15.60017778382161246, -77.50000000000000000 ) ) ;
#6831=DIRECTION ( 'NONE',  ( -1.000000000000000000, -0.000000000000000000, -0.000000000000000000 ) ) ;
#6838=CARTESIAN_POINT ( 'NONE',  ( -20.02113311122498729, -5.758675521474012626, -87.50000000000000000 ) ) ;
#6860=VERTEX_POINT ( 'NONE', #34094 ) ;
#6861=PLANE ( 'NONE',  #23473 ) ;
#6863=AXIS2_PLACEMENT_3D ( 'NONE', #21268, #18101, #18615 ) ;
#6870=LINE ( 'NONE', #28602, #12624 ) ;
#6893=DIRECTION ( 'NONE',  ( -0.1617819965527614312, 0.9868265225415265851, 0.000000000000000000 ) ) ;
#6903=ADVANCED_FACE ( 'NONE', ( #22730 ), #20576, .F. ) ;
#6908=VECTOR ( 'NONE', #27016, 1000.000000000000000 ) ;
#6910=PLANE ( 'NONE',  #5326 ) ;
#6917=VERTEX_POINT ( 'NONE', #9886 ) ;
#6920=EDGE_LOOP ( 'NONE', ( #14207, #24959, #21602, #28473 ) ) ;
#6924=ADVANCED_FACE ( 'NONE', ( #33748 ), #34400, .T. ) ;
#6931=CARTESIAN_POINT ( 'NONE',  ( 17.27856612038524631, 33.69708579775584667, 68.31122994652405112 ) ) ;
#6936=ORIENTED_EDGE ( 'NONE', *, *, #19698, .F. ) ;
#6938=DIRECTION ( 'NONE',  ( 0.000000000000000000, 0.000000000000000000, 1.000000000000000000 ) ) ;
#6939=CARTESIAN_POINT ( 'NONE',  ( 0.000000000000000000, 3.524919873834583163E-15, 68.31122994652405112 ) ) ;
#6944=ORIENTED_EDGE ( 'NONE', *, *, #593, .F. ) ;
#6950=DIRECTION ( 'NONE',  ( -0.000000000000000000, -0.000000000000000000, -1.000000000000000000 ) ) ;
#6952=CIRCLE ( 'NONE', #14940, 2.033421858999711951 ) ;
#6954=PLANE ( 'NONE',  #30360 ) ;
#6958=EDGE_CURVE ( 'NONE', #32277, #4182, #29461, .T. ) ;
#6965=EDGE_CURVE ( 'NONE', #29430, #29579, #12925, .T. ) ;
#6971=EDGE_CURVE ( 'NONE', #14721, #14210, #26428, .T. ) ;
#6980=ORIENTED_EDGE ( 'NONE', *, *, #24747, .T. ) ;
#6984=FACE_OUTER_BOUND ( 'NONE', #3945, .T. ) ;
#6986=FACE_OUTER_BOUND ( 'NONE', #14256, .T. ) ;
#6991=ORIENTED_EDGE ( 'NONE', *, *, #11533, .T. ) ;
#6992=CYLINDRICAL_SURFACE ( 'NONE', #34996, 2.033421858999711951 ) ;
#6993=CARTESIAN_POINT ( 'NONE',  ( 32.81769769215650712, 18.87860345536239137, 49.43553178847298568 ) ) ;
#7005=ORIENTED_EDGE ( 'NONE', *, *, #27817, .F. ) ;
#7009=EDGE_CURVE ( 'NONE', #5551, #17531, #4522, .T. ) ;
#7028=DIRECTION ( 'NONE',  ( 0.6473862847818285804, 0.7621620551276356847, 0.000000000000000000 ) ) ;
#7029=VECTOR ( 'NONE', #5236, 1000.000000000000000 ) ;
#7031=LINE ( 'NONE', #7202, #24958 ) ;
#7033=FACE_OUTER_BOUND ( 'NONE', #18283, .T. ) ;
#7035=DIRECTION ( 'NONE',  ( -0.3701381553399134550, 0.9289767198167918627, 0.000000000000000000 ) ) ;
#7036=ORIENTED_EDGE ( 'NONE', *, *, #6737, .T. ) ;
#7037=CARTESIAN_POINT ( 'NONE',  ( -1.307386931792819285, 37.83772838912469894, 68.31122994652405112 ) ) ;
#7039=DIRECTION ( 'NONE',  ( 0.000000000000000000, 0.000000000000000000, 1.000000000000000000 ) ) ;
#7045=DIRECTION ( 'NONE',  ( 0.6876994588534236508, 0.7259954919231305093, -0.000000000000000000 ) ) ;
#7046=VECTOR ( 'NONE', #8163, 1000.000000000000114 ) ;
#7058=DIRECTION ( 'NONE',  ( -0.000000000000000000, 1.836970198721029934E-16, -1.000000000000000000 ) ) ;
#7061=CARTESIAN_POINT ( 'NONE',  ( -5.021133111224886036, 8.235406450278430768, -87.50000000000000000 ) ) ;
#7062=DIRECTION ( 'NONE',  ( 0.8835120444460231592, -0.4684084406997896521, -0.000000000000000000 ) ) ;
#7064=ORIENTED_EDGE ( 'NONE', *, *, #10997, .T. ) ;
#7085=DIRECTION ( 'NONE',  ( -0.000000000000000000, -1.836970198721029688E-16, 1.000000000000000000 ) ) ;
#7096=CARTESIAN_POINT ( 'NONE',  ( 0.000000000000000000, -44.99999999999993605, -85.22165320886810491 ) ) ;
#7099=EDGE_CURVE ( 'NONE', #20342, #4500, #13269, .T. ) ;
#7108=PLANE ( 'NONE',  #15268 ) ;
#7116=VECTOR ( 'NONE', #25192, 1000.000000000000000 ) ;
#7119=VECTOR ( 'NONE', #18584, 1000.000000000000227 ) ;
#7122=CARTESIAN_POINT ( 'NONE',  ( -27.84632068199329780, 25.66368763279036358, -36.68877005347593467 ) ) ;
#7124=CYLINDRICAL_SURFACE ( 'NONE', #7131, 2.033421858999711951 ) ;
#7127=DIRECTION ( 'NONE',  ( 0.000000000000000000, 1.836970198721029441E-16, -1.000000000000000000 ) ) ;
#7129=CARTESIAN_POINT ( 'NONE',  ( 4.979875012683822710, -33.69708579775584667, 68.31122994652405112 ) ) ;
#7131=AXIS2_PLACEMENT_3D ( 'NONE', #18365, #12151, #34191 ) ;
#7137=DIRECTION ( 'NONE',  ( 0.05413890858541753337, 0.9985334138511239299, 1.834276123671687566E-16 ) ) ;
#7144=CARTESIAN_POINT ( 'NONE',  ( 0.000000000000000000, 3.524919873834583163E-15, 68.31122994652405112 ) ) ;
#7149=CARTESIAN_POINT ( 'NONE',  ( -5.021133111224886036, 4.168562732279008642, -87.50000000000000000 ) ) ;
#7161=DIRECTION ( 'NONE',  ( 0.000000000000000000, 1.000000000000000000, 0.000000000000000000 ) ) ;
#7162=EDGE_CURVE ( 'NONE', #20346, #2324, #24620, .T. ) ;
#7164=LINE ( 'NONE', #26050, #26882 ) ;
#7172=CARTESIAN_POINT ( 'NONE',  ( 18.63894936814906345, 26.67946662374789213, 68.31122994652405112 ) ) ;
#7174=AXIS2_PLACEMENT_3D ( 'NONE', #16697, #9553, #28933 ) ;
#7180=EDGE_CURVE ( 'NONE', #4182, #12655, #33354, .T. ) ;
#7181=EDGE_CURVE ( 'NONE', #7314, #17657, #11470, .T. ) ;
#7188=VECTOR ( 'NONE', #31512, 1000.000000000000000 ) ;
#7189=VECTOR ( 'NONE', #23971, 1000.000000000000227 ) ;
#7190=DIRECTION ( 'NONE',  ( -0.000000000000000000, 1.836970198721029934E-16, -1.000000000000000000 ) ) ;
#7194=DIRECTION ( 'NONE',  ( -0.2675283385292208105, -0.9635499925192230197, -1.770012621235684061E-16 ) ) ;
#7196=DIRECTION ( 'NONE',  ( -1.000000000000000000, 0.000000000000000000, 0.000000000000000000 ) ) ;
#7200=EDGE_LOOP ( 'NONE', ( #20587, #27812, #31721, #12380 ) ) ;
#7202=CARTESIAN_POINT ( 'NONE',  ( 21.85761591200894216, 30.91355005303805825, 68.31122994652405112 ) ) ;
#7203=VERTEX_POINT ( 'NONE', #13612 ) ;
#7209=EDGE_LOOP ( 'NONE', ( #3298, #12875, #26189, #1422 ) ) ;
#7213=CARTESIAN_POINT ( 'NONE',  ( 10.17231796313411429, 13.56412600238610366, -87.50000000000000000 ) ) ;
#7221=EDGE_CURVE ( 'NONE', #22677, #11706, #13973, .T. ) ;
#7223=ORIENTED_EDGE ( 'NONE', *, *, #12244, .T. ) ;
#7224=AXIS2_PLACEMENT_3D ( 'NONE', #33026, #25374, #27868 ) ;
#7226=ORIENTED_EDGE ( 'NONE', *, *, #28366, .T. ) ;
#7231=CIRCLE ( 'NONE', #33955, 2.033421858999711507 ) ;
#7240=DIRECTION ( 'NONE',  ( 0.000000000000000000, 1.836970198721029441E-16, -1.000000000000000000 ) ) ;
#7242=FACE_OUTER_BOUND ( 'NONE', #30227, .T. ) ;
#7248=CARTESIAN_POINT ( 'NONE',  ( 14.70109753509668948, 34.88954974633765005, 68.31122994652405112 ) ) ;
#7254=EDGE_CURVE ( 'NONE', #17151, #23603, #261, .T. ) ;
#7268=CIRCLE ( 'NONE', #10708, 10.00000000000000000 ) ;
#7269=CARTESIAN_POINT ( 'NONE',  ( -18.45373714011839539, 26.80790850550480897, 68.31122994652405112 ) ) ;
#7274=CARTESIAN_POINT ( 'NONE',  ( -9.978866888775426602, 18.16264470403145026, -67.50000000000000000 ) ) ;
#7275=DIRECTION ( 'NONE',  ( 0.05413890858541543089, 0.9985334138511240409, 0.000000000000000000 ) ) ;
#7276=CARTESIAN_POINT ( 'NONE',  ( 15.04122381213380244, 28.86114964982165887, 68.31122994652405112 ) ) ;
#7278=ORIENTED_EDGE ( 'NONE', *, *, #27033, .T. ) ;
#7289=EDGE_CURVE ( 'NONE', #28866, #33527, #20194, .T. ) ;
#7292=EDGE_CURVE ( 'NONE', #9877, #7307, #18547, .T. ) ;
#7296=AXIS2_PLACEMENT_3D ( 'NONE', #16518, #13836, #24669 ) ;
#7298=CARTESIAN_POINT ( 'NONE',  ( -21.41424479178918361, -24.50784553716280101, 68.31122994652405112 ) ) ;
#7303=EDGE_CURVE ( 'NONE', #18637, #2425, #31044, .T. ) ;
#7305=EDGE_LOOP ( 'NONE', ( #26522, #4521, #22234, #31960 ) ) ;
#7307=VERTEX_POINT ( 'NONE', #20530 ) ;
#7314=VERTEX_POINT ( 'NONE', #8975 ) ;
#7317=VECTOR ( 'NONE', #19315, 1000.000000000000000 ) ;
#7323=DIRECTION ( 'NONE',  ( -0.7621620551276362399, -0.6473862847818278032, 0.000000000000000000 ) ) ;
#7326=PLANE ( 'NONE',  #619 ) ;
#7327=CARTESIAN_POINT ( 'NONE',  ( 29.44023756548695658, 13.87360028845404969, 49.43553178847298568 ) ) ;
#7335=LINE ( 'NONE', #31390, #4149 ) ;
#7340=EDGE_CURVE ( 'NONE', #20827, #28866, #33525, .T. ) ;
#7343=ORIENTED_EDGE ( 'NONE', *, *, #27360, .F. ) ;
#7353=ORIENTED_EDGE ( 'NONE', *, *, #6576, .T. ) ;
#7355=ORIENTED_EDGE ( 'NONE', *, *, #18035, .T. ) ;
#7357=CARTESIAN_POINT ( 'NONE',  ( -9.978866888775426602, 16.12922284503174097, -87.50000000000000000 ) ) ;
#7358=EDGE_CURVE ( 'NONE', #24110, #5728, #34051, .T. ) ;
#7363=VERTEX_POINT ( 'NONE', #17705 ) ;
#7367=DIRECTION ( 'NONE',  ( -0.9941379571543595972, -0.1081190184239421009, -1.986114147597516136E-17 ) ) ;
#7373=VERTEX_POINT ( 'NONE', #31381 ) ;
#7379=DIRECTION ( 'NONE',  ( -0.000000000000000000, 1.836970198721029934E-16, -1.000000000000000000 ) ) ;
#7380=ORIENTED_EDGE ( 'NONE', *, *, #2637, .F. ) ;
#7382=ORIENTED_EDGE ( 'NONE', *, *, #28651, .T. ) ;
#7383=EDGE_CURVE ( 'NONE', #12838, #3029, #3964, .T. ) ;
#7387=ORIENTED_EDGE ( 'NONE', *, *, #29134, .T. ) ;
#7394=CARTESIAN_POINT ( 'NONE',  ( -6.637260778198712075, 37.28255902965928215, 68.31122994652405112 ) ) ;
#7408=ORIENTED_EDGE ( 'NONE', *, *, #3088, .T. ) ;
#7412=ADVANCED_FACE ( 'NONE', ( #2526 ), #18400, .F. ) ;
#7413=DIRECTION ( 'NONE',  ( -0.000000000000000000, 1.836970198721029934E-16, -1.000000000000000000 ) ) ;
#7415=EDGE_CURVE ( 'NONE', #24798, #12655, #16079, .T. ) ;
#7416=DIRECTION ( 'NONE',  ( -0.1378075576670459157, 0.8405889147755769564, -0.5238505067347569710 ) ) ;
#7420=EDGE_CURVE ( 'NONE', #31947, #23009, #8278, .T. ) ;
#7433=FACE_OUTER_BOUND ( 'NONE', #20297, .T. ) ;
#7434=VECTOR ( 'NONE', #26794, 1000.000000000000227 ) ;
#7435=FACE_OUTER_BOUND ( 'NONE', #5655, .T. ) ;
#7446=DIRECTION ( 'NONE',  ( 1.000000000000000000, 0.000000000000000000, 0.000000000000000000 ) ) ;
#7450=CARTESIAN_POINT ( 'NONE',  ( 1.532562817202168137, 32.50931595846690669, 49.43553178847298568 ) ) ;
#7454=ORIENTED_EDGE ( 'NONE', *, *, #635, .F. ) ;
#7456=DIRECTION ( 'NONE',  ( 0.000000000000000000, 0.000000000000000000, -1.000000000000000000 ) ) ;
#7460=VECTOR ( 'NONE', #9805, 1000.000000000000000 ) ;
#7461=DIRECTION ( 'NONE',  ( 1.000000000000000000, 0.000000000000000000, -0.000000000000000000 ) ) ;
#7465=ORIENTED_EDGE ( 'NONE', *, *, #12666, .T. ) ;
#7468=CARTESIAN_POINT ( 'NONE',  ( 0.000000000000000000, 1.974842713994612024E-15, 76.74945698428001606 ) ) ;
#7483=AXIS2_PLACEMENT_3D ( 'NONE', #6387, #33625, #9249 ) ;
#7484=ORIENTED_EDGE ( 'NONE', *, *, #4288, .T. ) ;
#7485=ORIENTED_EDGE ( 'NONE', *, *, #1589, .F. ) ;
#7490=ORIENTED_EDGE ( 'NONE', *, *, #31834, .T. ) ;
#7491=EDGE_LOOP ( 'NONE', ( #19669, #17057, #15453, #12771 ) ) ;
#7497=DIRECTION ( 'NONE',  ( 1.000000000000000000, 0.000000000000000000, -0.000000000000000000 ) ) ;
#7502=CARTESIAN_POINT ( 'NONE',  ( 5.390701026406702567, -37.47456861236018000, -36.68877005347593467 ) ) ;
#7503=FACE_OUTER_BOUND ( 'NONE', #34427, .T. ) ;
#7504=CARTESIAN_POINT ( 'NONE',  ( 10.17231796313411429, 17.63622956525712127, -77.50000000000000000 ) ) ;
#7515=DIRECTION ( 'NONE',  ( 0.8276889981568903432, -0.5611870653623827199, 0.000000000000000000 ) ) ;
#7521=DIRECTION ( 'NONE',  ( 0.5611870653623813876, -0.8276889981568911203, -0.000000000000000000 ) ) ;
#7523=DIRECTION ( 'NONE',  ( -0.000000000000000000, -1.836970198721029688E-16, 1.000000000000000000 ) ) ;
#7527=VECTOR ( 'NONE', #10209, 1000.000000000000000 ) ;
#7528=AXIS2_PLACEMENT_3D ( 'NONE', #269, #10780, #2575 ) ;
#7529=ORIENTED_EDGE ( 'NONE', *, *, #12163, .T. ) ;
#7536=DIRECTION ( 'NONE',  ( 0.000000000000000000, 1.836970198721029441E-16, -1.000000000000000000 ) ) ;
#7538=EDGE_CURVE ( 'NONE', #13424, #8890, #26387, .T. ) ;
#7539=ORIENTED_EDGE ( 'NONE', *, *, #253, .F. ) ;
#7542=CYLINDRICAL_SURFACE ( 'NONE', #4292, 2.036051781435508801 ) ;
#7544=DIRECTION ( 'NONE',  ( 0.000000000000000000, 1.836970198721029441E-16, -1.000000000000000000 ) ) ;
#7545=EDGE_CURVE ( 'NONE', #28866, #29720, #34406, .T. ) ;
#7549=ADVANCED_BREP_SHAPE_REPRESENTATION ( '', ( #34166, #28566 ), #18940 ) ;
#7553=VERTEX_POINT ( 'NONE', #2007 ) ;
#7555=LINE ( 'NONE', #13098, #29682 ) ;
#7556=DIRECTION ( 'NONE',  ( 0.1081190184239417262, 0.9941379571543595972, 0.000000000000000000 ) ) ;
#7560=VERTEX_POINT ( 'NONE', #10198 ) ;
#7561=VECTOR ( 'NONE', #30203, 1000.000000000000000 ) ;
#7562=VECTOR ( 'NONE', #20326, 1000.000000000000114 ) ;
#7567=ORIENTED_EDGE ( 'NONE', *, *, #19823, .T. ) ;
#7569=DIRECTION ( 'NONE',  ( 0.000000000000000000, 1.836970198721029441E-16, -1.000000000000000000 ) ) ;
#7571=VECTOR ( 'NONE', #27548, 1000.000000000000114 ) ;
#7573=ORIENTED_EDGE ( 'NONE', *, *, #25922, .T. ) ;
#7575=VERTEX_POINT ( 'NONE', #5016 ) ;
#7589=CARTESIAN_POINT ( 'NONE',  ( 32.40067729534749219, 3.066020821660475626, 49.43553178847298568 ) ) ;
#7590=LINE ( 'NONE', #4742, #9413 ) ;
#7599=ADVANCED_FACE ( 'NONE', ( #19104 ), #32422, .T. ) ;
#7610=ADVANCED_FACE ( 'NONE', ( #32597 ), #27443, .T. ) ;
#7619=VERTEX_POINT ( 'NONE', #3053 ) ;
#7624=LINE ( 'NONE', #2812, #27143 ) ;
#7643=VECTOR ( 'NONE', #33781, 1000.000000000000114 ) ;
#7645=CARTESIAN_POINT ( 'NONE',  ( 20.89386240318430410, 24.95297350523386726, 68.31122994652405112 ) ) ;
#7649=ORIENTED_EDGE ( 'NONE', *, *, #20685, .T. ) ;
#7662=ORIENTED_EDGE ( 'NONE', *, *, #25232, .T. ) ;
#7670=ORIENTED_EDGE ( 'NONE', *, *, #12272, .F. ) ;
#7678=ORIENTED_EDGE ( 'NONE', *, *, #23750, .T. ) ;
#7682=DIRECTION ( 'NONE',  ( -0.000000000000000000, -0.000000000000000000, -1.000000000000000000 ) ) ;
#7689=CARTESIAN_POINT ( 'NONE',  ( 13.32059394339353986, -35.43959265050634144, 68.31122994652405112 ) ) ;
#7692=AXIS2_PLACEMENT_3D ( 'NONE', #26879, #21717, #11043 ) ;
#7699=DIRECTION ( 'NONE',  ( 0.1081190184239420177, 0.9941379571543595972, -0.000000000000000000 ) ) ;
#7703=ORIENTED_EDGE ( 'NONE', *, *, #34768, .T. ) ;
#7704=EDGE_CURVE ( 'NONE', #32148, #10173, #21931, .T. ) ;
#7713=VERTEX_POINT ( 'NONE', #2872 ) ;
#7714=FACE_BOUND ( 'NONE', #32822, .T. ) ;
#7720=DIRECTION ( 'NONE',  ( -0.8276889981568903432, 0.5611870653623828309, 0.000000000000000000 ) ) ;
#7725=CARTESIAN_POINT ( 'NONE',  ( 5.021133111224473033, 6.201984591278717041, -67.50000000000000000 ) ) ;
#7735=DIRECTION ( 'NONE',  ( -0.9635499925192231307, -0.2675283385292199223, 0.000000000000000000 ) ) ;
#7736=CARTESIAN_POINT ( 'NONE',  ( 29.44023756548696369, 13.87360028845404969, 68.31122994652405112 ) ) ;
#7740=DIRECTION ( 'NONE',  ( 0.000000000000000000, -1.000000000000000000, -2.132064625830773463E-16 ) ) ;
#7742=LINE ( 'NONE', #15959, #8151 ) ;
#7746=CARTESIAN_POINT ( 'NONE',  ( -10.84269519964070305, -36.27449394610879096, 68.31122994652405112 ) ) ;
#7748=ORIENTED_EDGE ( 'NONE', *, *, #27426, .F. ) ;
#7750=FACE_OUTER_BOUND ( 'NONE', #6089, .T. ) ;
#7755=VECTOR ( 'NONE', #34003, 1000.000000000000000 ) ;
#7765=ORIENTED_EDGE ( 'NONE', *, *, #15906, .T. ) ;
#7766=ORIENTED_EDGE ( 'NONE', *, *, #34557, .T. ) ;
#7767=CARTESIAN_POINT ( 'NONE',  ( 5.021133111224473033, 4.168562732279004202, -67.50000000000000000 ) ) ;
#7771=FACE_OUTER_BOUND ( 'NONE', #29126, .T. ) ;
#7772=LINE ( 'NONE', #2260, #15641 ) ;
#7773=DIRECTION ( 'NONE',  ( 0.000000000000000000, -1.836970198721029934E-16, 1.000000000000000000 ) ) ;
#7776=VERTEX_POINT ( 'NONE', #17136 ) ;
#7782=AXIS2_PLACEMENT_3D ( 'NONE', #34344, #32017, #4777 ) ;
#7788=EDGE_LOOP ( 'NONE', ( #21908, #34638, #6025, #31710 ) ) ;
#7790=ADVANCED_FACE ( 'NONE', ( #33484 ), #11967, .F. ) ;
#7795=ORIENTED_EDGE ( 'NONE', *, *, #12555, .F. ) ;
#7801=DIRECTION ( 'NONE',  ( 0.000000000000000000, 1.836970198721029934E-16, -1.000000000000000000 ) ) ;
#7810=ORIENTED_EDGE ( 'NONE', *, *, #19794, .F. ) ;
#7811=PLANE ( 'NONE',  #1043 ) ;
#7815=DIRECTION ( 'NONE',  ( 0.000000000000000000, 1.000000000000000000, 1.836970198721029688E-16 ) ) ;
#7818=ORIENTED_EDGE ( 'NONE', *, *, #15617, .F. ) ;
#7819=VERTEX_POINT ( 'NONE', #7248 ) ;
#7825=ORIENTED_EDGE ( 'NONE', *, *, #18799, .F. ) ;
#7826=DIRECTION ( 'NONE',  ( 1.000000000000000000, 0.000000000000000000, 0.000000000000000000 ) ) ;
#7833=DIRECTION ( 'NONE',  ( 0.000000000000000000, 1.836970198721029934E-16, -1.000000000000000000 ) ) ;
#7834=DIRECTION ( 'NONE',  ( 0.000000000000000000, 1.836970198721029441E-16, -1.000000000000000000 ) ) ;
#7865=EDGE_CURVE ( 'NONE', #21604, #32940, #13421, .T. ) ;
#7871=VECTOR ( 'NONE', #33795, 1000.000000000000114 ) ;
#7873=DIRECTION ( 'NONE',  ( 0.000000000000000000, 1.000000000000000000, 0.000000000000000000 ) ) ;
#7878=VECTOR ( 'NONE', #33084, 1000.000000000000000 ) ;
#7882=VECTOR ( 'NONE', #25195, 1000.000000000000000 ) ;
#7883=DIRECTION ( 'NONE',  ( 0.000000000000000000, 1.000000000000000000, 0.000000000000000000 ) ) ;
#7886=LINE ( 'NONE', #23896, #7527 ) ;
#7892=EDGE_CURVE ( 'NONE', #19057, #8463, #21498, .T. ) ;
#7896=FACE_BOUND ( 'NONE', #20563, .T. ) ;
#7903=VECTOR ( 'NONE', #8740, 1000.000000000000000 ) ;
#7904=LINE ( 'NONE', #26072, #29894 ) ;
#7906=VERTEX_POINT ( 'NONE', #8314 ) ;
#7919=CARTESIAN_POINT ( 'NONE',  ( -32.71222340678873053, 19.07754906224033675, 68.31122994652405112 ) ) ;
#7920=ORIENTED_EDGE ( 'NONE', *, *, #522, .T. ) ;
#7923=ORIENTED_EDGE ( 'NONE', *, *, #15699, .T. ) ;
#7924=LINE ( 'NONE', #29297, #5271 ) ;
#7938=EDGE_CURVE ( 'NONE', #17702, #28091, #27009, .T. ) ;
#7939=AXIS2_PLACEMENT_3D ( 'NONE', #5082, #32149, #10967 ) ;
#7948=ADVANCED_FACE ( 'NONE', ( #26477 ), #2618, .T. ) ;
#7954=DIRECTION ( 'NONE',  ( -0.000000000000000000, -0.000000000000000000, -1.000000000000000000 ) ) ;
#7962=ORIENTED_EDGE ( 'NONE', *, *, #34586, .F. ) ;
#7976=EDGE_CURVE ( 'NONE', #18566, #13940, #10816, .T. ) ;
#7981=ORIENTED_EDGE ( 'NONE', *, *, #2919, .F. ) ;
#7985=EDGE_CURVE ( 'NONE', #11635, #19542, #33569, .T. ) ;
#7987=FACE_OUTER_BOUND ( 'NONE', #15622, .T. ) ;
#7989=ORIENTED_EDGE ( 'NONE', *, *, #7292, .T. ) ;
#7992=EDGE_CURVE ( 'NONE', #7619, #17138, #3666, .T. ) ;
#7993=DIRECTION ( 'NONE',  ( -0.2149704402110243773, -0.9766205557100865464, -0.000000000000000000 ) ) ;
#7995=CARTESIAN_POINT ( 'NONE',  ( 0.000000000000000000, 33.69708579775584667, 49.43553178847298568 ) ) ;
#7997=CARTESIAN_POINT ( 'NONE',  ( 31.83311414508816029, -6.771795677801490498, 49.43553178847298568 ) ) ;
#7999=ORIENTED_EDGE ( 'NONE', *, *, #17296, .F. ) ;
#8001=VECTOR ( 'NONE', #10017, 1000.000000000000227 ) ;
#8005=ORIENTED_EDGE ( 'NONE', *, *, #24601, .T. ) ;
#8011=DIRECTION ( 'NONE',  ( 0.000000000000000000, -1.000000000000000000, -1.836970198721029934E-16 ) ) ;
#8012=LINE ( 'NONE', #16579, #30958 ) ;
#8013=AXIS2_PLACEMENT_3D ( 'NONE', #32812, #26774, #10596 ) ;
#8014=PLANE ( 'NONE',  #20092 ) ;
#8015=AXIS2_PLACEMENT_3D ( 'NONE', #16865, #33556, #22890 ) ;
#8016=ORIENTED_EDGE ( 'NONE', *, *, #7976, .T. ) ;
#8027=LINE ( 'NONE', #32936, #20211 ) ;
#8035=LINE ( 'NONE', #5176, #943 ) ;
#8040=ORIENTED_EDGE ( 'NONE', *, *, #6772, .F. ) ;
#8046=EDGE_CURVE ( 'NONE', #28825, #24229, #661, .T. ) ;
#8051=VECTOR ( 'NONE', #20107, 1000.000000000000114 ) ;
#8062=VERTEX_POINT ( 'NONE', #2962 ) ;
#8069=FACE_BOUND ( 'NONE', #20564, .T. ) ;
#8070=ORIENTED_EDGE ( 'NONE', *, *, #14689, .F. ) ;
#8074=ADVANCED_FACE ( 'NONE', ( #19714 ), #33034, .T. ) ;
#8075=CARTESIAN_POINT ( 'NONE',  ( -45.00000000000000000, 42.49491490430484220, 36.69637551990492597 ) ) ;
#8081=DIRECTION ( 'NONE',  ( 0.000000000000000000, 1.000000000000000000, 0.000000000000000000 ) ) ;
#8089=DIRECTION ( 'NONE',  ( -1.000000000000000000, -0.000000000000000000, -0.000000000000000000 ) ) ;
#8094=PLANE ( 'NONE',  #21242 ) ;
#8098=LINE ( 'NONE', #18441, #26185 ) ;
#8104=CIRCLE ( 'NONE', #33692, 2.033421858999711951 ) ;
#8108=ORIENTED_EDGE ( 'NONE', *, *, #34271, .F. ) ;
#8110=LINE ( 'NONE', #19168, #11245 ) ;
#8113=ORIENTED_EDGE ( 'NONE', *, *, #23673, .T. ) ;
#8116=CARTESIAN_POINT ( 'NONE',  ( 22.89764159710611224, 13.56412600238610366, -77.50000000000000000 ) ) ;
#8119=ORIENTED_EDGE ( 'NONE', *, *, #19257, .F. ) ;
#8131=LINE ( 'NONE', #19011, #20414 ) ;
#8142=EDGE_CURVE ( 'NONE', #18475, #33757, #34398, .T. ) ;
#8147=LINE ( 'NONE', #22743, #33664 ) ;
#8148=ORIENTED_EDGE ( 'NONE', *, *, #30430, .F. ) ;
#8151=VECTOR ( 'NONE', #29639, 1000.000000000000000 ) ;
#8163=DIRECTION ( 'NONE',  ( 0.7621620551276367950, 0.6473862847818272481, 0.000000000000000000 ) ) ;
#8164=LINE ( 'NONE', #35067, #21534 ) ;
#8168=ORIENTED_EDGE ( 'NONE', *, *, #29090, .F. ) ;
#8175=VECTOR ( 'NONE', #24949, 1000.000000000000114 ) ;
#8182=ADVANCED_FACE ( 'NONE', ( #9712 ), #4527, .T. ) ;
#8184=LINE ( 'NONE', #32224, #13991 ) ;
#8202=VERTEX_POINT ( 'NONE', #4189 ) ;
#8207=LINE ( 'NONE', #29578, #14120 ) ;
#8208=EDGE_LOOP ( 'NONE', ( #19468, #34217, #3794, #2009 ) ) ;
#8210=CARTESIAN_POINT ( 'NONE',  ( -25.07182831876307105, -28.36910952062234870, 68.31122994652405112 ) ) ;
#8215=VERTEX_POINT ( 'NONE', #20581 ) ;
#8220=VECTOR ( 'NONE', #15111, 1000.000000000000000 ) ;
#8227=VECTOR ( 'NONE', #15339, 1000.000000000000000 ) ;
#8228=CIRCLE ( 'NONE', #32667, 10.00000000000000000 ) ;
#8231=DIRECTION ( 'NONE',  ( 0.9947866662129278836, -0.05393576583119110562, -0.08654722346309881575 ) ) ;
#8235=ADVANCED_FACE ( 'NONE', ( #7033 ), #23595, .F. ) ;
#8242=ORIENTED_EDGE ( 'NONE', *, *, #7992, .F. ) ;
#8244=ORIENTED_EDGE ( 'NONE', *, *, #32525, .T. ) ;
#8247=VECTOR ( 'NONE', #20963, 1000.000000000000000 ) ;
#8254=AXIS2_PLACEMENT_3D ( 'NONE', #5637, #8326, #1197 ) ;
#8262=ORIENTED_EDGE ( 'NONE', *, *, #17870, .T. ) ;
#8268=CARTESIAN_POINT ( 'NONE',  ( -45.00000000000000000, 42.49491490430484220, 36.69637551990492597 ) ) ;
#8272=DIRECTION ( 'NONE',  ( 0.9075754196709575616, 0.4198891015602635446, 0.000000000000000000 ) ) ;
#8277=CARTESIAN_POINT ( 'NONE',  ( -37.55078559520313064, -4.831299144296464121, 15.81122994652406710 ) ) ;
#8278=CIRCLE ( 'NONE', #23086, 2.033421858999711951 ) ;
#8281=ADVANCED_FACE ( 'NONE', ( #1365 ), #12238, .F. ) ;
#8282=EDGE_CURVE ( 'NONE', #9716, #2764, #18269, .T. ) ;
#8284=DIRECTION ( 'NONE',  ( -0.4684084406997904848, -0.8835120444460226041, -0.000000000000000000 ) ) ;
#8285=CARTESIAN_POINT ( 'NONE',  ( -28.00450684652667022, 16.58167570419054471, 68.31122994652405112 ) ) ;
#8288=ORIENTED_EDGE ( 'NONE', *, *, #10815, .T. ) ;
#8290=CARTESIAN_POINT ( 'NONE',  ( -20.02113311122488781, 6.201984591278720593, -87.50000000000000000 ) ) ;
#8293=ORIENTED_EDGE ( 'NONE', *, *, #7292, .F. ) ;
#8296=AXIS2_PLACEMENT_3D ( 'NONE', #3610, #25149, #29974 ) ;
#8302=DIRECTION ( 'NONE',  ( 3.697785493223492838E-32, 1.934419779023891545E-16, -1.000000000000000000 ) ) ;
#8311=DIRECTION ( 'NONE',  ( 0.000000000000000000, 1.836970198721029441E-16, -1.000000000000000000 ) ) ;
#8312=ORIENTED_EDGE ( 'NONE', *, *, #2961, .F. ) ;
#8313=VECTOR ( 'NONE', #4711, 1000.000000000000000 ) ;
#8314=CARTESIAN_POINT ( 'NONE',  ( -20.02113311122478123, 14.09580098603202458, -67.50000000000000000 ) ) ;
#8317=VERTEX_POINT ( 'NONE', #10415 ) ;
#8320=ORIENTED_EDGE ( 'NONE', *, *, #17017, .T. ) ;
#8326=DIRECTION ( 'NONE',  ( 0.000000000000000000, -1.000000000000000000, -1.836970198721029934E-16 ) ) ;
#8344=ORIENTED_EDGE ( 'NONE', *, *, #22707, .F. ) ;
#8351=VECTOR ( 'NONE', #10146, 1000.000000000000114 ) ;
#8358=CARTESIAN_POINT ( 'NONE',  ( -9.978866888775632660, -3.725253662474303784, -67.50000000000000000 ) ) ;
#8359=CARTESIAN_POINT ( 'NONE',  ( 5.021133111224265200, -13.65249191622732461, -87.50000000000000000 ) ) ;
#8361=ORIENTED_EDGE ( 'NONE', *, *, #31835, .T. ) ;
#8365=DIRECTION ( 'NONE',  ( 0.000000000000000000, 1.000000000000000000, 1.836970198721029688E-16 ) ) ;
#8368=CYLINDRICAL_SURFACE ( 'NONE', #7692, 2.085824230283342740 ) ;
#8371=DIRECTION ( 'NONE',  ( 3.697785493223492838E-32, 1.934419779023891545E-16, -1.000000000000000000 ) ) ;
#8375=ORIENTED_EDGE ( 'NONE', *, *, #6200, .T. ) ;
#8376=LINE ( 'NONE', #16584, #32485 ) ;
#8383=ORIENTED_EDGE ( 'NONE', *, *, #31763, .T. ) ;
#8384=CARTESIAN_POINT ( 'NONE',  ( 0.000000000000000000, 3.524919873834583163E-15, 68.31122994652405112 ) ) ;
#8390=VECTOR ( 'NONE', #13636, 1000.000000000000000 ) ;
#8393=CARTESIAN_POINT ( 'NONE',  ( -9.978866888775632660, -3.725253662474303784, -67.50000000000000000 ) ) ;
#8399=ORIENTED_EDGE ( 'NONE', *, *, #30630, .T. ) ;
#8400=VECTOR ( 'NONE', #27790, 999.9999999999998863 ) ;
#8411=CARTESIAN_POINT ( 'NONE',  ( 37.55078559520313775, -4.831299144296470338, 68.31122994652405112 ) ) ;
#8413=ORIENTED_EDGE ( 'NONE', *, *, #27426, .T. ) ;
#8423=FACE_BOUND ( 'NONE', #5408, .T. ) ;
#8424=ORIENTED_EDGE ( 'NONE', *, *, #12117, .F. ) ;
#8427=AXIS2_PLACEMENT_3D ( 'NONE', #11249, #20104, #32590 ) ;
#8436=EDGE_CURVE ( 'NONE', #21178, #18207, #18448, .T. ) ;
#8439=CARTESIAN_POINT ( 'NONE',  ( -20.02113311122488781, 8.235406450278430768, -87.50000000000000000 ) ) ;
#8445=LINE ( 'NONE', #8609, #7317 ) ;
#8447=DIRECTION ( 'NONE',  ( 0.7960930657056428661, -0.6051742151937663516, 0.000000000000000000 ) ) ;
#8453=CARTESIAN_POINT ( 'NONE',  ( 0.000000000000000000, 33.69708579775584667, 49.43553178847298568 ) ) ;
#8454=ORIENTED_EDGE ( 'NONE', *, *, #19698, .T. ) ;
#8456=CARTESIAN_POINT ( 'NONE',  ( 5.021133111224473033, 4.168562732279007754, -87.50000000000000000 ) ) ;
#8458=ADVANCED_FACE ( 'NONE', ( #11129 ), #614, .T. ) ;
#8461=CARTESIAN_POINT ( 'NONE',  ( -2.791255079241054649, -37.75727539589163939, -36.68877005347593467 ) ) ;
#8462=DIRECTION ( 'NONE',  ( -0.000000000000000000, -0.000000000000000000, -1.000000000000000000 ) ) ;
#8463=VERTEX_POINT ( 'NONE', #16838 ) ;
#8466=EDGE_CURVE ( 'NONE', #21431, #6259, #11302, .T. ) ;
#8480=PLANE ( 'NONE',  #27715 ) ;
#8484=EDGE_CURVE ( 'NONE', #8779, #6860, #21979, .T. ) ;
#8487=LINE ( 'NONE', #2959, #16433 ) ;
#8488=ORIENTED_EDGE ( 'NONE', *, *, #32543, .T. ) ;
#8492=ORIENTED_EDGE ( 'NONE', *, *, #28120, .T. ) ;
#8495=CARTESIAN_POINT ( 'NONE',  ( -37.85301660235036536, 0.7430237821112573027, -15.81122994652406355 ) ) ;
#8504=ADVANCED_FACE ( 'NONE', ( #13794 ), #22328, .F. ) ;
#8505=ORIENTED_EDGE ( 'NONE', *, *, #27189, .F. ) ;
#8507=ADVANCED_FACE ( 'NONE', ( #8797 ), #6284, .F. ) ;
#8508=EDGE_CURVE ( 'NONE', #20981, #2999, #13976, .T. ) ;
#8515=DIRECTION ( 'NONE',  ( 0.000000000000000000, 1.836970198721029934E-16, -1.000000000000000000 ) ) ;
#8521=CARTESIAN_POINT ( 'NONE',  ( -36.80830595996284416, 8.862931941313773265, 68.31122994652405112 ) ) ;
#8533=CARTESIAN_POINT ( 'NONE',  ( -23.78520691327551262, 22.21414650552148373, 68.31122994652405112 ) ) ;
#8544=EDGE_CURVE ( 'NONE', #8215, #33409, #14339, .T. ) ;
#8550=VECTOR ( 'NONE', #1040, 1000.000000000000000 ) ;
#8551=CARTESIAN_POINT ( 'NONE',  ( -32.17792593279633451, -19.96555837188920890, -36.68877005347593467 ) ) ;
#8552=VERTEX_POINT ( 'NONE', #86 ) ;
#8561=PLANE ( 'NONE',  #16297 ) ;
#8562=CARTESIAN_POINT ( 'NONE',  ( -27.13361903382165963, -26.41607761506755736, -36.68877005347593467 ) ) ;
#8563=DIRECTION ( 'NONE',  ( -0.000000000000000000, 1.836970198721029934E-16, -1.000000000000000000 ) ) ;
#8566=ORIENTED_EDGE ( 'NONE', *, *, #11534, .F. ) ;
#8568=DIRECTION ( 'NONE',  ( 1.000000000000000000, 0.000000000000000000, -0.000000000000000000 ) ) ;
#8576=DIRECTION ( 'NONE',  ( 0.000000000000000000, -1.000000000000000000, -1.836970198721029934E-16 ) ) ;
#8577=LINE ( 'NONE', #19978, #31584 ) ;
#8580=DIRECTION ( 'NONE',  ( 0.000000000000000000, 1.000000000000000000, 1.934419779023891545E-16 ) ) ;
#8582=EDGE_CURVE ( 'NONE', #22067, #26131, #29987, .T. ) ;
#8584=ORIENTED_EDGE ( 'NONE', *, *, #6204, .T. ) ;
#8588=EDGE_CURVE ( 'NONE', #27945, #11027, #11661, .T. ) ;
#8590=VERTEX_POINT ( 'NONE', #14154 ) ;
#8591=FACE_OUTER_BOUND ( 'NONE', #10226, .T. ) ;
#8593=VERTEX_POINT ( 'NONE', #22861 ) ;
#8602=ORIENTED_EDGE ( 'NONE', *, *, #5718, .F. ) ;
#8607=ORIENTED_EDGE ( 'NONE', *, *, #20098, .T. ) ;
#8609=CARTESIAN_POINT ( 'NONE',  ( 3.235562306570555532E-30, 8.235406450278427215, -67.50000000000000000 ) ) ;
#8612=VECTOR ( 'NONE', #32834, 1000.000000000000000 ) ;
#8624=VECTOR ( 'NONE', #303, 1000.000000000000114 ) ;
#8628=DIRECTION ( 'NONE',  ( 0.000000000000000000, 1.836970198721029441E-16, -1.000000000000000000 ) ) ;
#8629=EDGE_CURVE ( 'NONE', #4640, #28395, #28549, .T. ) ;
#8631=ORIENTED_EDGE ( 'NONE', *, *, #9555, .F. ) ;
#8632=VECTOR ( 'NONE', #26314, 999.9999999999998863 ) ;
#8637=DIRECTION ( 'NONE',  ( 0.000000000000000000, 1.836970198721029441E-16, -1.000000000000000000 ) ) ;
#8642=LINE ( 'NONE', #27685, #11048 ) ;
#8649=DIRECTION ( 'NONE',  ( 0.000000000000000000, 1.000000000000000000, 0.000000000000000000 ) ) ;
#8650=CARTESIAN_POINT ( 'NONE',  ( 22.89764159710615132, -1.579009122040562207, -77.50000000000000000 ) ) ;
#8659=CARTESIAN_POINT ( 'NONE',  ( -2.216215597024039141, -32.46987467335850397, -36.68877005347593467 ) ) ;
#8675=DIRECTION ( 'NONE',  ( 0.000000000000000000, 1.836970198721029688E-16, -1.000000000000000000 ) ) ;
#8678=ADVANCED_FACE ( 'NONE', ( #31388 ), #6992, .F. ) ;
#8679=EDGE_CURVE ( 'NONE', #17981, #6860, #4317, .T. ) ;
#8685=LINE ( 'NONE', #14407, #18479 ) ;
#8687=AXIS2_PLACEMENT_3D ( 'NONE', #20845, #4620, #28854 ) ;
#8688=ORIENTED_EDGE ( 'NONE', *, *, #19115, .F. ) ;
#8691=ORIENTED_EDGE ( 'NONE', *, *, #4284, .T. ) ;
#8693=EDGE_CURVE ( 'NONE', #18536, #22062, #9846, .T. ) ;
#8694=CARTESIAN_POINT ( 'NONE',  ( -25.63124651156763179, 20.05601094782693394, 68.31122994652405112 ) ) ;
#8700=EDGE_CURVE ( 'NONE', #28240, #22752, #28733, .T. ) ;
#8720=LINE ( 'NONE', #544, #24157 ) ;
#8735=VECTOR ( 'NONE', #33714, 1000.000000000000000 ) ;
#8739=CARTESIAN_POINT ( 'NONE',  ( -31.68358972719164512, 7.440061483287534472, 68.31122994652405112 ) ) ;
#8740=DIRECTION ( 'NONE',  ( 0.000000000000000000, 1.836970198721029441E-16, -1.000000000000000000 ) ) ;
#8745=CARTESIAN_POINT ( 'NONE',  ( 12.46788440507149964, 30.06253867087536946, 68.31122994652405112 ) ) ;
#8750=ORIENTED_EDGE ( 'NONE', *, *, #2568, .F. ) ;
#8752=DIRECTION ( 'NONE',  ( 0.000000000000000000, 0.000000000000000000, 1.000000000000000000 ) ) ;
#8754=DIRECTION ( 'NONE',  ( 0.000000000000000000, 1.836970198721029441E-16, -1.000000000000000000 ) ) ;
#8764=VERTEX_POINT ( 'NONE', #18228 ) ;
#8765=VECTOR ( 'NONE', #10164, 1000.000000000000114 ) ;
#8766=AXIS2_PLACEMENT_3D ( 'NONE', #24960, #31489, #19996 ) ;
#8772=EDGE_CURVE ( 'NONE', #21158, #1876, #21587, .T. ) ;
#8779=VERTEX_POINT ( 'NONE', #18586 ) ;
#8781=FACE_BOUND ( 'NONE', #13923, .T. ) ;
#8782=VECTOR ( 'NONE', #18699, 1000.000000000000114 ) ;
#8783=ADVANCED_FACE ( 'NONE', ( #26210 ), #2530, .F. ) ;
#8784=DIRECTION ( 'NONE',  ( 0.000000000000000000, 0.000000000000000000, 1.000000000000000000 ) ) ;
#8787=VERTEX_POINT ( 'NONE', #34585 ) ;
#8788=AXIS2_PLACEMENT_3D ( 'NONE', #23069, #2335, #23874 ) ;
#8795=ORIENTED_EDGE ( 'NONE', *, *, #20035, .F. ) ;
#8797=FACE_OUTER_BOUND ( 'NONE', #22085, .T. ) ;
#8803=ORIENTED_EDGE ( 'NONE', *, *, #30700, .F. ) ;
#8804=DIRECTION ( 'NONE',  ( -0.000000000000000000, 1.836970198721029934E-16, -1.000000000000000000 ) ) ;
#8805=CARTESIAN_POINT ( 'NONE',  ( -23.46927268871045058, -22.54767421130281946, -36.68877005347593467 ) ) ;
#8809=CARTESIAN_POINT ( 'NONE',  ( -23.46927268871044348, -22.54767421130285143, 68.31122994652405112 ) ) ;
#8810=VECTOR ( 'NONE', #4878, 1000.000000000000227 ) ;
#8814=ORIENTED_EDGE ( 'NONE', *, *, #12666, .F. ) ;
#8818=EDGE_LOOP ( 'NONE', ( #1777, #3697, #28289, #29176 ) ) ;
#8819=CARTESIAN_POINT ( 'NONE',  ( 6.078604839177340402, 33.69708579775584667, -36.68877005347592757 ) ) ;
#8820=AXIS2_PLACEMENT_3D ( 'NONE', #34239, #34591, #34416 ) ;
#8830=ADVANCED_FACE ( 'NONE', ( #29423 ), #13233, .F. ) ;
#8831=CARTESIAN_POINT ( 'NONE',  ( -36.80830595996284416, 8.862931941313773265, 68.31122994652405112 ) ) ;
#8834=DIRECTION ( 'NONE',  ( -0.7621620551276363509, -0.6473862847818278032, -0.000000000000000000 ) ) ;
#8854=CARTESIAN_POINT ( 'NONE',  ( -35.00000000000000000, 3.353962854566122864, -15.81122994652406355 ) ) ;
#8857=VERTEX_POINT ( 'NONE', #33133 ) ;
#8861=ORIENTED_EDGE ( 'NONE', *, *, #19938, .F. ) ;
#8863=CARTESIAN_POINT ( 'NONE',  ( -1.307386931792819285, 32.51914993179681090, 68.31122994652405112 ) ) ;
#8865=DIRECTION ( 'NONE',  ( 0.3193015301359797276, 0.9476531711828024562, -0.000000000000000000 ) ) ;
#8871=VECTOR ( 'NONE', #30613, 1000.000000000000000 ) ;
#8872=DIRECTION ( 'NONE',  ( 0.7621620551276372391, -0.6473862847818265820, -0.000000000000000000 ) ) ;
#8882=DIRECTION ( 'NONE',  ( 3.697785493223492838E-32, 1.934419779023891545E-16, -1.000000000000000000 ) ) ;
#8883=VERTEX_POINT ( 'NONE', #13753 ) ;
#8884=ORIENTED_EDGE ( 'NONE', *, *, #20769, .T. ) ;
#8890=VERTEX_POINT ( 'NONE', #5893 ) ;
#8902=VERTEX_POINT ( 'NONE', #8931 ) ;
#8923=FACE_OUTER_BOUND ( 'NONE', #24535, .T. ) ;
#8927=DIRECTION ( 'NONE',  ( 0.5155538571770231782, 0.8568571761675883858, -0.000000000000000000 ) ) ;
#8931=CARTESIAN_POINT ( 'NONE',  ( 36.10877985260814427, 11.38239727801116352, 68.31122994652405112 ) ) ;
#8933=DIRECTION ( 'NONE',  ( 1.000000000000000000, 0.000000000000000000, 0.000000000000000000 ) ) ;
#8935=FACE_OUTER_BOUND ( 'NONE', #28140, .T. ) ;
#8948=EDGE_CURVE ( 'NONE', #16070, #8857, #33964, .T. ) ;
#8953=CARTESIAN_POINT ( 'NONE',  ( -35.00000000000000711, 28.28427124746189847, -36.68877005347593467 ) ) ;
#8955=ORIENTED_EDGE ( 'NONE', *, *, #10312, .F. ) ;
#8960=ADVANCED_FACE ( 'NONE', ( #3406 ), #19451, .F. ) ;
#8963=FACE_OUTER_BOUND ( 'NONE', #21642, .T. ) ;
#8965=ORIENTED_EDGE ( 'NONE', *, *, #12068, .T. ) ;
#8974=AXIS2_PLACEMENT_3D ( 'NONE', #20571, #7196, #18098 ) ;
#8975=CARTESIAN_POINT ( 'NONE',  ( -35.00000000000000000, -14.38258422898373112, -21.76353962326704661 ) ) ;
#8978=CARTESIAN_POINT ( 'NONE',  ( 20.62763069236413926, -31.74750072459299588, 68.31122994652405112 ) ) ;
#8981=CARTESIAN_POINT ( 'NONE',  ( -35.00000000000000000, -38.34433698000722046, 36.69637551990492597 ) ) ;
#8982=PLANE ( 'NONE',  #21333 ) ;
#8994=CARTESIAN_POINT ( 'NONE',  ( 0.000000000000000000, 2.296212748401288367E-15, 47.49999999999999289 ) ) ;
#8996=VERTEX_POINT ( 'NONE', #6776 ) ;
#9006=CIRCLE ( 'NONE', #31807, 32.54542015209056416 ) ;
#9008=AXIS2_PLACEMENT_3D ( 'NONE', #10722, #21572, #32411 ) ;
#9009=DIRECTION ( 'NONE',  ( 1.000000000000000000, 0.000000000000000000, -0.000000000000000000 ) ) ;
#9013=CARTESIAN_POINT ( 'NONE',  ( -27.76765758629847269, -16.97532223688794417, 68.31122994652405112 ) ) ;
#9014=DIRECTION ( 'NONE',  ( 0.000000000000000000, -1.000000000000000000, -2.132064625830773463E-16 ) ) ;
#9015=DIRECTION ( 'NONE',  ( 1.000000000000000000, 0.000000000000000000, -0.000000000000000000 ) ) ;
#9021=EDGE_LOOP ( 'NONE', ( #5778, #11626, #6399, #4547 ) ) ;
#9030=CIRCLE ( 'NONE', #28916, 2.033421858999711951 ) ;
#9041=ADVANCED_FACE ( 'NONE', ( #34013 ), #25473, .F. ) ;
#9048=EDGE_LOOP ( 'NONE', ( #24737, #16653, #22932, #10755, #16559, #4994, #19193, #31457, #11567 ) ) ;
#9050=ORIENTED_EDGE ( 'NONE', *, *, #3846, .T. ) ;
#9053=DIRECTION ( 'NONE',  ( 0.000000000000000000, 1.836970198721029441E-16, -1.000000000000000000 ) ) ;
#9058=ORIENTED_EDGE ( 'NONE', *, *, #22055, .F. ) ;
#9062=DIRECTION ( 'NONE',  ( 3.697785493223492838E-32, 1.934419779023891545E-16, -1.000000000000000000 ) ) ;
#9064=ORIENTED_EDGE ( 'NONE', *, *, #22865, .T. ) ;
#9071=PLANE ( 'NONE',  #7483 ) ;
#9076=EDGE_CURVE ( 'NONE', #21855, #26665, #26001, .T. ) ;
#9077=ORIENTED_EDGE ( 'NONE', *, *, #31570, .F. ) ;
#9078=VECTOR ( 'NONE', #2866, 1000.000000000000000 ) ;
#9081=ADVANCED_FACE ( 'NONE', ( #31000 ), #33487, .T. ) ;
#9082=ORIENTED_EDGE ( 'NONE', *, *, #5390, .T. ) ;
#9093=AXIS2_PLACEMENT_3D ( 'NONE', #1383, #14752, #25575 ) ;
#9097=ORIENTED_EDGE ( 'NONE', *, *, #3946, .F. ) ;
#9099=CARTESIAN_POINT ( 'NONE',  ( -37.85301660235036536, 0.7430237821112573027, 68.31122994652405112 ) ) ;
#9105=ORIENTED_EDGE ( 'NONE', *, *, #31119, .F. ) ;
#9106=DIRECTION ( 'NONE',  ( -0.000000000000000000, 1.836970198721029934E-16, -1.000000000000000000 ) ) ;
#9117=EDGE_LOOP ( 'NONE', ( #1674, #2503, #685, #20378 ) ) ;
#9124=ORIENTED_EDGE ( 'NONE', *, *, #30126, .T. ) ;
#9125=ORIENTED_EDGE ( 'NONE', *, *, #25006, .F. ) ;
#9134=DIRECTION ( 'NONE',  ( -0.9289767198167918627, 0.3701381553399132329, 6.799327607689958420E-17 ) ) ;
#9136=CARTESIAN_POINT ( 'NONE',  ( 5.021133111224679091, 28.08988295778447508, -67.50000000000000000 ) ) ;
#9147=CARTESIAN_POINT ( 'NONE',  ( -5.021133111225092982, -11.61907005722761177, -87.50000000000000000 ) ) ;
#9151=EDGE_CURVE ( 'NONE', #22010, #5671, #29203, .T. ) ;
#9158=CARTESIAN_POINT ( 'NONE',  ( 10.17231796313411429, 13.56412600238610189, -77.50000000000000000 ) ) ;
#9159=CARTESIAN_POINT ( 'NONE',  ( -5.614556921127968003, -37.45022281665699637, 68.31122994652405112 ) ) ;
#9160=CARTESIAN_POINT ( 'NONE',  ( 0.000000000000000000, 3.524919873834583163E-15, 68.31122994652405112 ) ) ;
#9163=LINE ( 'NONE', #30880, #9184 ) ;
#9164=VECTOR ( 'NONE', #1654, 1000.000000000000000 ) ;
#9165=ORIENTED_EDGE ( 'NONE', *, *, #19121, .T. ) ;
#9168=ADVANCED_FACE ( 'NONE', ( #13191 ), #15505, .T. ) ;
#9172=ORIENTED_EDGE ( 'NONE', *, *, #9581, .T. ) ;
#9176=PLANE ( 'NONE',  #5462 ) ;
#9180=VERTEX_POINT ( 'NONE', #5150 ) ;
#9181=AXIS2_PLACEMENT_3D ( 'NONE', #12812, #28987, #1587 ) ;
#9183=PLANE ( 'NONE',  #24848 ) ;
#9184=VECTOR ( 'NONE', #2934, 1000.000000000000000 ) ;
#9190=PLANE ( 'NONE',  #19831 ) ;
#9193=DIRECTION ( 'NONE',  ( 0.9985334138511239299, -0.05413890858541752643, -0.000000000000000000 ) ) ;
#9199=ADVANCED_FACE ( 'NONE', ( #4796 ), #35079, .F. ) ;
#9205=VECTOR ( 'NONE', #3838, 1000.000000000000114 ) ;
#9207=AXIS2_PLACEMENT_3D ( 'NONE', #20595, #34465, #17951 ) ;
#9217=DIRECTION ( 'NONE',  ( 0.6473862847818266930, 0.7621620551276372391, 1.400068981865444109E-16 ) ) ;
#9218=CARTESIAN_POINT ( 'NONE',  ( -35.00000000000000000, 0.000000000000000000, 0.000000000000000000 ) ) ;
#9230=CARTESIAN_POINT ( 'NONE',  ( 10.17231796313409298, 4.274639749586563120, -87.50000000000000000 ) ) ;
#9234=VECTOR ( 'NONE', #24491, 1000.000000000000000 ) ;
#9237=EDGE_CURVE ( 'NONE', #20173, #8317, #30568, .T. ) ;
#9244=ADVANCED_FACE ( 'NONE', ( #34903 ), #32035, .T. ) ;
#9249=DIRECTION ( 'NONE',  ( 0.000000000000000000, 0.000000000000000000, -1.000000000000000000 ) ) ;
#9265=DIRECTION ( 'NONE',  ( -1.000000000000000000, 0.000000000000000000, 0.000000000000000000 ) ) ;
#9270=DIRECTION ( 'NONE',  ( 0.1617819965527648451, 0.9868265225415261410, 1.812770913216290044E-16 ) ) ;
#9276=CARTESIAN_POINT ( 'NONE',  ( 9.630725478591894984, 36.62364762272929397, 68.31122994652405112 ) ) ;
#9280=CARTESIAN_POINT ( 'NONE',  ( -5.021133111224886036, 6.201984591278717041, -67.50000000000000000 ) ) ;
#9281=DIRECTION ( 'NONE',  ( -1.000000000000000000, 6.792721752314501023E-48, -3.697785493223492838E-32 ) ) ;
#9286=ADVANCED_FACE ( 'NONE', ( #34538 ), #10155, .T. ) ;
#9290=CARTESIAN_POINT ( 'NONE',  ( 27.99209646187092559, 25.49206711720156093, 68.31122994652405112 ) ) ;
#9295=ORIENTED_EDGE ( 'NONE', *, *, #20714, .T. ) ;
#9310=CARTESIAN_POINT ( 'NONE',  ( -29.72561944762171393, -13.25111019240559251, 68.31122994652405112 ) ) ;
#9312=ORIENTED_EDGE ( 'NONE', *, *, #14771, .F. ) ;
#9313=DIRECTION ( 'NONE',  ( -0.000000000000000000, -1.836970198721029688E-16, 1.000000000000000000 ) ) ;
#9317=DIRECTION ( 'NONE',  ( -0.9635499925192230197, 0.2675283385292207550, 0.000000000000000000 ) ) ;
#9321=VERTEX_POINT ( 'NONE', #538 ) ;
#9337=EDGE_CURVE ( 'NONE', #4220, #1172, #10103, .T. ) ;
#9342=CARTESIAN_POINT ( 'NONE',  ( -9.978866888775632660, -1.691831803474588058, -87.50000000000000000 ) ) ;
#9345=ORIENTED_EDGE ( 'NONE', *, *, #11981, .T. ) ;
#9346=CARTESIAN_POINT ( 'NONE',  ( -35.00000000000000000, 16.36947364650383818, -36.69637551990492597 ) ) ;
#9349=AXIS2_PLACEMENT_3D ( 'NONE', #32151, #15974, #21643 ) ;
#9350=VERTEX_POINT ( 'NONE', #22073 ) ;
#9354=ORIENTED_EDGE ( 'NONE', *, *, #35020, .F. ) ;
#9361=AXIS2_PLACEMENT_3D ( 'NONE', #34949, #21416, #18761 ) ;
#9364=DIRECTION ( 'NONE',  ( 0.1081190184239419622, -0.9941379571543595972, 0.000000000000000000 ) ) ;
#9366=ORIENTED_EDGE ( 'NONE', *, *, #34187, .F. ) ;
#9367=AXIS2_PLACEMENT_3D ( 'NONE', #16804, #11274, #27629 ) ;
#9375=CARTESIAN_POINT ( 'NONE',  ( 0.000000000000000000, 1.974842713994612024E-15, 76.74945698428001606 ) ) ;
#9376=CARTESIAN_POINT ( 'NONE',  ( -14.49673343639653744, 34.98409864655521773, 68.31122994652405112 ) ) ;
#9377=ORIENTED_EDGE ( 'NONE', *, *, #34026, .T. ) ;
#9395=CARTESIAN_POINT ( 'NONE',  ( -5.021133111224782120, 14.09580098603202458, -67.50000000000000000 ) ) ;
#9398=EDGE_LOOP ( 'NONE', ( #3085, #21517, #19902, #28574 ) ) ;
#9402=CARTESIAN_POINT ( 'NONE',  ( 3.985664461616347742E-15, -32.54542015209057126, 76.74945698428001606 ) ) ;
#9403=EDGE_CURVE ( 'NONE', #5171, #5918, #5850, .T. ) ;
#9413=VECTOR ( 'NONE', #27172, 1000.000000000000000 ) ;
#9416=VERTEX_POINT ( 'NONE', #5388 ) ;
#9439=AXIS2_PLACEMENT_3D ( 'NONE', #21228, #13405, #32255 ) ;
#9448=FACE_OUTER_BOUND ( 'NONE', #19792, .T. ) ;
#9451=LINE ( 'NONE', #6401, #3971 ) ;
#9472=DIRECTION ( 'NONE',  ( 1.000000000000000000, 0.000000000000000000, 0.000000000000000000 ) ) ;
#9476=CARTESIAN_POINT ( 'NONE',  ( 0.000000000000000000, 3.214697847761802057E-14, -87.50000000000000000 ) ) ;
#9479=VECTOR ( 'NONE', #7323, 1000.000000000000114 ) ;
#9481=ADVANCED_FACE ( 'NONE', ( #12285 ), #12108, .F. ) ;
#9483=EDGE_CURVE ( 'NONE', #34419, #30924, #6386, .T. ) ;
#9489=EDGE_CURVE ( 'NONE', #15441, #33917, #3542, .T. ) ;
#9492=ORIENTED_EDGE ( 'NONE', *, *, #13001, .F. ) ;
#9500=EDGE_CURVE ( 'NONE', #30129, #32360, #6203, .T. ) ;
#9502=CARTESIAN_POINT ( 'NONE',  ( -30.58418286738120884, -22.31615353445080174, 68.31122994652405112 ) ) ;
#9507=CARTESIAN_POINT ( 'NONE',  ( -35.00000000000000000, 8.360858262960551457, 68.31122994652405112 ) ) ;
#9512=CARTESIAN_POINT ( 'NONE',  ( 30.98406361983693103, 9.959526819984921175, 68.31122994652405112 ) ) ;
#9513=CARTESIAN_POINT ( 'NONE',  ( -9.978866888775733912, -11.61907005722761532, -67.50000000000000000 ) ) ;
#9518=DIRECTION ( 'NONE',  ( 0.000000000000000000, -1.000000000000000000, 0.000000000000000000 ) ) ;
#9519=DIRECTION ( 'NONE',  ( 0.000000000000000000, 1.000000000000000000, 0.000000000000000000 ) ) ;
#9527=VECTOR ( 'NONE', #10463, 1000.000000000000000 ) ;
#9529=ORIENTED_EDGE ( 'NONE', *, *, #22258, .T. ) ;
#9537=DIRECTION ( 'NONE',  ( 1.000000000000000000, 0.000000000000000000, -0.000000000000000000 ) ) ;
#9547=DIRECTION ( 'NONE',  ( 0.000000000000000000, 1.836970198721029934E-16, -1.000000000000000000 ) ) ;
#9552=ORIENTED_EDGE ( 'NONE', *, *, #19216, .F. ) ;
#9553=DIRECTION ( 'NONE',  ( 0.000000000000000000, 1.836970198721029688E-16, -1.000000000000000000 ) ) ;
#9554=DIRECTION ( 'NONE',  ( -0.3203292411224473168, 0.8039657716618124894, -0.5010271602200255803 ) ) ;
#9555=EDGE_CURVE ( 'NONE', #3078, #3836, #828, .T. ) ;
#9556=DIRECTION ( 'NONE',  ( 0.8568571761675904952, -0.5155538571770196254, -0.000000000000000000 ) ) ;
#9565=EDGE_CURVE ( 'NONE', #32705, #30129, #19527, .T. ) ;
#9566=EDGE_CURVE ( 'NONE', #4598, #16921, #30587, .T. ) ;
#9567=ORIENTED_EDGE ( 'NONE', *, *, #7865, .T. ) ;
#9569=DIRECTION ( 'NONE',  ( -0.000000000000000000, -1.000000000000000000, -0.000000000000000000 ) ) ;
#9571=VECTOR ( 'NONE', #21778, 1000.000000000000000 ) ;
#9574=ORIENTED_EDGE ( 'NONE', *, *, #893, .F. ) ;
#9578=FACE_OUTER_BOUND ( 'NONE', #15485, .T. ) ;
#9581=EDGE_CURVE ( 'NONE', #25253, #16922, #14188, .T. ) ;
#9591=DIRECTION ( 'NONE',  ( -1.000000000000000000, 6.792721752314501023E-48, -3.697785493223492838E-32 ) ) ;
#9592=CARTESIAN_POINT ( 'NONE',  ( -5.021133111225196011, -21.54630831098063837, -67.50000000000000000 ) ) ;
#9594=ORIENTED_EDGE ( 'NONE', *, *, #29299, .T. ) ;
#9596=CIRCLE ( 'NONE', #12452, 2.033421858999710619 ) ;
#9605=EDGE_CURVE ( 'NONE', #13218, #19961, #11165, .T. ) ;
#9607=CYLINDRICAL_SURFACE ( 'NONE', #9181, 2.033421858999711951 ) ;
#9613=ORIENTED_EDGE ( 'NONE', *, *, #5479, .F. ) ;
#9615=ORIENTED_EDGE ( 'NONE', *, *, #20466, .T. ) ;
#9619=ORIENTED_EDGE ( 'NONE', *, *, #2951, .F. ) ;
#9621=CARTESIAN_POINT ( 'NONE',  ( 14.70109753509668948, 34.88954974633767137, -36.68877005347593467 ) ) ;
#9631=AXIS2_PLACEMENT_3D ( 'NONE', #4880, #32461, #29808 ) ;
#9632=DIRECTION ( 'NONE',  ( -1.000000000000000000, 6.792721752314501023E-48, -3.697785493223492838E-32 ) ) ;
#9641=VECTOR ( 'NONE', #12520, 1000.000000000000227 ) ;
#9643=LINE ( 'NONE', #4452, #11603 ) ;
#9644=CARTESIAN_POINT ( 'NONE',  ( 3.235562306570555532E-30, 14.09580098603202636, -87.50000000000000000 ) ) ;
#9656=ORIENTED_EDGE ( 'NONE', *, *, #11143, .T. ) ;
#9672=CARTESIAN_POINT ( 'NONE',  ( -9.144464960067640646, -31.23432620483745836, 68.31122994652405112 ) ) ;
#9674=CARTESIAN_POINT ( 'NONE',  ( 22.10765473302597073, -12.47301499840864025, -77.50000000000000000 ) ) ;
#9685=CARTESIAN_POINT ( 'NONE',  ( 28.11866956577617316, 16.38733641342590985, 68.31122994652405112 ) ) ;
#9696=VECTOR ( 'NONE', #7062, 1000.000000000000000 ) ;
#9701=DIRECTION ( 'NONE',  ( 0.9635499925192229087, -0.2675283385292207550, 0.000000000000000000 ) ) ;
#9706=ORIENTED_EDGE ( 'NONE', *, *, #29976, .F. ) ;
#9712=FACE_OUTER_BOUND ( 'NONE', #13982, .T. ) ;
#9716=VERTEX_POINT ( 'NONE', #21825 ) ;
#9720=EDGE_CURVE ( 'NONE', #11190, #32452, #2725, .T. ) ;
#9745=EDGE_LOOP ( 'NONE', ( #30235, #700, #24938, #11771 ) ) ;
#9746=ORIENTED_EDGE ( 'NONE', *, *, #446, .T. ) ;
#9747=ORIENTED_EDGE ( 'NONE', *, *, #21165, .F. ) ;
#9749=DIRECTION ( 'NONE',  ( 3.697785493223492838E-32, 1.934419779023891545E-16, -1.000000000000000000 ) ) ;
#9751=AXIS2_PLACEMENT_3D ( 'NONE', #11205, #16553, #29892 ) ;
#9753=CARTESIAN_POINT ( 'NONE',  ( -26.18205399241665177, -19.33143609808336549, 68.31122994652405112 ) ) ;
#9761=AXIS2_PLACEMENT_3D ( 'NONE', #32172, #28803, #15296 ) ;
#9764=AXIS2_PLACEMENT_3D ( 'NONE', #9753, #23292, #34851 ) ;
#9765=ORIENTED_EDGE ( 'NONE', *, *, #23235, .F. ) ;
#9769=LINE ( 'NONE', #17633, #31480 ) ;
#9772=CARTESIAN_POINT ( 'NONE',  ( 0.000000000000000000, -33.69708579775584667, 49.43553178847298568 ) ) ;
#9776=CIRCLE ( 'NONE', #18805, 2.033421858999711951 ) ;
#9781=AXIS2_PLACEMENT_3D ( 'NONE', #34871, #20984, #31823 ) ;
#9782=LINE ( 'NONE', #25976, #29471 ) ;
#9791=CARTESIAN_POINT ( 'NONE',  ( 5.021133111224576062, 18.16264470403145381, -87.50000000000000000 ) ) ;
#9792=CARTESIAN_POINT ( 'NONE',  ( 10.62930655775863364, -36.34639295086972766, 68.31122994652405112 ) ) ;
#9794=ORIENTED_EDGE ( 'NONE', *, *, #28371, .F. ) ;
#9796=ORIENTED_EDGE ( 'NONE', *, *, #18407, .F. ) ;
#9800=ORIENTED_EDGE ( 'NONE', *, *, #7704, .F. ) ;
#9805=DIRECTION ( 'NONE',  ( 0.000000000000000000, 1.836970198721029441E-16, -1.000000000000000000 ) ) ;
#9813=LINE ( 'NONE', #4983, #4025 ) ;
#9816=( NAMED_UNIT ( * ) PLANE_ANGLE_UNIT ( ) SI_UNIT ( $, .RADIAN. ) );
#9821=VERTEX_POINT ( 'NONE', #17298 ) ;
#9824=EDGE_CURVE ( 'NONE', #25488, #32966, #27596, .T. ) ;
#9826=EDGE_CURVE ( 'NONE', #23287, #20094, #30978, .T. ) ;
#9827=ORIENTED_EDGE ( 'NONE', *, *, #1886, .F. ) ;
#9833=ORIENTED_EDGE ( 'NONE', *, *, #22980, .T. ) ;
#9835=DIRECTION ( 'NONE',  ( -0.9985334138511239299, 0.05413890858541762358, 0.000000000000000000 ) ) ;
#9837=CARTESIAN_POINT ( 'NONE',  ( -29.68486519896224962, 23.49918569563713078, -36.68877005347593467 ) ) ;
#9846=LINE ( 'NONE', #23372, #24173 ) ;
#9851=VECTOR ( 'NONE', #23042, 1000.000000000000000 ) ;
#9872=EDGE_CURVE ( 'NONE', #11743, #31368, #1767, .T. ) ;
#9874=CARTESIAN_POINT ( 'NONE',  ( -35.00000000000000000, -7.062798427011560243, 17.20188834027727154 ) ) ;
#9877=VERTEX_POINT ( 'NONE', #7096 ) ;
#9878=CARTESIAN_POINT ( 'NONE',  ( 37.71145559917817280, 3.353962854566119756, 68.31122994652405112 ) ) ;
#9886=CARTESIAN_POINT ( 'NONE',  ( -8.267476927982267298, 31.47782073335737962, -36.68877005347593467 ) ) ;
#9892=FACE_OUTER_BOUND ( 'NONE', #32212, .T. ) ;
#9897=ORIENTED_EDGE ( 'NONE', *, *, #7162, .F. ) ;
#9901=AXIS2_PLACEMENT_3D ( 'NONE', #5959, #16861, #22178 ) ;
#9908=VECTOR ( 'NONE', #1152, 1000.000000000000000 ) ;
#9916=VECTOR ( 'NONE', #11448, 1000.000000000000000 ) ;
#9919=EDGE_CURVE ( 'NONE', #18651, #17757, #12994, .T. ) ;
#9926=ADVANCED_FACE ( 'NONE', ( #9448 ), #28820, .F. ) ;
#9935=CIRCLE ( 'NONE', #29828, 2.036051781435508801 ) ;
#9940=VERTEX_POINT ( 'NONE', #7269 ) ;
#9950=LINE ( 'NONE', #20294, #34787 ) ;
#9961=ORIENTED_EDGE ( 'NONE', *, *, #25922, .F. ) ;
#9963=CARTESIAN_POINT ( 'NONE',  ( 0.000000000000000000, 3.524919873834583163E-15, 68.31122994652405112 ) ) ;
#9965=EDGE_CURVE ( 'NONE', #2856, #16456, #9782, .T. ) ;
#9966=CARTESIAN_POINT ( 'NONE',  ( 0.000000000000000000, 33.69708579775584667, 49.43553178847298568 ) ) ;
#9969=ORIENTED_EDGE ( 'NONE', *, *, #7545, .T. ) ;
#9970=EDGE_CURVE ( 'NONE', #6016, #14870, #1600, .T. ) ;
#9971=EDGE_CURVE ( 'NONE', #19731, #10833, #12985, .T. ) ;
#9972=LINE ( 'NONE', #29190, #20848 ) ;
#9979=VERTEX_POINT ( 'NONE', #20645 ) ;
#9980=VECTOR ( 'NONE', #609, 1000.000000000000000 ) ;
#9983=LINE ( 'NONE', #15696, #2459 ) ;
#9985=CARTESIAN_POINT ( 'NONE',  ( -15.64512930492131382, -28.53829535743846435, 68.31122994652405112 ) ) ;
#9991=EDGE_CURVE ( 'NONE', #23775, #11101, #20990, .T. ) ;
#9994=( NAMED_UNIT ( * ) SI_UNIT ( $, .STERADIAN. ) SOLID_ANGLE_UNIT ( ) );
#10002=DIRECTION ( 'NONE',  ( 1.000000000000000000, 0.000000000000000000, -0.000000000000000000 ) ) ;
#10005=ORIENTED_EDGE ( 'NONE', *, *, #21025, .T. ) ;
#10008=VERTEX_POINT ( 'NONE', #31158 ) ;
#10017=DIRECTION ( 'NONE',  ( 0.2149704402110236556, 0.9766205557100866574, 0.000000000000000000 ) ) ;
#10027=CARTESIAN_POINT ( 'NONE',  ( -9.978866888775527855, 8.235406450278427215, -67.50000000000000000 ) ) ;
#10035=VECTOR ( 'NONE', #22155, 1000.000000000000000 ) ;
#10038=ORIENTED_EDGE ( 'NONE', *, *, #9483, .T. ) ;
#10055=VERTEX_POINT ( 'NONE', #5647 ) ;
#10058=DIRECTION ( 'NONE',  ( 0.000000000000000000, 1.836970198721029441E-16, -1.000000000000000000 ) ) ;
#10076=CARTESIAN_POINT ( 'NONE',  ( 9.736651044630743712, -33.69708579775584667, 68.31122994652405112 ) ) ;
#10078=VECTOR ( 'NONE', #7379, 1000.000000000000000 ) ;
#10082=ORIENTED_EDGE ( 'NONE', *, *, #16461, .T. ) ;
#10086=AXIS2_PLACEMENT_3D ( 'NONE', #10977, #35024, #30021 ) ;
#10097=VERTEX_POINT ( 'NONE', #13346 ) ;
#10098=ORIENTED_EDGE ( 'NONE', *, *, #14068, .T. ) ;
#10101=CARTESIAN_POINT ( 'NONE',  ( 5.021133111224576062, 14.09580098603202636, -87.50000000000000000 ) ) ;
#10102=VECTOR ( 'NONE', #11081, 1000.000000000000114 ) ;
#10103=CIRCLE ( 'NONE', #6694, 32.54542015209056416 ) ;
#10112=CARTESIAN_POINT ( 'NONE',  ( 5.021133111224265200, -15.68591377522703745, -67.50000000000000000 ) ) ;
#10113=ORIENTED_EDGE ( 'NONE', *, *, #28366, .F. ) ;
#10124=CARTESIAN_POINT ( 'NONE',  ( -23.93921925319781963, 29.33115633223347274, -36.68877005347593467 ) ) ;
#10130=VECTOR ( 'NONE', #17265, 1000.000000000000000 ) ;
#10133=VECTOR ( 'NONE', #17355, 1000.000000000000114 ) ;
#10135=CARTESIAN_POINT ( 'NONE',  ( -5.021133111224782120, 18.16264470403145026, -67.50000000000000000 ) ) ;
#10138=EDGE_LOOP ( 'NONE', ( #22939, #22401, #30702, #27350 ) ) ;
#10141=DIRECTION ( 'NONE',  ( 0.5611870653623822758, 0.8276889981568905652, -0.000000000000000000 ) ) ;
#10142=DIRECTION ( 'NONE',  ( 0.000000000000000000, 1.836970198721029441E-16, -1.000000000000000000 ) ) ;
#10146=DIRECTION ( 'NONE',  ( -0.6876994588534230957, -0.7259954919231310644, 0.000000000000000000 ) ) ;
#10148=FACE_OUTER_BOUND ( 'NONE', #32442, .T. ) ;
#10154=ORIENTED_EDGE ( 'NONE', *, *, #3912, .T. ) ;
#10155=PLANE ( 'NONE',  #11257 ) ;
#10160=DIRECTION ( 'NONE',  ( -0.000000000000000000, 1.836970198721029688E-16, -1.000000000000000000 ) ) ;
#10163=DIRECTION ( 'NONE',  ( -0.000000000000000000, 1.836970198721029934E-16, -1.000000000000000000 ) ) ;
#10164=DIRECTION ( 'NONE',  ( 0.000000000000000000, 0.8958117331950893325, -0.4444337280967883275 ) ) ;
#10170=EDGE_CURVE ( 'NONE', #17629, #18432, #3169, .T. ) ;
#10171=ADVANCED_FACE ( 'NONE', ( #28265 ), #14221, .F. ) ;
#10173=VERTEX_POINT ( 'NONE', #30222 ) ;
#10183=PLANE ( 'NONE',  #17039 ) ;
#10186=VERTEX_POINT ( 'NONE', #863 ) ;
#10189=EDGE_LOOP ( 'NONE', ( #19227, #6936, #33110, #4210, #24558 ) ) ;
#10192=DIRECTION ( 'NONE',  ( -0.000000000000000000, 1.000000000000000000, 0.000000000000000000 ) ) ;
#10194=CARTESIAN_POINT ( 'NONE',  ( 25.76952721012208514, 19.87802405277947315, 68.31122994652405112 ) ) ;
#10198=CARTESIAN_POINT ( 'NONE',  ( -5.614556921127968003, -37.45022281665697506, -36.68877005347593467 ) ) ;
#10203=LINE ( 'NONE', #15552, #29807 ) ;
#10205=VECTOR ( 'NONE', #13391, 1000.000000000000000 ) ;
#10209=DIRECTION ( 'NONE',  ( -1.000000000000000000, 6.792721752314501023E-48, -3.697785493223492838E-32 ) ) ;
#10224=CARTESIAN_POINT ( 'NONE',  ( -21.41424479178920492, -24.50784553716282232, 68.31122994652405112 ) ) ;
#10226=EDGE_LOOP ( 'NONE', ( #6029, #13381, #14983, #8399 ) ) ;
#10228=CARTESIAN_POINT ( 'NONE',  ( -9.978866888775527855, 6.201984591278720593, -87.50000000000000000 ) ) ;
#10230=DIRECTION ( 'NONE',  ( 1.000000000000000000, 0.000000000000000000, -0.000000000000000000 ) ) ;
#10232=DIRECTION ( 'NONE',  ( 0.000000000000000000, -0.5288966977476834419, -0.8486862100397269959 ) ) ;
#10239=DIRECTION ( 'NONE',  ( -1.000000000000000000, -0.000000000000000000, -0.000000000000000000 ) ) ;
#10243=PLANE ( 'NONE',  #34231 ) ;
#10244=DIRECTION ( 'NONE',  ( 0.000000000000000000, 1.836970198721029441E-16, -1.000000000000000000 ) ) ;
#10248=CARTESIAN_POINT ( 'NONE',  ( -35.00000000000000000, -12.29554237047778287, 20.46290632209285576 ) ) ;
#10251=DIRECTION ( 'NONE',  ( 0.000000000000000000, -1.000000000000000000, -2.132064625830773463E-16 ) ) ;
#10255=DIRECTION ( 'NONE',  ( 0.8276889981568904542, 0.5611870653623824978, -0.000000000000000000 ) ) ;
#10263=CARTESIAN_POINT ( 'NONE',  ( 3.235562306570555532E-30, 18.16264470403145026, -67.50000000000000000 ) ) ;
#10265=VECTOR ( 'NONE', #22408, 1000.000000000000114 ) ;
#10285=DIRECTION ( 'NONE',  ( -0.000000000000000000, -0.000000000000000000, -1.000000000000000000 ) ) ;
#10289=DIRECTION ( 'NONE',  ( 0.000000000000000000, -1.000000000000000000, -1.836970198721029934E-16 ) ) ;
#10292=ORIENTED_EDGE ( 'NONE', *, *, #14063, .T. ) ;
#10302=VERTEX_POINT ( 'NONE', #25943 ) ;
#10311=LINE ( 'NONE', #7450, #20385 ) ;
#10312=EDGE_CURVE ( 'NONE', #4500, #27567, #28903, .T. ) ;
#10317=VECTOR ( 'NONE', #10511, 1000.000000000000000 ) ;
#10321=ORIENTED_EDGE ( 'NONE', *, *, #18290, .F. ) ;
#10329=LINE ( 'NONE', #21546, #25714 ) ;
#10336=DIRECTION ( 'NONE',  ( -0.1081190184239433083, 0.9941379571543594862, 1.826201800709962632E-16 ) ) ;
#10337=DIRECTION ( 'NONE',  ( -1.997825486195707906E-17, 0.000000000000000000, 1.000000000000000000 ) ) ;
#10342=VECTOR ( 'NONE', #19330, 999.9999999999998863 ) ;
#10350=ORIENTED_EDGE ( 'NONE', *, *, #30883, .T. ) ;
#10355=DIRECTION ( 'NONE',  ( 0.9476531711828023452, -0.3193015301359802827, -5.865473952658207447E-17 ) ) ;
#10357=ORIENTED_EDGE ( 'NONE', *, *, #4592, .F. ) ;
#10362=LINE ( 'NONE', #32066, #21524 ) ;
#10364=PLANE ( 'NONE',  #5627 ) ;
#10372=AXIS2_PLACEMENT_3D ( 'NONE', #5940, #32647, #10607 ) ;
#10373=DIRECTION ( 'NONE',  ( -0.7621620551276367950, -0.6473862847818272481, 0.000000000000000000 ) ) ;
#10375=EDGE_CURVE ( 'NONE', #15121, #8787, #21124, .T. ) ;
#10391=CIRCLE ( 'NONE', #25173, 32.54542015209057126 ) ;
#10393=ORIENTED_EDGE ( 'NONE', *, *, #557, .F. ) ;
#10396=ORIENTED_EDGE ( 'NONE', *, *, #7358, .T. ) ;
#10398=DIRECTION ( 'NONE',  ( 3.697785493223492838E-32, 1.934419779023891545E-16, -1.000000000000000000 ) ) ;
#10406=CARTESIAN_POINT ( 'NONE',  ( 35.63428259149704758, -12.79065496477508823, 68.31122994652405112 ) ) ;
#10413=LINE ( 'NONE', #27298, #14755 ) ;
#10415=CARTESIAN_POINT ( 'NONE',  ( 5.021133111224473033, 4.168562732279004202, -67.50000000000000000 ) ) ;
#10423=AXIS2_PLACEMENT_3D ( 'NONE', #10740, #18927, #24414 ) ;
#10427=PLANE ( 'NONE',  #26500 ) ;
#10432=DIRECTION ( 'NONE',  ( 0.000000000000000000, -0.000000000000000000, 1.000000000000000000 ) ) ;
#10436=EDGE_CURVE ( 'NONE', #8062, #14584, #12955, .T. ) ;
#10441=DIRECTION ( 'NONE',  ( -0.6051742151937650194, 0.7960930657056437543, 0.000000000000000000 ) ) ;
#10443=FACE_OUTER_BOUND ( 'NONE', #22886, .T. ) ;
#10444=EDGE_CURVE ( 'NONE', #15156, #2086, #15975, .T. ) ;
#10457=LINE ( 'NONE', #21826, #439 ) ;
#10458=DIRECTION ( 'NONE',  ( 0.8854131517428555087, -0.2458337514780907784, -0.3944734685057935675 ) ) ;
#10463=DIRECTION ( 'NONE',  ( -1.000000000000000000, 6.792721752314501023E-48, -3.697785493223492838E-32 ) ) ;
#10473=ORIENTED_EDGE ( 'NONE', *, *, #26035, .T. ) ;
#10476=DIRECTION ( 'NONE',  ( 0.2149704402110243495, 0.9766205557100865464, 0.000000000000000000 ) ) ;
#10479=VERTEX_POINT ( 'NONE', #3472 ) ;
#10481=PLANE ( 'NONE',  #27393 ) ;
#10482=LINE ( 'NONE', #32353, #16827 ) ;
#10484=CIRCLE ( 'NONE', #23562, 32.54542015209055705 ) ;
#10485=ORIENTED_EDGE ( 'NONE', *, *, #5283, .F. ) ;
#10491=CARTESIAN_POINT ( 'NONE',  ( 22.10765473302597073, -16.64466345897532662, -77.50000000000000000 ) ) ;
#10496=EDGE_LOOP ( 'NONE', ( #5054, #9058, #22688, #30759 ) ) ;
#10501=PLANE ( 'NONE',  #4229 ) ;
#10507=LINE ( 'NONE', #26864, #15176 ) ;
#10511=DIRECTION ( 'NONE',  ( 1.000000000000000000, 0.000000000000000000, 0.000000000000000000 ) ) ;
#10514=CARTESIAN_POINT ( 'NONE',  ( 10.17231796313409298, 6.310691531022070144, -77.50000000000000000 ) ) ;
#10517=DIRECTION ( 'NONE',  ( 1.000000000000000000, 0.000000000000000000, -0.000000000000000000 ) ) ;
#10521=CARTESIAN_POINT ( 'NONE',  ( -30.58418286738120884, -22.31615353445078043, -36.68877005347593467 ) ) ;
#10527=AXIS2_PLACEMENT_3D ( 'NONE', #26688, #2293, #13171 ) ;
#10528=EDGE_CURVE ( 'NONE', #24474, #10186, #20428, .T. ) ;
#10533=ORIENTED_EDGE ( 'NONE', *, *, #34633, .F. ) ;
#10534=DIRECTION ( 'NONE',  ( -0.000000000000000000, -1.836970198721029688E-16, 1.000000000000000000 ) ) ;
#10538=ORIENTED_EDGE ( 'NONE', *, *, #28939, .T. ) ;
#10550=AXIS2_PLACEMENT_3D ( 'NONE', #28377, #18064, #12011 ) ;
#10553=DIRECTION ( 'NONE',  ( 0.000000000000000000, 0.000000000000000000, 1.000000000000000000 ) ) ;
#10556=EDGE_LOOP ( 'NONE', ( #950, #7278, #10713, #28471 ) ) ;
#10557=DIRECTION ( 'NONE',  ( 0.000000000000000000, 1.000000000000000000, 0.000000000000000000 ) ) ;
#10568=ORIENTED_EDGE ( 'NONE', *, *, #24560, .T. ) ;
#10570=DIRECTION ( 'NONE',  ( 0.000000000000000000, 1.000000000000000000, 0.000000000000000000 ) ) ;
#10576=DIRECTION ( 'NONE',  ( 0.000000000000000000, 1.836970198721029441E-16, -1.000000000000000000 ) ) ;
#10579=ORIENTED_EDGE ( 'NONE', *, *, #4085, .F. ) ;
#10584=EDGE_LOOP ( 'NONE', ( #28746, #13086, #14609, #19170 ) ) ;
#10595=PLANE ( 'NONE',  #12471 ) ;
#10596=DIRECTION ( 'NONE',  ( 0.000000000000000000, -1.000000000000000000, 0.000000000000000000 ) ) ;
#10607=DIRECTION ( 'NONE',  ( 1.000000000000000000, 0.000000000000000000, 0.000000000000000000 ) ) ;
#10608=ORIENTED_EDGE ( 'NONE', *, *, #24689, .T. ) ;
#10612=DIRECTION ( 'NONE',  ( 0.000000000000000000, 1.000000000000000000, 1.836970198721029688E-16 ) ) ;
#10614=ADVANCED_FACE ( 'NONE', ( #4171 ), #31241, .F. ) ;
#10617=EDGE_CURVE ( 'NONE', #25524, #17023, #27805, .T. ) ;
#10619=ADVANCED_FACE ( 'NONE', ( #30890 ), #10183, .T. ) ;
#10627=ORIENTED_EDGE ( 'NONE', *, *, #18951, .T. ) ;
#10632=ORIENTED_EDGE ( 'NONE', *, *, #8046, .T. ) ;
#10635=DIRECTION ( 'NONE',  ( -0.000000000000000000, -1.836970198721029688E-16, 1.000000000000000000 ) ) ;
#10637=CARTESIAN_POINT ( 'NONE',  ( 18.19419936998244225, -33.21164777187627237, 49.43553178847298568 ) ) ;
#10647=ORIENTED_EDGE ( 'NONE', *, *, #27607, .F. ) ;
#10648=VECTOR ( 'NONE', #34582, 1000.000000000000000 ) ;
#10649=AXIS2_PLACEMENT_3D ( 'NONE', #11429, #19632, #2708 ) ;
#10651=LINE ( 'NONE', #35038, #33130 ) ;
#10652=ORIENTED_EDGE ( 'NONE', *, *, #8582, .F. ) ;
#10659=CARTESIAN_POINT ( 'NONE',  ( 6.857172176539690689, 37.23415287044793587, 68.31122994652405112 ) ) ;
#10665=EDGE_CURVE ( 'NONE', #16556, #18985, #2222, .T. ) ;
#10668=VECTOR ( 'NONE', #7536, 1000.000000000000000 ) ;
#10681=LINE ( 'NONE', #16387, #7046 ) ;
#10682=CARTESIAN_POINT ( 'NONE',  ( 20.89386240318430410, 24.95297350523386726, 68.31122994652405112 ) ) ;
#10685=DIRECTION ( 'NONE',  ( 0.000000000000000000, 1.836970198721029441E-16, -1.000000000000000000 ) ) ;
#10686=ORIENTED_EDGE ( 'NONE', *, *, #20034, .T. ) ;
#10689=DIRECTION ( 'NONE',  ( 0.000000000000000000, 1.836970198721029441E-16, -1.000000000000000000 ) ) ;
#10690=ORIENTED_EDGE ( 'NONE', *, *, #29486, .F. ) ;
#10693=EDGE_CURVE ( 'NONE', #32960, #2754, #3991, .T. ) ;
#10697=ORIENTED_EDGE ( 'NONE', *, *, #12806, .T. ) ;
#10698=DIRECTION ( 'NONE',  ( 0.000000000000000000, 1.836970198721029688E-16, -1.000000000000000000 ) ) ;
#10704=AXIS2_PLACEMENT_3D ( 'NONE', #28296, #19935, #28112 ) ;
#10706=DIRECTION ( 'NONE',  ( -0.9868265225415261410, -0.1617819965527648174, 0.000000000000000000 ) ) ;
#10708=AXIS2_PLACEMENT_3D ( 'NONE', #23201, #1137, #34045 ) ;
#10710=DIRECTION ( 'NONE',  ( 3.697785493223492838E-32, 1.934419779023891545E-16, -1.000000000000000000 ) ) ;
#10713=ORIENTED_EDGE ( 'NONE', *, *, #33727, .T. ) ;
#10714=ORIENTED_EDGE ( 'NONE', *, *, #11587, .F. ) ;
#10722=CARTESIAN_POINT ( 'NONE',  ( 10.17231796313407344, -3.615060903476079890, -77.50000000000000000 ) ) ;
#10723=ORIENTED_EDGE ( 'NONE', *, *, #34139, .T. ) ;
#10731=DIRECTION ( 'NONE',  ( 0.000000000000000000, 1.000000000000000000, 0.000000000000000000 ) ) ;
#10740=CARTESIAN_POINT ( 'NONE',  ( -20.02113311122509032, -13.65249191622732816, -67.50000000000000000 ) ) ;
#10741=LINE ( 'NONE', #18588, #17333 ) ;
#10743=CARTESIAN_POINT ( 'NONE',  ( 37.55078559520313775, -4.831299144296470338, 68.31122994652405112 ) ) ;
#10744=ORIENTED_EDGE ( 'NONE', *, *, #23109, .F. ) ;
#10745=PLANE ( 'NONE',  #4234 ) ;
#10749=ORIENTED_EDGE ( 'NONE', *, *, #7985, .F. ) ;
#10755=ORIENTED_EDGE ( 'NONE', *, *, #34192, .T. ) ;
#10756=FACE_BOUND ( 'NONE', #10969, .T. ) ;
#10761=LINE ( 'NONE', #10930, #9571 ) ;
#10764=ORIENTED_EDGE ( 'NONE', *, *, #22211, .T. ) ;
#10765=CARTESIAN_POINT ( 'NONE',  ( -14.84098889165989377, 28.96462362251111244, 68.31122994652405112 ) ) ;
#10780=DIRECTION ( 'NONE',  ( 0.000000000000000000, 0.000000000000000000, 1.000000000000000000 ) ) ;
#10782=CARTESIAN_POINT ( 'NONE',  ( -5.021133111224679091, 24.02303923978505296, -87.50000000000000000 ) ) ;
#10785=DIRECTION ( 'NONE',  ( 0.000000000000000000, 1.836970198721029441E-16, -1.000000000000000000 ) ) ;
#10790=FACE_OUTER_BOUND ( 'NONE', #32864, .T. ) ;
#10793=ORIENTED_EDGE ( 'NONE', *, *, #1121, .F. ) ;
#10794=CARTESIAN_POINT ( 'NONE',  ( -35.00000000000000000, 16.36947364650383818, 36.69637551990492597 ) ) ;
#10801=DIRECTION ( 'NONE',  ( 0.000000000000000000, 1.000000000000000000, 0.000000000000000000 ) ) ;
#10803=VERTEX_POINT ( 'NONE', #27249 ) ;
#10805=ORIENTED_EDGE ( 'NONE', *, *, #13468, .F. ) ;
#10808=EDGE_CURVE ( 'NONE', #22671, #17531, #2858, .T. ) ;
#10813=CARTESIAN_POINT ( 'NONE',  ( -35.00000000000000000, -7.062798427011537150, -17.20188834027723246 ) ) ;
#10815=EDGE_CURVE ( 'NONE', #2754, #7575, #24565, .T. ) ;
#10816=LINE ( 'NONE', #21662, #27636 ) ;
#10830=DIRECTION ( 'NONE',  ( 0.000000000000000000, 1.836970198721029441E-16, -1.000000000000000000 ) ) ;
#10832=EDGE_LOOP ( 'NONE', ( #19160, #23703, #14227, #23497, #14455, #3733, #14424, #30590 ) ) ;
#10833=VERTEX_POINT ( 'NONE', #20311 ) ;
#10838=DIRECTION ( 'NONE',  ( 0.000000000000000000, 1.836970198721029441E-16, -1.000000000000000000 ) ) ;
#10840=LINE ( 'NONE', #15670, #22981 ) ;
#10841=ORIENTED_EDGE ( 'NONE', *, *, #28427, .F. ) ;
#10846=CARTESIAN_POINT ( 'NONE',  ( 5.021133111224679091, 26.05646109878476580, -87.50000000000000000 ) ) ;
#10847=LINE ( 'NONE', #8831, #31751 ) ;
#10848=VERTEX_POINT ( 'NONE', #17304 ) ;
#10849=ORIENTED_EDGE ( 'NONE', *, *, #24691, .T. ) ;
#10859=EDGE_CURVE ( 'NONE', #3630, #13120, #1945, .T. ) ;
#10862=CARTESIAN_POINT ( 'NONE',  ( 0.000000000000000000, 3.524919873834583163E-15, 68.31122994652405112 ) ) ;
#10866=CARTESIAN_POINT ( 'NONE',  ( -5.021133111225196011, -21.54630831098063481, -87.50000000000000000 ) ) ;
#10873=VERTEX_POINT ( 'NONE', #12829 ) ;
#10876=EDGE_CURVE ( 'NONE', #21448, #4640, #10311, .T. ) ;
#10877=VERTEX_POINT ( 'NONE', #4428 ) ;
#10879=AXIS2_PLACEMENT_3D ( 'NONE', #23328, #1269, #1441 ) ;
#10883=ORIENTED_EDGE ( 'NONE', *, *, #11670, .F. ) ;
#10884=VECTOR ( 'NONE', #7569, 1000.000000000000000 ) ;
#10890=CARTESIAN_POINT ( 'NONE',  ( -37.12776225901827587, -7.411627343331139706, -36.68877005347593467 ) ) ;
#10895=CARTESIAN_POINT ( 'NONE',  ( -20.02113311122488781, 4.168562732279004202, -67.50000000000000000 ) ) ;
#10897=FACE_OUTER_BOUND ( 'NONE', #21948, .T. ) ;
#10901=CARTESIAN_POINT ( 'NONE',  ( -37.12776225901827587, -7.411627343331159246, 68.31122994652405112 ) ) ;
#10909=LINE ( 'NONE', #32430, #32638 ) ;
#10911=AXIS2_PLACEMENT_3D ( 'NONE', #30002, #2242, #21994 ) ;
#10912=LINE ( 'NONE', #10743, #8175 ) ;
#10913=VECTOR ( 'NONE', #20101, 1000.000000000000000 ) ;
#10914=ORIENTED_EDGE ( 'NONE', *, *, #15451, .T. ) ;
#10922=EDGE_CURVE ( 'NONE', #16922, #16320, #20996, .T. ) ;
#10930=CARTESIAN_POINT ( 'NONE',  ( 1.532562817202168137, 32.50931595846690669, 68.31122994652405112 ) ) ;
#10935=VECTOR ( 'NONE', #14169, 1000.000000000000114 ) ;
#10936=DIRECTION ( 'NONE',  ( 0.7259954919231316195, 0.6876994588534225405, 1.263283411590315942E-16 ) ) ;
#10937=EDGE_CURVE ( 'NONE', #29298, #7776, #18347, .T. ) ;
#10943=ORIENTED_EDGE ( 'NONE', *, *, #9337, .T. ) ;
#10946=CARTESIAN_POINT ( 'NONE',  ( -2.791255079241054649, -37.75727539589166071, 68.31122994652405112 ) ) ;
#10951=EDGE_CURVE ( 'NONE', #1165, #14972, #12476, .T. ) ;
#10957=MECHANICAL_DESIGN_GEOMETRIC_PRESENTATION_REPRESENTATION('',(#17237),#31955);
#10959=DIRECTION ( 'NONE',  ( -0.9766205557100866574, -0.2149704402110243218, -3.948942922735925786E-17 ) ) ;
#10963=EDGE_CURVE ( 'NONE', #16672, #12010, #30029, .T. ) ;
#10964=ADVANCED_FACE ( 'NONE', ( #25808 ), #15675, .T. ) ;
#10967=DIRECTION ( 'NONE',  ( 0.000000000000000000, -1.000000000000000000, 0.000000000000000000 ) ) ;
#10968=VERTEX_POINT ( 'NONE', #7274 ) ;
#10969=EDGE_LOOP ( 'NONE', ( #30011, #4591, #31824, #9345 ) ) ;
#10971=DIRECTION ( 'NONE',  ( -1.000000000000000000, 6.792721752314501023E-48, -3.697785493223492838E-32 ) ) ;
#10972=CARTESIAN_POINT ( 'NONE',  ( -35.00000000000000000, -4.831299144296466785, 15.81122994652406355 ) ) ;
#10975=CARTESIAN_POINT ( 'NONE',  ( -37.58721499952019940, -4.609089608337739286, -15.81122994652406355 ) ) ;
#10977=CARTESIAN_POINT ( 'NONE',  ( 30.69344702212033127, -10.82204614554912681, 68.31122994652405112 ) ) ;
#10982=CIRCLE ( 'NONE', #29732, 2.033421858999711951 ) ;
#10985=CARTESIAN_POINT ( 'NONE',  ( 32.81769769215652133, 18.87860345536237006, 68.31122994652405112 ) ) ;
#10993=CARTESIAN_POINT ( 'NONE',  ( 37.55078559520313775, -4.831299144296451686, 49.43553178847298568 ) ) ;
#10997=EDGE_CURVE ( 'NONE', #13120, #30998, #18174, .T. ) ;
#10999=FACE_OUTER_BOUND ( 'NONE', #24591, .T. ) ;
#11005=ORIENTED_EDGE ( 'NONE', *, *, #3471, .F. ) ;
#11009=DIRECTION ( 'NONE',  ( 0.000000000000000000, -0.5288966977476834419, 0.8486862100397269959 ) ) ;
#11017=ORIENTED_EDGE ( 'NONE', *, *, #17549, .F. ) ;
#11018=EDGE_LOOP ( 'NONE', ( #10154, #34627, #2910, #29659 ) ) ;
#11023=CARTESIAN_POINT ( 'NONE',  ( -35.00000000000000000, 16.36947364650383818, -36.69637551990492597 ) ) ;
#11024=ORIENTED_EDGE ( 'NONE', *, *, #2651, .T. ) ;
#11025=ORIENTED_EDGE ( 'NONE', *, *, #3912, .F. ) ;
#11027=VERTEX_POINT ( 'NONE', #13868 ) ;
#11030=CARTESIAN_POINT ( 'NONE',  ( 9.630725478591894984, 36.62364762272931529, -36.68877005347593467 ) ) ;
#11035=AXIS2_PLACEMENT_3D ( 'NONE', #3413, #27800, #33853 ) ;
#11036=AXIS2_PLACEMENT_3D ( 'NONE', #15833, #24332, #19025 ) ;
#11042=CARTESIAN_POINT ( 'NONE',  ( 0.000000000000000000, 3.524919873834583163E-15, 68.31122994652405112 ) ) ;
#11043=DIRECTION ( 'NONE',  ( 0.000000000000000000, 1.000000000000000000, 0.000000000000000000 ) ) ;
#11046=DIRECTION ( 'NONE',  ( 0.6876994588534225405, -0.7259954919231316195, 0.000000000000000000 ) ) ;
#11048=VECTOR ( 'NONE', #14538, 1000.000000000000114 ) ;
#11056=ORIENTED_EDGE ( 'NONE', *, *, #12306, .F. ) ;
#11057=VECTOR ( 'NONE', #10141, 1000.000000000000227 ) ;
#11058=ORIENTED_EDGE ( 'NONE', *, *, #16162, .T. ) ;
#11070=CARTESIAN_POINT ( 'NONE',  ( -23.78520691327551972, 22.21414650552148728, 68.31122994652405112 ) ) ;
#11074=DIRECTION ( 'NONE',  ( -0.5155538571770231782, -0.8568571761675883858, 0.000000000000000000 ) ) ;
#11076=CARTESIAN_POINT ( 'NONE',  ( 6.078604839177343955, 33.69708579775584667, 49.43553178847298568 ) ) ;
#11077=DIRECTION ( 'NONE',  ( 0.000000000000000000, 1.000000000000000000, 0.000000000000000000 ) ) ;
#11081=DIRECTION ( 'NONE',  ( -0.4198891015602644883, -0.9075754196709571175, -0.000000000000000000 ) ) ;
#11083=AXIS2_PLACEMENT_3D ( 'NONE', #7357, #21606, #18249 ) ;
#11084=DIRECTION ( 'NONE',  ( 1.000000000000000000, -0.000000000000000000, -0.000000000000000000 ) ) ;
#11088=DIRECTION ( 'NONE',  ( 1.000000000000000000, 0.000000000000000000, -0.000000000000000000 ) ) ;
#11090=LINE ( 'NONE', #22655, #22500 ) ;
#11092=AXIS2_PLACEMENT_3D ( 'NONE', #15510, #4016, #28248 ) ;
#11100=ORIENTED_EDGE ( 'NONE', *, *, #33626, .T. ) ;
#11101=VERTEX_POINT ( 'NONE', #29889 ) ;
#11105=ORIENTED_EDGE ( 'NONE', *, *, #17944, .T. ) ;
#11111=VECTOR ( 'NONE', #6150, 1000.000000000000000 ) ;
#11117=EDGE_LOOP ( 'NONE', ( #23188, #27557, #9800, #12438, #5691 ) ) ;
#11129=FACE_OUTER_BOUND ( 'NONE', #20695, .T. ) ;
#11131=ADVANCED_FACE ( 'NONE', ( #27383 ), #7811, .F. ) ;
#11143=EDGE_CURVE ( 'NONE', #11027, #5171, #2469, .T. ) ;
#11146=PLANE ( 'NONE',  #10911 ) ;
#11148=LINE ( 'NONE', #8809, #675 ) ;
#11150=EDGE_LOOP ( 'NONE', ( #34054, #16198, #7748, #18117, #33505, #5553, #23477, #12246 ) ) ;
#11159=CIRCLE ( 'NONE', #8296, 32.54542015209057126 ) ;
#11165=LINE ( 'NONE', #29845, #34544 ) ;
#11172=CARTESIAN_POINT ( 'NONE',  ( -1.307386931792819285, 32.51914993179678959, 68.31122994652405112 ) ) ;
#11175=LINE ( 'NONE', #16881, #20620 ) ;
#11177=EDGE_CURVE ( 'NONE', #16061, #21875, #12988, .T. ) ;
#11178=DIRECTION ( 'NONE',  ( 0.000000000000000000, 1.836970198721029441E-16, -1.000000000000000000 ) ) ;
#11181=FACE_OUTER_BOUND ( 'NONE', #18906, .T. ) ;
#11188=LINE ( 'NONE', #3158, #24550 ) ;
#11190=VERTEX_POINT ( 'NONE', #6548 ) ;
#11193=CARTESIAN_POINT ( 'NONE',  ( -9.978866888775527855, 6.201984591278717041, -67.50000000000000000 ) ) ;
#11197=DIRECTION ( 'NONE',  ( 0.000000000000000000, 1.836970198721029441E-16, -1.000000000000000000 ) ) ;
#11199=VERTEX_POINT ( 'NONE', #3702 ) ;
#11205=CARTESIAN_POINT ( 'NONE',  ( 0.000000000000000000, 3.524919873834583163E-15, 68.31122994652405112 ) ) ;
#11206=VECTOR ( 'NONE', #35070, 1000.000000000000114 ) ;
#11212=EDGE_CURVE ( 'NONE', #3836, #12737, #27560, .T. ) ;
#11216=ORIENTED_EDGE ( 'NONE', *, *, #5181, .T. ) ;
#11221=VERTEX_POINT ( 'NONE', #3176 ) ;
#11230=AXIS2_PLACEMENT_3D ( 'NONE', #24060, #12889, #10373 ) ;
#11241=CARTESIAN_POINT ( 'NONE',  ( 26.04754872656010178, -19.51229300245305964, 49.43553178847298568 ) ) ;
#11244=DIRECTION ( 'NONE',  ( 0.3203292411224474279, -0.8039657716618124894, -0.5010271602200255803 ) ) ;
#11245=VECTOR ( 'NONE', #29834, 1000.000000000000000 ) ;
#11249=CARTESIAN_POINT ( 'NONE',  ( -20.72055270933793736, 25.09707290294328885, 68.31122994652405112 ) ) ;
#11251=DIRECTION ( 'NONE',  ( -0.000000000000000000, -0.000000000000000000, 1.000000000000000000 ) ) ;
#11252=DIRECTION ( 'NONE',  ( 1.000000000000000000, 0.000000000000000000, 0.000000000000000000 ) ) ;
#11256=DIRECTION ( 'NONE',  ( -1.000000000000000000, 6.792721752314501023E-48, -3.697785493223492838E-32 ) ) ;
#11257=AXIS2_PLACEMENT_3D ( 'NONE', #21014, #10698, #8365 ) ;
#11262=EDGE_CURVE ( 'NONE', #29040, #13030, #3822, .T. ) ;
#11269=CARTESIAN_POINT ( 'NONE',  ( 0.000000000000000000, 16.36473396058513075, -36.68877005347593467 ) ) ;
#11270=EDGE_CURVE ( 'NONE', #7307, #29615, #18142, .T. ) ;
#11273=EDGE_LOOP ( 'NONE', ( #12967, #28642, #30383, #17086 ) ) ;
#11274=DIRECTION ( 'NONE',  ( -0.2149704402110247936, -0.9766205557100865464, -1.794022856297800030E-16 ) ) ;
#11278=ORIENTED_EDGE ( 'NONE', *, *, #15682, .F. ) ;
#11283=ORIENTED_EDGE ( 'NONE', *, *, #19340, .T. ) ;
#11291=ORIENTED_EDGE ( 'NONE', *, *, #32094, .F. ) ;
#11299=AXIS2_PLACEMENT_3D ( 'NONE', #7276, #34701, #1606 ) ;
#11302=LINE ( 'NONE', #32643, #10035 ) ;
#11306=FACE_OUTER_BOUND ( 'NONE', #21612, .T. ) ;
#11307=ORIENTED_EDGE ( 'NONE', *, *, #30229, .F. ) ;
#11309=EDGE_CURVE ( 'NONE', #34117, #30456, #28444, .T. ) ;
#11311=DIRECTION ( 'NONE',  ( -0.000000000000000000, 1.836970198721029934E-16, -1.000000000000000000 ) ) ;
#11314=DIRECTION ( 'NONE',  ( -0.9075754196709575616, 0.4198891015602634891, -0.000000000000000000 ) ) ;
#11323=VERTEX_POINT ( 'NONE', #23449 ) ;
#11328=CARTESIAN_POINT ( 'NONE',  ( -35.71762877834949990, -12.58147180936565235, -20.64109601603115607 ) ) ;
#11335=LINE ( 'NONE', #10972, #26742 ) ;
#11336=VERTEX_POINT ( 'NONE', #17616 ) ;
#11342=FACE_OUTER_BOUND ( 'NONE', #28090, .T. ) ;
#11349=FACE_OUTER_BOUND ( 'NONE', #7305, .T. ) ;
#11351=ORIENTED_EDGE ( 'NONE', *, *, #8544, .T. ) ;
#11353=ADVANCED_FACE ( 'NONE', ( #26820 ), #16159, .F. ) ;
#11360=CARTESIAN_POINT ( 'NONE',  ( 18.19419936998243870, -33.21164777187627237, 68.31122994652405112 ) ) ;
#11364=CARTESIAN_POINT ( 'NONE',  ( 30.98406361983693103, 9.959526819984921175, 68.31122994652405112 ) ) ;
#11367=EDGE_CURVE ( 'NONE', #29615, #1937, #17515, .T. ) ;
#11370=CARTESIAN_POINT ( 'NONE',  ( 11.62236370382047745, -30.39942490923500884, 68.31122994652405112 ) ) ;
#11393=CARTESIAN_POINT ( 'NONE',  ( -35.71762877834949990, -12.58147180936565945, 20.64109601603116673 ) ) ;
#11394=DIRECTION ( 'NONE',  ( 0.3193015301359797276, 0.9476531711828024562, -0.000000000000000000 ) ) ;
#11395=EDGE_CURVE ( 'NONE', #3900, #18597, #5095, .T. ) ;
#11396=EDGE_LOOP ( 'NONE', ( #24088, #21088, #29111, #15765 ) ) ;
#11403=EDGE_CURVE ( 'NONE', #4890, #27831, #34845, .T. ) ;
#11405=EDGE_CURVE ( 'NONE', #1890, #12838, #10457, .T. ) ;
#11408=ORIENTED_EDGE ( 'NONE', *, *, #12367, .F. ) ;
#11410=LINE ( 'NONE', #732, #27553 ) ;
#11418=CARTESIAN_POINT ( 'NONE',  ( 5.021133111224679091, 28.08988295778447508, -87.50000000000000000 ) ) ;
#11420=CARTESIAN_POINT ( 'NONE',  ( -17.07420202168509604, 33.79163469797341435, 68.31122994652405112 ) ) ;
#11424=CARTESIAN_POINT ( 'NONE',  ( -31.87924797510910935, -6.551177101682126747, 68.31122994652405112 ) ) ;
#11425=DIRECTION ( 'NONE',  ( 0.000000000000000000, 1.836970198721029934E-16, -1.000000000000000000 ) ) ;
#11428=VECTOR ( 'NONE', #23411, 1000.000000000000114 ) ;
#11429=CARTESIAN_POINT ( 'NONE',  ( 0.000000000000000000, 6.992329373473909019E-15, 49.43553178847298568 ) ) ;
#11432=CARTESIAN_POINT ( 'NONE',  ( 29.63313772848249883, -13.45665341906702572, 68.31122994652405112 ) ) ;
#11437=LINE ( 'NONE', #16445, #15621 ) ;
#11438=DIRECTION ( 'NONE',  ( 0.000000000000000000, 0.000000000000000000, 1.000000000000000000 ) ) ;
#11439=ORIENTED_EDGE ( 'NONE', *, *, #31763, .F. ) ;
#11443=CIRCLE ( 'NONE', #18826, 32.54542015209057126 ) ;
#11446=ADVANCED_FACE ( 'NONE', ( #29847 ), #13649, .F. ) ;
#11447=VERTEX_POINT ( 'NONE', #15816 ) ;
#11448=DIRECTION ( 'NONE',  ( 0.000000000000000000, -0.8486862100397269959, 0.5288966977476833309 ) ) ;
#11456=CARTESIAN_POINT ( 'NONE',  ( 35.63428259149704758, -12.79065496477508823, 68.31122994652405112 ) ) ;
#11461=APPLICATION_CONTEXT ( 'automotive_design' ) ;
#11470=LINE ( 'NONE', #5409, #19682 ) ;
#11476=VECTOR ( 'NONE', #16886, 1000.000000000000000 ) ;
#11479=CARTESIAN_POINT ( 'NONE',  ( -2.791255079241054649, -37.75727539589163939, -36.68877005347593467 ) ) ;
#11482=DIRECTION ( 'NONE',  ( 0.2675283385292215321, 0.9635499925192227977, 0.000000000000000000 ) ) ;
#11484=VERTEX_POINT ( 'NONE', #27168 ) ;
#11485=FACE_OUTER_BOUND ( 'NONE', #2603, .T. ) ;
#11491=LINE ( 'NONE', #24994, #23382 ) ;
#11492=ORIENTED_EDGE ( 'NONE', *, *, #33441, .T. ) ;
#11498=CARTESIAN_POINT ( 'NONE',  ( 28.11866956577617316, 16.38733641342590985, 68.31122994652405112 ) ) ;
#11502=CARTESIAN_POINT ( 'NONE',  ( 30.45781707305797426, -22.50252913745434569, 49.43553178847298568 ) ) ;
#11510=ORIENTED_EDGE ( 'NONE', *, *, #15120, .F. ) ;
#11514=DIRECTION ( 'NONE',  ( 0.000000000000000000, -1.000000000000000000, -2.132064625830773463E-16 ) ) ;
#11516=CARTESIAN_POINT ( 'NONE',  ( 23.93847777447631131, 22.04889236939138186, 68.31122994652405112 ) ) ;
#11526=AXIS2_PLACEMENT_3D ( 'NONE', #8533, #14426, #33448 ) ;
#11533=EDGE_CURVE ( 'NONE', #12217, #3404, #16870, .T. ) ;
#11534=EDGE_CURVE ( 'NONE', #30543, #32722, #19706, .T. ) ;
#11543=ORIENTED_EDGE ( 'NONE', *, *, #34671, .T. ) ;
#11544=DIRECTION ( 'NONE',  ( 0.000000000000000000, 0.000000000000000000, 1.000000000000000000 ) ) ;
#11546=VECTOR ( 'NONE', #15603, 1000.000000000000000 ) ;
#11553=ADVANCED_FACE ( 'NONE', ( #30191 ), #25551, .F. ) ;
#11558=ADVANCED_FACE ( 'NONE', ( #33213 ), #8480, .T. ) ;
#11561=ORIENTED_EDGE ( 'NONE', *, *, #34127, .F. ) ;
#11565=CARTESIAN_POINT ( 'NONE',  ( -37.69926482250235722, 3.578808500140874926, -16.17202516343390428 ) ) ;
#11566=CARTESIAN_POINT ( 'NONE',  ( 22.10765473302597073, -16.64466345897532307, -87.50000000000000000 ) ) ;
#11567=ORIENTED_EDGE ( 'NONE', *, *, #14621, .F. ) ;
#11569=DIRECTION ( 'NONE',  ( -0.000000000000000000, 1.836970198721029934E-16, -1.000000000000000000 ) ) ;
#11572=CARTESIAN_POINT ( 'NONE',  ( 0.000000000000000000, -33.69708579775584667, 49.43553178847298568 ) ) ;
#11575=LINE ( 'NONE', #19589, #16624 ) ;
#11579=LINE ( 'NONE', #19767, #8871 ) ;
#11585=ADVANCED_FACE ( 'NONE', ( #22187 ), #17046, .F. ) ;
#11587=EDGE_CURVE ( 'NONE', #17023, #16061, #3484, .T. ) ;
#11592=ORIENTED_EDGE ( 'NONE', *, *, #26478, .F. ) ;
#11594=AXIS2_PLACEMENT_3D ( 'NONE', #28145, #17134, #6414 ) ;
#11598=CARTESIAN_POINT ( 'NONE',  ( -9.410814080250917257, 36.67205378194064735, 68.31122994652405112 ) ) ;
#11603=VECTOR ( 'NONE', #20674, 1000.000000000000114 ) ;
#11605=ORIENTED_EDGE ( 'NONE', *, *, #3030, .T. ) ;
#11607=DIRECTION ( 'NONE',  ( -1.000000000000000000, 6.792721752314501023E-48, -3.697785493223492838E-32 ) ) ;
#11613=DIRECTION ( 'NONE',  ( 3.697785493223492838E-32, 1.934419779023891545E-16, -1.000000000000000000 ) ) ;
#11625=LINE ( 'NONE', #6077, #28663 ) ;
#11626=ORIENTED_EDGE ( 'NONE', *, *, #29825, .F. ) ;
#11629=VECTOR ( 'NONE', #1263, 1000.000000000000000 ) ;
#11635=VERTEX_POINT ( 'NONE', #20233 ) ;
#11640=CARTESIAN_POINT ( 'NONE',  ( -11.83261234297099662, -30.31820670846265742, -36.68877005347593467 ) ) ;
#11644=DIRECTION ( 'NONE',  ( 0.000000000000000000, 1.836970198721029441E-16, -1.000000000000000000 ) ) ;
#11645=CARTESIAN_POINT ( 'NONE',  ( 22.89764159710611224, 15.60017778382161246, -77.50000000000000000 ) ) ;
#11650=CIRCLE ( 'NONE', #15059, 2.033421858999710619 ) ;
#11654=ORIENTED_EDGE ( 'NONE', *, *, #21535, .T. ) ;
#11661=LINE ( 'NONE', #8978, #19649 ) ;
#11662=LINE ( 'NONE', #19674, #24552 ) ;
#11663=ADVANCED_FACE ( 'NONE', ( #29096 ), #12562, .T. ) ;
#11664=CARTESIAN_POINT ( 'NONE',  ( -5.038454199367317976, -32.15304576796694391, -36.68877005347593467 ) ) ;
#11666=CARTESIAN_POINT ( 'NONE',  ( -36.80830595996284416, 8.862931941313773265, 68.31122994652405112 ) ) ;
#11667=ADVANCED_FACE ( 'NONE', ( #31248 ), #15069, .F. ) ;
#11670=EDGE_CURVE ( 'NONE', #33546, #21129, #12396, .T. ) ;
#11672=CARTESIAN_POINT ( 'NONE',  ( 26.97014235612466493, -26.57093094961043889, 68.31122994652405112 ) ) ;
#11676=DIRECTION ( 'NONE',  ( 3.697785493223492838E-32, 1.934419779023891545E-16, -1.000000000000000000 ) ) ;
#11680=ORIENTED_EDGE ( 'NONE', *, *, #19938, .T. ) ;
#11681=VECTOR ( 'NONE', #28254, 1000.000000000000000 ) ;
#11684=ORIENTED_EDGE ( 'NONE', *, *, #28330, .T. ) ;
#11689=CARTESIAN_POINT ( 'NONE',  ( -40.71667869272602758, -14.57327534360751109, 21.88237730393305469 ) ) ;
#11697=CIRCLE ( 'NONE', #30438, 2.033421858999711951 ) ;
#11700=ORIENTED_EDGE ( 'NONE', *, *, #16988, .F. ) ;
#11704=EDGE_CURVE ( 'NONE', #1937, #33546, #18256, .T. ) ;
#11706=VERTEX_POINT ( 'NONE', #17745 ) ;
#11709=ADVANCED_FACE ( 'NONE', ( #26249 ), #20747, .T. ) ;
#11712=AXIS2_PLACEMENT_3D ( 'NONE', #7298, #28678, #22994 ) ;
#11713=EDGE_CURVE ( 'NONE', #31774, #29370, #1598, .T. ) ;
#11725=AXIS2_PLACEMENT_3D ( 'NONE', #9280, #6417, #31811 ) ;
#11734=ORIENTED_EDGE ( 'NONE', *, *, #21101, .F. ) ;
#11737=CIRCLE ( 'NONE', #31610, 32.54542015209056416 ) ;
#11741=ORIENTED_EDGE ( 'NONE', *, *, #22707, .T. ) ;
#11743=VERTEX_POINT ( 'NONE', #14897 ) ;
#11744=DIRECTION ( 'NONE',  ( 0.000000000000000000, 1.000000000000000000, 0.000000000000000000 ) ) ;
#11745=ORIENTED_EDGE ( 'NONE', *, *, #21079, .T. ) ;
#11751=VECTOR ( 'NONE', #25462, 1000.000000000000000 ) ;
#11760=DIRECTION ( 'NONE',  ( -0.9289767198167909745, 0.3701381553399156199, 0.000000000000000000 ) ) ;
#11761=EDGE_CURVE ( 'NONE', #20902, #22067, #25730, .T. ) ;
#11766=VECTOR ( 'NONE', #11314, 1000.000000000000114 ) ;
#11771=ORIENTED_EDGE ( 'NONE', *, *, #24983, .T. ) ;
#11774=CARTESIAN_POINT ( 'NONE',  ( -35.00000000000000000, -38.34433698000722046, 36.69637551990492597 ) ) ;
#11775=CIRCLE ( 'NONE', #2654, 32.54542015209056416 ) ;
#11793=VERTEX_POINT ( 'NONE', #21265 ) ;
#11802=FACE_OUTER_BOUND ( 'NONE', #14029, .T. ) ;
#11803=CARTESIAN_POINT ( 'NONE',  ( -9.410814080250917257, 36.67205378194064735, 68.31122994652405112 ) ) ;
#11806=AXIS2_PLACEMENT_3D ( 'NONE', #20669, #18360, #21187 ) ;
#11807=EDGE_CURVE ( 'NONE', #27734, #34696, #13608, .T. ) ;
#11812=DIRECTION ( 'NONE',  ( -0.1617819965527650672, 0.9868265225415261410, 1.812770913216289798E-16 ) ) ;
#11813=LINE ( 'NONE', #28164, #32483 ) ;
#11817=VECTOR ( 'NONE', #16507, 1000.000000000000000 ) ;
#11822=ORIENTED_EDGE ( 'NONE', *, *, #17297, .F. ) ;
#11825=ADVANCED_FACE ( 'NONE', ( #18612 ), #18436, .T. ) ;
#11828=ORIENTED_EDGE ( 'NONE', *, *, #31016, .F. ) ;
#11830=DIRECTION ( 'NONE',  ( -0.05413890858541763051, -0.9985334138511239299, -1.834276123671687319E-16 ) ) ;
#11834=PLANE ( 'NONE',  #26013 ) ;
#11837=CARTESIAN_POINT ( 'NONE',  ( -41.91891556802573859, 16.36473396058513785, -36.68877005347594178 ) ) ;
#11840=VECTOR ( 'NONE', #4515, 1000.000000000000000 ) ;
#11845=DIRECTION ( 'NONE',  ( 0.8568571761675904952, -0.5155538571770196254, -0.000000000000000000 ) ) ;
#11846=DIRECTION ( 'NONE',  ( 0.000000000000000000, 1.836970198721029688E-16, -1.000000000000000000 ) ) ;
#11852=CARTESIAN_POINT ( 'NONE',  ( 0.000000000000000000, -32.54542015209057126, 87.50000000000000000 ) ) ;
#11860=CIRCLE ( 'NONE', #30596, 32.54542015209057126 ) ;
#11864=ORIENTED_EDGE ( 'NONE', *, *, #32930, .F. ) ;
#11877=ADVANCED_FACE ( 'NONE', ( #75 ), #21441, .F. ) ;
#11882=FACE_OUTER_BOUND ( 'NONE', #25927, .T. ) ;
#11883=ORIENTED_EDGE ( 'NONE', *, *, #8772, .F. ) ;
#11897=CARTESIAN_POINT ( 'NONE',  ( -29.34345171400087793, 14.07715221144536777, -36.68877005347593467 ) ) ;
#11904=PLANE ( 'NONE',  #1918 ) ;
#11905=EDGE_CURVE ( 'NONE', #20048, #3630, #22684, .T. ) ;
#11907=DIRECTION ( 'NONE',  ( 0.000000000000000000, 1.836970198721029441E-16, -1.000000000000000000 ) ) ;
#11910=ORIENTED_EDGE ( 'NONE', *, *, #10808, .F. ) ;
#11917=FACE_OUTER_BOUND ( 'NONE', #11117, .T. ) ;
#11929=ORIENTED_EDGE ( 'NONE', *, *, #28520, .T. ) ;
#11935=CARTESIAN_POINT ( 'NONE',  ( 31.83311414508813897, -6.771795677801495827, 68.31122994652405112 ) ) ;
#11947=LINE ( 'NONE', #20307, #584 ) ;
#11949=ORIENTED_EDGE ( 'NONE', *, *, #2823, .F. ) ;
#11952=FACE_OUTER_BOUND ( 'NONE', #5913, .T. ) ;
#11961=ADVANCED_FACE ( 'NONE', ( #5925 ), #19840, .F. ) ;
#11962=DIRECTION ( 'NONE',  ( 0.5155538571770216238, -0.8568571761675893850, 0.000000000000000000 ) ) ;
#11963=PLANE ( 'NONE',  #4430 ) ;
#11966=ORIENTED_EDGE ( 'NONE', *, *, #33174, .T. ) ;
#11967=CYLINDRICAL_SURFACE ( 'NONE', #11725, 2.033421858999711507 ) ;
#11968=CARTESIAN_POINT ( 'NONE',  ( 3.235562306570555532E-30, -11.61907005722761177, -87.50000000000000000 ) ) ;
#11975=DIRECTION ( 'NONE',  ( -0.3193015301359803382, -0.9476531711828023452, 0.000000000000000000 ) ) ;
#11978=ORIENTED_EDGE ( 'NONE', *, *, #16537, .F. ) ;
#11979=DIRECTION ( 'NONE',  ( -0.9868265225415260300, -0.1617819965527650394, 0.000000000000000000 ) ) ;
#11981=EDGE_CURVE ( 'NONE', #18461, #32452, #16468, .T. ) ;
#11982=ORIENTED_EDGE ( 'NONE', *, *, #5654, .T. ) ;
#11986=VECTOR ( 'NONE', #9591, 1000.000000000000000 ) ;
#11990=ORIENTED_EDGE ( 'NONE', *, *, #28529, .F. ) ;
#11991=ORIENTED_EDGE ( 'NONE', *, *, #10170, .F. ) ;
#11992=DIRECTION ( 'NONE',  ( 0.000000000000000000, 1.000000000000000000, 1.836970198721029688E-16 ) ) ;
#11998=EDGE_CURVE ( 'NONE', #8062, #13770, #24972, .T. ) ;
#11999=ADVANCED_FACE ( 'NONE', ( #8781, #19664 ), #11834, .F. ) ;
#12002=CARTESIAN_POINT ( 'NONE',  ( -1.307386931792819285, 32.51914993179681090, -36.68877005347593467 ) ) ;
#12010=VERTEX_POINT ( 'NONE', #13968 ) ;
#12011=DIRECTION ( 'NONE',  ( 1.000000000000000000, 0.000000000000000000, 0.000000000000000000 ) ) ;
#12017=VECTOR ( 'NONE', #32943, 1000.000000000000000 ) ;
#12028=ORIENTED_EDGE ( 'NONE', *, *, #7545, .F. ) ;
#12029=CARTESIAN_POINT ( 'NONE',  ( 0.000000000000000000, 3.524919873834583163E-15, 68.31122994652405112 ) ) ;
#12032=ORIENTED_EDGE ( 'NONE', *, *, #26717, .T. ) ;
#12035=VERTEX_POINT ( 'NONE', #7149 ) ;
#12044=FACE_OUTER_BOUND ( 'NONE', #23646, .T. ) ;
#12047=AXIS2_PLACEMENT_3D ( 'NONE', #15517, #10163, #23857 ) ;
#12050=AXIS2_PLACEMENT_3D ( 'NONE', #3460, #8462, #13990 ) ;
#12064=LINE ( 'NONE', #7037, #28030 ) ;
#12068=EDGE_CURVE ( 'NONE', #14410, #594, #15368, .T. ) ;
#12072=ORIENTED_EDGE ( 'NONE', *, *, #25302, .T. ) ;
#12078=ORIENTED_EDGE ( 'NONE', *, *, #6797, .T. ) ;
#12087=ORIENTED_EDGE ( 'NONE', *, *, #28719, .T. ) ;
#12099=LINE ( 'NONE', #22938, #7871 ) ;
#12101=DIRECTION ( 'NONE',  ( 0.000000000000000000, 1.000000000000000000, 0.000000000000000000 ) ) ;
#12103=ORIENTED_EDGE ( 'NONE', *, *, #7289, .T. ) ;
#12108=PLANE ( 'NONE',  #10704 ) ;
#12115=CARTESIAN_POINT ( 'NONE',  ( -45.00000000000000000, 16.36947364650383818, -36.69637551990492597 ) ) ;
#12117=EDGE_CURVE ( 'NONE', #29230, #25215, #7268, .T. ) ;
#12124=VERTEX_POINT ( 'NONE', #6806 ) ;
#12129=CARTESIAN_POINT ( 'NONE',  ( 1.532562817202168137, 37.83772838912469894, 68.31122994652405112 ) ) ;
#12135=VERTEX_POINT ( 'NONE', #6633 ) ;
#12138=FACE_OUTER_BOUND ( 'NONE', #22003, .T. ) ;
#12142=CIRCLE ( 'NONE', #24602, 32.54542015209057126 ) ;
#12148=ADVANCED_FACE ( 'NONE', ( #18052 ), #28877, .F. ) ;
#12151=DIRECTION ( 'NONE',  ( -0.000000000000000000, 1.836970198721029934E-16, -1.000000000000000000 ) ) ;
#12155=ORIENTED_EDGE ( 'NONE', *, *, #27360, .T. ) ;
#12160=VECTOR ( 'NONE', #24344, 1000.000000000000227 ) ;
#12163=EDGE_CURVE ( 'NONE', #1041, #24110, #25476, .T. ) ;
#12175=ORIENTED_EDGE ( 'NONE', *, *, #5822, .F. ) ;
#12176=CARTESIAN_POINT ( 'NONE',  ( 0.000000000000000000, 2.281310696040539424E-14, -36.68877005347592757 ) ) ;
#12178=ORIENTED_EDGE ( 'NONE', *, *, #13235, .F. ) ;
#12183=DIRECTION ( 'NONE',  ( 0.000000000000000000, -1.000000000000000000, -1.836970198721029934E-16 ) ) ;
#12191=DIRECTION ( 'NONE',  ( -0.9289767198167914186, -0.3701381553399144542, 0.000000000000000000 ) ) ;
#12202=VERTEX_POINT ( 'NONE', #32104 ) ;
#12205=DIRECTION ( 'NONE',  ( -0.000000000000000000, -0.000000000000000000, -1.000000000000000000 ) ) ;
#12206=AXIS2_PLACEMENT_3D ( 'NONE', #17999, #6441, #1123 ) ;
#12211=FACE_OUTER_BOUND ( 'NONE', #33984, .T. ) ;
#12212=ORIENTED_EDGE ( 'NONE', *, *, #21973, .T. ) ;
#12216=VERTEX_POINT ( 'NONE', #7502 ) ;
#12217=VERTEX_POINT ( 'NONE', #30 ) ;
#12218=LINE ( 'NONE', #20559, #5898 ) ;
#12229=DIRECTION ( 'NONE',  ( 0.000000000000000000, 1.836970198721029441E-16, -1.000000000000000000 ) ) ;
#12234=ADVANCED_FACE ( 'NONE', ( #21576 ), #4646, .F. ) ;
#12238=PLANE ( 'NONE',  #6547 ) ;
#12239=EDGE_CURVE ( 'NONE', #19542, #26155, #31882, .T. ) ;
#12241=LINE ( 'NONE', #1368, #18924 ) ;
#12244=EDGE_CURVE ( 'NONE', #736, #6259, #11860, .T. ) ;
#12246=ORIENTED_EDGE ( 'NONE', *, *, #33580, .F. ) ;
#12258=LINE ( 'NONE', #9402, #5339 ) ;
#12272=EDGE_CURVE ( 'NONE', #22594, #23988, #10362, .T. ) ;
#12273=DIRECTION ( 'NONE',  ( 0.000000000000000000, 1.000000000000000000, 1.934419779023891545E-16 ) ) ;
#12275=VECTOR ( 'NONE', #9569, 1000.000000000000000 ) ;
#12278=ORIENTED_EDGE ( 'NONE', *, *, #3654, .F. ) ;
#12281=VERTEX_POINT ( 'NONE', #18576 ) ;
#12285=FACE_OUTER_BOUND ( 'NONE', #24865, .T. ) ;
#12286=DIRECTION ( 'NONE',  ( -0.2149704402110242940, 0.9766205557100865464, 0.000000000000000000 ) ) ;
#12291=CARTESIAN_POINT ( 'NONE',  ( 29.63313772848251659, -13.45665341906703460, 49.43553178847298568 ) ) ;
#12292=VECTOR ( 'NONE', #32985, 1000.000000000000000 ) ;
#12298=DIRECTION ( 'NONE',  ( 0.000000000000000000, 1.836970198721029441E-16, -1.000000000000000000 ) ) ;
#12306=EDGE_CURVE ( 'NONE', #20173, #29194, #21400, .T. ) ;
#12309=VERTEX_POINT ( 'NONE', #22766 ) ;
#12313=VECTOR ( 'NONE', #9193, 1000.000000000000114 ) ;
#12315=DIRECTION ( 'NONE',  ( 0.9985334138511239299, 0.05413890858541755419, 0.000000000000000000 ) ) ;
#12323=DIRECTION ( 'NONE',  ( -0.9289767198167914186, -0.3701381553399144542, 0.000000000000000000 ) ) ;
#12342=EDGE_LOOP ( 'NONE', ( #1249, #7484, #9165, #6097 ) ) ;
#12343=LINE ( 'NONE', #30677, #33414 ) ;
#12349=ADVANCED_FACE ( 'NONE', ( #31131 ), #3047, .F. ) ;
#12353=DIRECTION ( 'NONE',  ( 0.000000000000000000, 1.836970198721029441E-16, -1.000000000000000000 ) ) ;
#12363=ORIENTED_EDGE ( 'NONE', *, *, #10876, .T. ) ;
#12365=CARTESIAN_POINT ( 'NONE',  ( -45.00000000000000000, -38.34433698000722046, -36.69637551990492597 ) ) ;
#12366=LINE ( 'NONE', #6115, #197 ) ;
#12367=EDGE_CURVE ( 'NONE', #31704, #31010, #24760, .T. ) ;
#12373=LINE ( 'NONE', #11852, #2486 ) ;
#12374=CARTESIAN_POINT ( 'NONE',  ( -5.021133111225196011, -23.57973016998034765, -67.50000000000000000 ) ) ;
#12376=AXIS2_PLACEMENT_3D ( 'NONE', #22894, #33389, #9014 ) ;
#12377=ORIENTED_EDGE ( 'NONE', *, *, #10375, .F. ) ;
#12380=ORIENTED_EDGE ( 'NONE', *, *, #24823, .T. ) ;
#12384=ORIENTED_EDGE ( 'NONE', *, *, #30025, .T. ) ;
#12386=EDGE_LOOP ( 'NONE', ( #25247, #30983, #7005, #29717 ) ) ;
#12387=ORIENTED_EDGE ( 'NONE', *, *, #25659, .T. ) ;
#12394=CARTESIAN_POINT ( 'NONE',  ( 29.82459402470852083, -33.69708579775584667, -49.43553178847298568 ) ) ;
#12396=LINE ( 'NONE', #4690, #11840 ) ;
#12405=CARTESIAN_POINT ( 'NONE',  ( 10.96230482721425403, -14.55883922869198344, -77.50000000000000000 ) ) ;
#12424=ORIENTED_EDGE ( 'NONE', *, *, #17654, .F. ) ;
#12432=LINE ( 'NONE', #15273, #34339 ) ;
#12434=DIRECTION ( 'NONE',  ( 0.000000000000000000, -1.000000000000000000, -2.132064625830773463E-16 ) ) ;
#12436=LINE ( 'NONE', #31454, #6651 ) ;
#12438=ORIENTED_EDGE ( 'NONE', *, *, #30913, .F. ) ;
#12441=ORIENTED_EDGE ( 'NONE', *, *, #4284, .F. ) ;
#12447=EDGE_CURVE ( 'NONE', #2115, #3468, #12099, .T. ) ;
#12450=ORIENTED_EDGE ( 'NONE', *, *, #28120, .F. ) ;
#12452=AXIS2_PLACEMENT_3D ( 'NONE', #20106, #9062, #12101 ) ;
#12454=CIRCLE ( 'NONE', #13586, 32.54542015209055705 ) ;
#12459=AXIS2_PLACEMENT_3D ( 'NONE', #14927, #20778, #12434 ) ;
#12464=VECTOR ( 'NONE', #24321, 1000.000000000000114 ) ;
#12467=ORIENTED_EDGE ( 'NONE', *, *, #19261, .F. ) ;
#12469=ORIENTED_EDGE ( 'NONE', *, *, #3225, .T. ) ;
#12471=AXIS2_PLACEMENT_3D ( 'NONE', #24271, #10232, #15583 ) ;
#12473=ORIENTED_EDGE ( 'NONE', *, *, #28791, .F. ) ;
#12474=ADVANCED_FACE ( 'NONE', ( #2096 ), #15460, .F. ) ;
#12476=LINE ( 'NONE', #29184, #32863 ) ;
#12479=ORIENTED_EDGE ( 'NONE', *, *, #29849, .F. ) ;
#12507=AXIS2_PLACEMENT_3D ( 'NONE', #6354, #33776, #3861 ) ;
#12517=EDGE_LOOP ( 'NONE', ( #6551, #1491, #16660, #10485, #27546, #23812 ) ) ;
#12518=LINE ( 'NONE', #25681, #20260 ) ;
#12520=DIRECTION ( 'NONE',  ( -0.2149704402110242940, 0.9766205557100865464, 0.000000000000000000 ) ) ;
#12527=ORIENTED_EDGE ( 'NONE', *, *, #324, .T. ) ;
#12528=CARTESIAN_POINT ( 'NONE',  ( -5.021133111225196011, -23.57973016998034765, -67.50000000000000000 ) ) ;
#12529=DIRECTION ( 'NONE',  ( -1.000000000000000000, 0.000000000000000000, -0.000000000000000000 ) ) ;
#12545=EDGE_CURVE ( 'NONE', #33018, #19775, #17793, .T. ) ;
#12555=EDGE_CURVE ( 'NONE', #24340, #10848, #34038, .T. ) ;
#12559=ORIENTED_EDGE ( 'NONE', *, *, #3846, .F. ) ;
#12562=PLANE ( 'NONE',  #28857 ) ;
#12565=VERTEX_POINT ( 'NONE', #15989 ) ;
#12592=EDGE_CURVE ( 'NONE', #24229, #19626, #23972, .T. ) ;
#12603=ORIENTED_EDGE ( 'NONE', *, *, #31, .T. ) ;
#12608=CARTESIAN_POINT ( 'NONE',  ( 0.000000000000000000, 6.992329373473909019E-15, 49.43553178847298568 ) ) ;
#12610=LINE ( 'NONE', #12792, #13929 ) ;
#12622=EDGE_CURVE ( 'NONE', #29816, #31010, #2263, .T. ) ;
#12624=VECTOR ( 'NONE', #4202, 1000.000000000000114 ) ;
#12625=LINE ( 'NONE', #23461, #17788 ) ;
#12633=ORIENTED_EDGE ( 'NONE', *, *, #7162, .T. ) ;
#12644=AXIS2_PLACEMENT_3D ( 'NONE', #6285, #19850, #20024 ) ;
#12650=CARTESIAN_POINT ( 'NONE',  ( -20.02113311122498729, -1.691831803474588058, -87.50000000000000000 ) ) ;
#12653=ORIENTED_EDGE ( 'NONE', *, *, #31414, .F. ) ;
#12654=DIRECTION ( 'NONE',  ( 0.000000000000000000, 1.836970198721029441E-16, -1.000000000000000000 ) ) ;
#12655=VERTEX_POINT ( 'NONE', #10813 ) ;
#12659=EDGE_CURVE ( 'NONE', #15568, #22002, #17945, .T. ) ;
#12660=EDGE_CURVE ( 'NONE', #22062, #30758, #8487, .T. ) ;
#12661=CARTESIAN_POINT ( 'NONE',  ( 0.000000000000000000, -33.69708579775585378, -36.68877005347594178 ) ) ;
#12666=EDGE_CURVE ( 'NONE', #16274, #24474, #8131, .T. ) ;
#12674=CARTESIAN_POINT ( 'NONE',  ( 10.17231796313407344, -1.579009122040562207, -77.50000000000000000 ) ) ;
#12675=EDGE_CURVE ( 'NONE', #13441, #19968, #32331, .T. ) ;
#12677=CARTESIAN_POINT ( 'NONE',  ( -35.00000000000000000, -46.95407462254104303, 36.69637551990492597 ) ) ;
#12679=EDGE_LOOP ( 'NONE', ( #11561, #32794, #8312, #23816 ) ) ;
#12681=ORIENTED_EDGE ( 'NONE', *, *, #17944, .F. ) ;
#12682=ORIENTED_EDGE ( 'NONE', *, *, #34139, .F. ) ;
#12688=ADVANCED_FACE ( 'NONE', ( #11882 ), #9190, .T. ) ;
#12689=CARTESIAN_POINT ( 'NONE',  ( 0.000000000000000000, 3.524919873834583163E-15, 68.31122994652405112 ) ) ;
#12705=CARTESIAN_POINT ( 'NONE',  ( 4.815661544189684840, -32.18716788982705168, 49.43553178847298568 ) ) ;
#12708=DIRECTION ( 'NONE',  ( -1.000000000000000000, 6.792721752314501023E-48, -3.697785493223492838E-32 ) ) ;
#12712=ORIENTED_EDGE ( 'NONE', *, *, #8582, .T. ) ;
#12714=CARTESIAN_POINT ( 'NONE',  ( 0.000000000000000000, 3.524919873834583163E-15, 68.31122994652405112 ) ) ;
#12731=EDGE_LOOP ( 'NONE', ( #308, #21879, #16333, #1807, #2508 ) ) ;
#12733=AXIS2_PLACEMENT_3D ( 'NONE', #5122, #11009, #21858 ) ;
#12735=FACE_OUTER_BOUND ( 'NONE', #20878, .T. ) ;
#12737=VERTEX_POINT ( 'NONE', #31089 ) ;
#12746=ORIENTED_EDGE ( 'NONE', *, *, #9566, .F. ) ;
#12758=ORIENTED_EDGE ( 'NONE', *, *, #21261, .T. ) ;
#12759=FACE_OUTER_BOUND ( 'NONE', #33634, .T. ) ;
#12760=ORIENTED_EDGE ( 'NONE', *, *, #12659, .F. ) ;
#12761=DIRECTION ( 'NONE',  ( 1.000000000000000000, 0.000000000000000000, 0.000000000000000000 ) ) ;
#12762=ORIENTED_EDGE ( 'NONE', *, *, #31516, .T. ) ;
#12763=DIRECTION ( 'NONE',  ( -0.7621620551276359068, 0.6473862847818281363, 0.000000000000000000 ) ) ;
#12769=DIRECTION ( 'NONE',  ( 0.4684084406997904848, 0.8835120444460226041, 0.000000000000000000 ) ) ;
#12771=ORIENTED_EDGE ( 'NONE', *, *, #6056, .F. ) ;
#12773=VECTOR ( 'NONE', #8754, 1000.000000000000000 ) ;
#12779=CARTESIAN_POINT ( 'NONE',  ( 0.000000000000000000, 3.524919873834583163E-15, 68.31122994652405112 ) ) ;
#12792=CARTESIAN_POINT ( 'NONE',  ( 37.09133285470120711, -7.633836879289874311, 68.31122994652405112 ) ) ;
#12800=CARTESIAN_POINT ( 'NONE',  ( -14.84098889165989377, 28.96462362251113376, -36.68877005347593467 ) ) ;
#12803=VERTEX_POINT ( 'NONE', #30377 ) ;
#12806=EDGE_CURVE ( 'NONE', #10968, #18461, #5976, .T. ) ;
#12812=CARTESIAN_POINT ( 'NONE',  ( -20.02113311122478123, 16.12922284503173742, -67.50000000000000000 ) ) ;
#12816=VECTOR ( 'NONE', #14671, 1000.000000000000000 ) ;
#12817=ORIENTED_EDGE ( 'NONE', *, *, #11405, .F. ) ;
#12829=CARTESIAN_POINT ( 'NONE',  ( 20.89386240318430765, 24.95297350523388502, 49.43553178847298568 ) ) ;
#12836=CARTESIAN_POINT ( 'NONE',  ( 0.000000000000000000, 6.992329373473909019E-15, 49.43553178847298568 ) ) ;
#12838=VERTEX_POINT ( 'NONE', #9376 ) ;
#12848=LINE ( 'NONE', #9985, #15117 ) ;
#12859=EDGE_CURVE ( 'NONE', #1876, #29973, #5617, .T. ) ;
#12870=EDGE_CURVE ( 'NONE', #18597, #13218, #7031, .T. ) ;
#12871=ORIENTED_EDGE ( 'NONE', *, *, #2830, .F. ) ;
#12875=ORIENTED_EDGE ( 'NONE', *, *, #30630, .F. ) ;
#12882=CARTESIAN_POINT ( 'NONE',  ( 21.85761591200894216, 30.91355005303806180, 49.43553178847298568 ) ) ;
#12888=ORIENTED_EDGE ( 'NONE', *, *, #20133, .T. ) ;
#12889=DIRECTION ( 'NONE',  ( -0.6473862847818272481, 0.7621620551276367950, 1.400068981865443616E-16 ) ) ;
#12897=ORIENTED_EDGE ( 'NONE', *, *, #28604, .F. ) ;
#12902=ORIENTED_EDGE ( 'NONE', *, *, #13300, .T. ) ;
#12904=CIRCLE ( 'NONE', #17473, 32.54542015209054995 ) ;
#12905=ORIENTED_EDGE ( 'NONE', *, *, #9566, .T. ) ;
#12911=ORIENTED_EDGE ( 'NONE', *, *, #32525, .F. ) ;
#12912=CARTESIAN_POINT ( 'NONE',  ( 4.815661544189684840, -32.18716788982705168, 49.43553178847298568 ) ) ;
#12914=VECTOR ( 'NONE', #9281, 1000.000000000000000 ) ;
#12916=PLANE ( 'NONE',  #2900 ) ;
#12917=ORIENTED_EDGE ( 'NONE', *, *, #30425, .T. ) ;
#12919=LINE ( 'NONE', #10765, #15709 ) ;
#12924=ORIENTED_EDGE ( 'NONE', *, *, #1405, .F. ) ;
#12925=LINE ( 'NONE', #34625, #13376 ) ;
#12940=AXIS2_PLACEMENT_3D ( 'NONE', #25646, #17667, #14647 ) ;
#12941=ORIENTED_EDGE ( 'NONE', *, *, #31065, .T. ) ;
#12950=ORIENTED_EDGE ( 'NONE', *, *, #18613, .F. ) ;
#12953=EDGE_LOOP ( 'NONE', ( #29843, #29622, #17738, #16727 ) ) ;
#12955=LINE ( 'NONE', #18647, #5055 ) ;
#12967=ORIENTED_EDGE ( 'NONE', *, *, #16765, .T. ) ;
#12968=DIRECTION ( 'NONE',  ( -0.000000000000000000, -1.836970198721029688E-16, 1.000000000000000000 ) ) ;
#12971=CARTESIAN_POINT ( 'NONE',  ( -18.45373714011839539, 26.80790850550483029, -36.68877005347593467 ) ) ;
#12974=ORIENTED_EDGE ( 'NONE', *, *, #27882, .F. ) ;
#12976=DIRECTION ( 'NONE',  ( 1.000000000000000000, 0.000000000000000000, 0.000000000000000000 ) ) ;
#12980=FACE_OUTER_BOUND ( 'NONE', #2051, .T. ) ;
#12985=CIRCLE ( 'NONE', #14125, 32.54542015209055705 ) ;
#12988=CIRCLE ( 'NONE', #33941, 2.033421858999710619 ) ;
#12993=AXIS2_PLACEMENT_3D ( 'NONE', #21222, #10192, #21042 ) ;
#12994=LINE ( 'NONE', #15138, #25468 ) ;
#13000=CARTESIAN_POINT ( 'NONE',  ( 22.89764159710611224, 17.63622956525712127, -77.50000000000000000 ) ) ;
#13001=EDGE_CURVE ( 'NONE', #7776, #25782, #24380, .T. ) ;
#13002=VECTOR ( 'NONE', #21540, 1000.000000000000114 ) ;
#13004=DIRECTION ( 'NONE',  ( 3.697785493223492838E-32, 1.934419779023891545E-16, -1.000000000000000000 ) ) ;
#13024=LINE ( 'NONE', #18551, #3679 ) ;
#13030=VERTEX_POINT ( 'NONE', #18789 ) ;
#13032=VERTEX_POINT ( 'NONE', #27131 ) ;
#13033=EDGE_CURVE ( 'NONE', #27628, #35091, #10413, .T. ) ;
#13048=CARTESIAN_POINT ( 'NONE',  ( -32.54223829851967764, 0.4550817492056100644, 68.31122994652405112 ) ) ;
#13051=EDGE_CURVE ( 'NONE', #15452, #29720, #2224, .T. ) ;
#13061=DIRECTION ( 'NONE',  ( 0.000000000000000000, 1.836970198721029441E-16, -1.000000000000000000 ) ) ;
#13068=CARTESIAN_POINT ( 'NONE',  ( -18.38714294329533416, -33.09555747561021377, 68.31122994652405112 ) ) ;
#13071=CIRCLE ( 'NONE', #7939, 10.87635688602997597 ) ;
#13073=DIRECTION ( 'NONE',  ( 1.000000000000000000, 0.000000000000000000, 0.000000000000000000 ) ) ;
#13086=ORIENTED_EDGE ( 'NONE', *, *, #893, .T. ) ;
#13094=DIRECTION ( 'NONE',  ( 0.000000000000000000, 1.836970198721029441E-16, -1.000000000000000000 ) ) ;
#13098=CARTESIAN_POINT ( 'NONE',  ( -17.07420202168509604, 33.79163469797343566, -36.68877005347593467 ) ) ;
#13103=ORIENTED_EDGE ( 'NONE', *, *, #25006, .T. ) ;
#13112=CARTESIAN_POINT ( 'NONE',  ( 2.123179190381536685, -33.69708579775584667, 68.31122994652405112 ) ) ;
#13114=DIRECTION ( 'NONE',  ( 0.000000000000000000, 1.836970198721029934E-16, -1.000000000000000000 ) ) ;
#13116=VECTOR ( 'NONE', #16332, 1000.000000000000000 ) ;
#13119=PLANE ( 'NONE',  #26136 ) ;
#13120=VERTEX_POINT ( 'NONE', #25514 ) ;
#13123=VECTOR ( 'NONE', #5703, 1000.000000000000000 ) ;
#13132=DIRECTION ( 'NONE',  ( 0.000000000000000000, -1.000000000000000000, -1.541976423090495633E-16 ) ) ;
#13142=PLANE ( 'NONE',  #9761 ) ;
#13143=CIRCLE ( 'NONE', #5713, 32.54542015209054995 ) ;
#13147=EDGE_CURVE ( 'NONE', #29871, #20735, #17011, .T. ) ;
#13151=FACE_OUTER_BOUND ( 'NONE', #4861, .T. ) ;
#13152=CIRCLE ( 'NONE', #13723, 2.033421858999710619 ) ;
#13154=LINE ( 'NONE', #24503, #29654 ) ;
#13169=ORIENTED_EDGE ( 'NONE', *, *, #15906, .F. ) ;
#13171=DIRECTION ( 'NONE',  ( -0.5155538571770215128, 0.8568571761675892740, 0.000000000000000000 ) ) ;
#13173=VECTOR ( 'NONE', #24672, 1000.000000000000000 ) ;
#13174=ORIENTED_EDGE ( 'NONE', *, *, #5463, .F. ) ;
#13180=AXIS2_PLACEMENT_3D ( 'NONE', #12029, #6660, #25893 ) ;
#13187=EDGE_CURVE ( 'NONE', #26665, #23603, #20018, .T. ) ;
#13188=CARTESIAN_POINT ( 'NONE',  ( 14.70109753509668948, 34.88954974633767137, -36.68877005347593467 ) ) ;
#13191=FACE_OUTER_BOUND ( 'NONE', #708, .T. ) ;
#13192=DIRECTION ( 'NONE',  ( 0.9476531711828023452, -0.3193015301359802827, -0.000000000000000000 ) ) ;
#13202=EDGE_LOOP ( 'NONE', ( #20758, #12155 ) ) ;
#13207=AXIS2_PLACEMENT_3D ( 'NONE', #26480, #24154, #32341 ) ;
#13214=CARTESIAN_POINT ( 'NONE',  ( 36.10877985260814427, 11.38239727801116352, 68.31122994652405112 ) ) ;
#13215=DIRECTION ( 'NONE',  ( 3.697785493223492838E-32, 1.934419779023891545E-16, -1.000000000000000000 ) ) ;
#13217=ORIENTED_EDGE ( 'NONE', *, *, #19511, .T. ) ;
#13218=VERTEX_POINT ( 'NONE', #6111 ) ;
#13222=EDGE_CURVE ( 'NONE', #30722, #17724, #16652, .T. ) ;
#13223=DIRECTION ( 'NONE',  ( -0.6473862847818285804, -0.7621620551276356847, -0.000000000000000000 ) ) ;
#13224=LINE ( 'NONE', #24404, #1755 ) ;
#13226=EDGE_LOOP ( 'NONE', ( #33738, #18960, #20944, #14319 ) ) ;
#13233=PLANE ( 'NONE',  #11230 ) ;
#13235=EDGE_CURVE ( 'NONE', #20173, #18637, #8445, .T. ) ;
#13269=LINE ( 'NONE', #24275, #15694 ) ;
#13270=AXIS2_PLACEMENT_3D ( 'NONE', #4145, #3445, #25518 ) ;
#13287=FACE_OUTER_BOUND ( 'NONE', #16367, .T. ) ;
#13300=EDGE_CURVE ( 'NONE', #33860, #6574, #2805, .T. ) ;
#13306=DIRECTION ( 'NONE',  ( 0.000000000000000000, 1.000000000000000000, 1.934419779023891545E-16 ) ) ;
#13307=ORIENTED_EDGE ( 'NONE', *, *, #12239, .F. ) ;
#13308=ORIENTED_EDGE ( 'NONE', *, *, #18257, .F. ) ;
#13309=CIRCLE ( 'NONE', #30365, 2.036051781435508801 ) ;
#13317=PLANE ( 'NONE',  #4552 ) ;
#13318=CARTESIAN_POINT ( 'NONE',  ( -8.267476927982267298, 31.47782073335735831, 68.31122994652405112 ) ) ;
#13331=CARTESIAN_POINT ( 'NONE',  ( -29.72561944762171393, -13.25111019240559251, 68.31122994652405112 ) ) ;
#13339=ORIENTED_EDGE ( 'NONE', *, *, #31613, .T. ) ;
#13343=VERTEX_POINT ( 'NONE', #6642 ) ;
#13345=EDGE_CURVE ( 'NONE', #32269, #18432, #17540, .T. ) ;
#13346=CARTESIAN_POINT ( 'NONE',  ( 4.748287528889715493E-15, 32.54542015209057837, -87.50000000000000000 ) ) ;
#13349=CARTESIAN_POINT ( 'NONE',  ( 5.021133111224576062, 14.09580098603202458, -67.50000000000000000 ) ) ;
#13359=VECTOR ( 'NONE', #10706, 1000.000000000000114 ) ;
#13362=FACE_OUTER_BOUND ( 'NONE', #34890, .T. ) ;
#13368=DIRECTION ( 'NONE',  ( 0.000000000000000000, 1.836970198721029441E-16, -1.000000000000000000 ) ) ;
#13376=VECTOR ( 'NONE', #16120, 1000.000000000000114 ) ;
#13378=DIRECTION ( 'NONE',  ( -0.000000000000000000, 1.836970198721029688E-16, -1.000000000000000000 ) ) ;
#13381=ORIENTED_EDGE ( 'NONE', *, *, #26035, .F. ) ;
#13388=ORIENTED_EDGE ( 'NONE', *, *, #22996, .F. ) ;
#13390=CARTESIAN_POINT ( 'NONE',  ( -45.00000000000000000, -46.95407462254104303, -36.69637551990492597 ) ) ;
#13391=DIRECTION ( 'NONE',  ( 0.8276889981568903432, -0.5611870653623828309, 0.000000000000000000 ) ) ;
#13393=VECTOR ( 'NONE', #23076, 1000.000000000000000 ) ;
#13395=ORIENTED_EDGE ( 'NONE', *, *, #20099, .F. ) ;
#13397=DIRECTION ( 'NONE',  ( -0.4198891015602651544, 0.9075754196709567845, 0.000000000000000000 ) ) ;
#13402=PLANE ( 'NONE',  #17722 ) ;
#13405=DIRECTION ( 'NONE',  ( -0.4684084406997903738, -0.8835120444460228262, -1.622985295858433536E-16 ) ) ;
#13407=VECTOR ( 'NONE', #25828, 1000.000000000000000 ) ;
#13410=DIRECTION ( 'NONE',  ( 0.000000000000000000, 0.000000000000000000, 1.000000000000000000 ) ) ;
#13415=DIRECTION ( 'NONE',  ( 3.697785493223492838E-32, 1.934419779023891545E-16, -1.000000000000000000 ) ) ;
#13421=CIRCLE ( 'NONE', #20807, 2.036051781435508801 ) ;
#13423=ADVANCED_FACE ( 'NONE', ( #860 ), #33592, .F. ) ;
#13424=VERTEX_POINT ( 'NONE', #14401 ) ;
#13425=CARTESIAN_POINT ( 'NONE',  ( 0.000000000000000000, 2.281310696040539424E-14, -36.68877005347592757 ) ) ;
#13436=CARTESIAN_POINT ( 'NONE',  ( 12.46788440507150320, 30.06253867087537657, 68.31122994652405112 ) ) ;
#13437=CARTESIAN_POINT ( 'NONE',  ( 0.000000000000000000, 3.524919873834583163E-15, 68.31122994652405112 ) ) ;
#13438=ADVANCED_FACE ( 'NONE', ( #19909 ), #22921, .F. ) ;
#13441=VERTEX_POINT ( 'NONE', #30751 ) ;
#13450=LINE ( 'NONE', #24281, #4103 ) ;
#13455=DIRECTION ( 'NONE',  ( 0.000000000000000000, -1.000000000000000000, 0.000000000000000000 ) ) ;
#13460=ORIENTED_EDGE ( 'NONE', *, *, #29540, .F. ) ;
#13462=ORIENTED_EDGE ( 'NONE', *, *, #10951, .T. ) ;
#13468=EDGE_CURVE ( 'NONE', #32774, #17833, #25554, .T. ) ;
#13472=ORIENTED_EDGE ( 'NONE', *, *, #28939, .F. ) ;
#13475=ORIENTED_EDGE ( 'NONE', *, *, #9337, .F. ) ;
#13476=DIRECTION ( 'NONE',  ( 1.000000000000000000, 0.000000000000000000, 0.000000000000000000 ) ) ;
#13482=DIRECTION ( 'NONE',  ( 0.000000000000000000, 0.000000000000000000, 1.000000000000000000 ) ) ;
#13484=VERTEX_POINT ( 'NONE', #17605 ) ;
#13510=LINE ( 'NONE', #21860, #26025 ) ;
#13513=AXIS2_PLACEMENT_3D ( 'NONE', #30368, #2953, #33212 ) ;
#13515=CARTESIAN_POINT ( 'NONE',  ( -45.00000000000000000, 3.353962854566122864, 15.81122994652406355 ) ) ;
#13522=AXIS2_PLACEMENT_3D ( 'NONE', #31758, #7367, #1530 ) ;
#13529=LINE ( 'NONE', #2661, #13002 ) ;
#13534=VECTOR ( 'NONE', #2554, 1000.000000000000114 ) ;
#13536=ORIENTED_EDGE ( 'NONE', *, *, #8436, .T. ) ;
#13539=CARTESIAN_POINT ( 'NONE',  ( -32.54223829851967764, 0.4550817492056293823, -36.68877005347593467 ) ) ;
#13541=CARTESIAN_POINT ( 'NONE',  ( -5.021133111224679091, 24.02303923978504940, -67.50000000000000000 ) ) ;
#13565=DIRECTION ( 'NONE',  ( -0.000000000000000000, -0.000000000000000000, -1.000000000000000000 ) ) ;
#13566=EDGE_LOOP ( 'NONE', ( #13599, #21130, #9656, #16415 ) ) ;
#13568=CARTESIAN_POINT ( 'NONE',  ( 1.532562817202168137, 32.50931595846690669, 68.31122994652405112 ) ) ;
#13569=DIRECTION ( 'NONE',  ( 0.9985334138511240409, -0.05413890858541543089, -9.945156166269024927E-18 ) ) ;
#13570=EDGE_CURVE ( 'NONE', #11101, #1704, #13637, .T. ) ;
#13580=ADVANCED_FACE ( 'NONE', ( #16674 ), #13119, .T. ) ;
#13582=FACE_OUTER_BOUND ( 'NONE', #25745, .T. ) ;
#13584=CARTESIAN_POINT ( 'NONE',  ( 32.54460952423471554, 0.2297037030477364072, 49.43553178847298568 ) ) ;
#13586=AXIS2_PLACEMENT_3D ( 'NONE', #24358, #27869, #3313 ) ;
#13587=CARTESIAN_POINT ( 'NONE',  ( 27.64943126350854286, -17.16721653852533791, 49.43553178847298568 ) ) ;
#13599=ORIENTED_EDGE ( 'NONE', *, *, #19261, .T. ) ;
#13602=AXIS2_PLACEMENT_3D ( 'NONE', #24403, #16254, #22106 ) ;
#13605=ORIENTED_EDGE ( 'NONE', *, *, #1015, .F. ) ;
#13607=DIRECTION ( 'NONE',  ( 0.000000000000000000, 1.836970198721029688E-16, -1.000000000000000000 ) ) ;
#13608=LINE ( 'NONE', #2385, #4405 ) ;
#13612=CARTESIAN_POINT ( 'NONE',  ( 10.17231796313409298, 8.346743312457581609, -87.50000000000000000 ) ) ;
#13614=EDGE_LOOP ( 'NONE', ( #29935, #33227, #27432, #16278 ) ) ;
#13615=EDGE_CURVE ( 'NONE', #9940, #3430, #23953, .T. ) ;
#13623=EDGE_CURVE ( 'NONE', #23058, #27275, #13071, .T. ) ;
#13627=LINE ( 'NONE', #24286, #24795 ) ;
#13629=VECTOR ( 'NONE', #19059, 1000.000000000000000 ) ;
#13634=ORIENTED_EDGE ( 'NONE', *, *, #31016, .T. ) ;
#13636=DIRECTION ( 'NONE',  ( -1.000000000000000000, 6.792721752314501023E-48, -3.697785493223492838E-32 ) ) ;
#13637=LINE ( 'NONE', #21640, #23304 ) ;
#13643=CARTESIAN_POINT ( 'NONE',  ( 23.93847777447631131, 22.04889236939138542, 49.43553178847298568 ) ) ;
#13644=CARTESIAN_POINT ( 'NONE',  ( -32.32899628990713126, -3.747048406849353697, 68.31122994652405112 ) ) ;
#13649=PLANE ( 'NONE',  #2687 ) ;
#13660=ORIENTED_EDGE ( 'NONE', *, *, #937, .T. ) ;
#13671=DIRECTION ( 'NONE',  ( 0.9985334138511239299, -0.05413890858541752643, -0.000000000000000000 ) ) ;
#13673=ORIENTED_EDGE ( 'NONE', *, *, #22257, .F. ) ;
#13674=CIRCLE ( 'NONE', #3506, 2.033421858999711507 ) ;
#13679=DIRECTION ( 'NONE',  ( -0.9635499925192230197, -0.2675283385292205329, 0.000000000000000000 ) ) ;
#13684=EDGE_LOOP ( 'NONE', ( #12087, #14465, #17262, #1074 ) ) ;
#13693=ADVANCED_FACE ( 'NONE', ( #25848 ), #23187, .F. ) ;
#13703=AXIS2_PLACEMENT_3D ( 'NONE', #13921, #16604, #11252 ) ;
#13705=CARTESIAN_POINT ( 'NONE',  ( 21.24400529595486731, -24.65555945140049232, 49.43553178847298568 ) ) ;
#13710=CARTESIAN_POINT ( 'NONE',  ( 18.63894936814906345, 26.67946662374789213, 49.43553178847298568 ) ) ;
#13718=EDGE_LOOP ( 'NONE', ( #16530, #4915, #11291, #34500, #2268, #20208 ) ) ;
#13723=AXIS2_PLACEMENT_3D ( 'NONE', #8359, #16562, #22066 ) ;
#13728=AXIS2_PLACEMENT_3D ( 'NONE', #282, #30709, #805 ) ;
#13735=LINE ( 'NONE', #29752, #30041 ) ;
#13737=ORIENTED_EDGE ( 'NONE', *, *, #15682, .T. ) ;
#13753=CARTESIAN_POINT ( 'NONE',  ( -13.53398258527560749, -35.36769364574537633, -36.68877005347593467 ) ) ;
#13765=AXIS2_PLACEMENT_3D ( 'NONE', #32915, #24543, #22074 ) ;
#13770=VERTEX_POINT ( 'NONE', #34735 ) ;
#13772=DIRECTION ( 'NONE',  ( 0.000000000000000000, 1.000000000000000000, 1.836970198721029688E-16 ) ) ;
#13775=DIRECTION ( 'NONE',  ( -0.6051742151937650194, -0.7960930657056438653, 0.000000000000000000 ) ) ;
#13782=PLANE ( 'NONE',  #27321 ) ;
#13785=CIRCLE ( 'NONE', #13207, 2.085824230283342740 ) ;
#13788=DIRECTION ( 'NONE',  ( -0.000000000000000000, -0.000000000000000000, -1.000000000000000000 ) ) ;
#13794=FACE_OUTER_BOUND ( 'NONE', #19136, .T. ) ;
#13795=CARTESIAN_POINT ( 'NONE',  ( -45.00000000000000000, 16.36947364650383818, 36.69637551990492597 ) ) ;
#13796=CARTESIAN_POINT ( 'NONE',  ( 13.32059394339353986, -35.43959265050632013, -36.68877005347593467 ) ) ;
#13806=ORIENTED_EDGE ( 'NONE', *, *, #23258, .F. ) ;
#13809=PLANE ( 'NONE',  #16593 ) ;
#13816=ORIENTED_EDGE ( 'NONE', *, *, #1292, .T. ) ;
#13836=DIRECTION ( 'NONE',  ( -0.000000000000000000, -1.836970198721029688E-16, 1.000000000000000000 ) ) ;
#13838=CARTESIAN_POINT ( 'NONE',  ( 0.000000000000000000, -33.69708579775584667, 49.43553178847298568 ) ) ;
#13844=CARTESIAN_POINT ( 'NONE',  ( 0.000000000000000000, -33.69708579775584667, 49.43553178847298568 ) ) ;
#13862=LINE ( 'NONE', #24701, #16774 ) ;
#13864=ORIENTED_EDGE ( 'NONE', *, *, #442, .T. ) ;
#13865=ORIENTED_EDGE ( 'NONE', *, *, #6971, .F. ) ;
#13868=CARTESIAN_POINT ( 'NONE',  ( 20.62763069236413926, -31.74750072459299588, 68.31122994652405112 ) ) ;
#13873=ORIENTED_EDGE ( 'NONE', *, *, #33298, .T. ) ;
#13879=PLANE ( 'NONE',  #22087 ) ;
#13880=EDGE_CURVE ( 'NONE', #32148, #21072, #29573, .T. ) ;
#13881=CARTESIAN_POINT ( 'NONE',  ( 3.235562306570555532E-30, 1.325223266901699007E-14, -67.50000000000000000 ) ) ;
#13882=ORIENTED_EDGE ( 'NONE', *, *, #7538, .T. ) ;
#13891=CIRCLE ( 'NONE', #8766, 2.033421858999711951 ) ;
#13892=FACE_OUTER_BOUND ( 'NONE', #27711, .T. ) ;
#13918=FACE_OUTER_BOUND ( 'NONE', #21485, .T. ) ;
#13920=DIRECTION ( 'NONE',  ( -0.000000000000000000, -1.836970198721029688E-16, 1.000000000000000000 ) ) ;
#13921=CARTESIAN_POINT ( 'NONE',  ( 0.000000000000000000, 6.992329373473909019E-15, 49.43553178847298568 ) ) ;
#13923=EDGE_LOOP ( 'NONE', ( #8424, #28536 ) ) ;
#13929=VECTOR ( 'NONE', #33606, 1000.000000000000000 ) ;
#13940=VERTEX_POINT ( 'NONE', #8551 ) ;
#13944=AXIS2_PLACEMENT_3D ( 'NONE', #25882, #28894, #17713 ) ;
#13948=ORIENTED_EDGE ( 'NONE', *, *, #11262, .T. ) ;
#13949=EDGE_CURVE ( 'NONE', #1876, #20519, #30268, .T. ) ;
#13951=VECTOR ( 'NONE', #30100, 1000.000000000000000 ) ;
#13953=AXIS2_PLACEMENT_3D ( 'NONE', #4009, #17933, #28759 ) ;
#13955=PLANE ( 'NONE',  #16749 ) ;
#13968=CARTESIAN_POINT ( 'NONE',  ( 8.927936315454015670, -31.29690601358702651, 49.43553178847298568 ) ) ;
#13969=CIRCLE ( 'NONE', #2035, 32.54542015209055705 ) ;
#13970=CARTESIAN_POINT ( 'NONE',  ( -45.00000000000000000, -46.95407462254104303, 36.69637551990492597 ) ) ;
#13973=LINE ( 'NONE', #3273, #13985 ) ;
#13976=LINE ( 'NONE', #8268, #21978 ) ;
#13982=EDGE_LOOP ( 'NONE', ( #27604, #5120, #15903, #31644 ) ) ;
#13985=VECTOR ( 'NONE', #16835, 1000.000000000000000 ) ;
#13986=EDGE_CURVE ( 'NONE', #18999, #6917, #3385, .T. ) ;
#13989=CARTESIAN_POINT ( 'NONE',  ( -35.00000000000000000, 42.49491490430484220, 36.69637551990492597 ) ) ;
#13990=DIRECTION ( 'NONE',  ( 1.000000000000000000, 0.000000000000000000, 0.000000000000000000 ) ) ;
#13991=VECTOR ( 'NONE', #7834, 1000.000000000000000 ) ;
#13993=ORIENTED_EDGE ( 'NONE', *, *, #7009, .F. ) ;
#13998=FACE_OUTER_BOUND ( 'NONE', #31244, .T. ) ;
#14002=CARTESIAN_POINT ( 'NONE',  ( 23.31255882915078814, -22.70966696615089830, 68.31122994652405112 ) ) ;
#14005=CARTESIAN_POINT ( 'NONE',  ( 0.000000000000000000, -33.69708579775584667, -36.68877005347592757 ) ) ;
#14013=CARTESIAN_POINT ( 'NONE',  ( 0.000000000000000000, 3.524919873834583163E-15, 68.31122994652405112 ) ) ;
#14019=LINE ( 'NONE', #27706, #33106 ) ;
#14028=EDGE_CURVE ( 'NONE', #29720, #20094, #25978, .T. ) ;
#14029=EDGE_LOOP ( 'NONE', ( #33090, #3962, #10533, #16475 ) ) ;
#14030=LINE ( 'NONE', #3683, #26806 ) ;
#14043=ORIENTED_EDGE ( 'NONE', *, *, #16583, .T. ) ;
#14049=DIRECTION ( 'NONE',  ( 0.9289767198167914186, -0.3701381553399144542, 0.000000000000000000 ) ) ;
#14062=DIRECTION ( 'NONE',  ( 0.000000000000000000, 1.000000000000000000, 0.000000000000000000 ) ) ;
#14063=EDGE_CURVE ( 'NONE', #15632, #23681, #9451, .T. ) ;
#14066=DIRECTION ( 'NONE',  ( 0.000000000000000000, 1.836970198721029441E-16, -1.000000000000000000 ) ) ;
#14068=EDGE_CURVE ( 'NONE', #7373, #9180, #11947, .T. ) ;
#14069=DIRECTION ( 'NONE',  ( -0.7621620551276356847, -0.6473862847818285804, -1.189229312204944401E-16 ) ) ;
#14070=DIRECTION ( 'NONE',  ( 1.000000000000000000, -0.000000000000000000, -0.000000000000000000 ) ) ;
#14094=CARTESIAN_POINT ( 'NONE',  ( -25.07182831876307105, -28.36910952062232738, -36.68877005347593467 ) ) ;
#14098=DIRECTION ( 'NONE',  ( -0.000000000000000000, 1.836970198721029688E-16, -1.000000000000000000 ) ) ;
#14103=AXIS2_PLACEMENT_3D ( 'NONE', #149, #29700, #7801 ) ;
#14111=DIRECTION ( 'NONE',  ( 0.9476531711828030113, 0.3193015301359780622, -0.000000000000000000 ) ) ;
#14112=AXIS2_PLACEMENT_3D ( 'NONE', #20009, #9134, #255 ) ;
#14118=( NAMED_UNIT ( * ) PLANE_ANGLE_UNIT ( ) SI_UNIT ( $, .RADIAN. ) );
#14120=VECTOR ( 'NONE', #19092, 1000.000000000000000 ) ;
#14124=EDGE_LOOP ( 'NONE', ( #12917, #15797, #4530, #17035 ) ) ;
#14125=AXIS2_PLACEMENT_3D ( 'NONE', #15669, #2119, #25802 ) ;
#14128=LINE ( 'NONE', #25318, #17338 ) ;
#14133=AXIS2_PLACEMENT_3D ( 'NONE', #28365, #13569, #15539 ) ;
#14150=VECTOR ( 'NONE', #31369, 1000.000000000000000 ) ;
#14154=CARTESIAN_POINT ( 'NONE',  ( -35.00000000000000000, -46.95407462254104303, 36.69637551990492597 ) ) ;
#14160=DIRECTION ( 'NONE',  ( -0.000000000000000000, 1.000000000000000000, 0.000000000000000000 ) ) ;
#14163=CARTESIAN_POINT ( 'NONE',  ( 5.021133111224162171, -21.54630831098063837, -67.50000000000000000 ) ) ;
#14165=VECTOR ( 'NONE', #27701, 1000.000000000000000 ) ;
#14169=DIRECTION ( 'NONE',  ( 0.9941379571543593752, -0.1081190184239433083, -0.000000000000000000 ) ) ;
#14172=ADVANCED_FACE ( 'NONE', ( #29179 ), #31819, .T. ) ;
#14174=AXIS2_PLACEMENT_3D ( 'NONE', #29187, #26510, #4781 ) ;
#14180=LINE ( 'NONE', #22355, #3062 ) ;
#14183=DIRECTION ( 'NONE',  ( -0.000000000000000000, 1.836970198721029688E-16, -1.000000000000000000 ) ) ;
#14188=LINE ( 'NONE', #25014, #33403 ) ;
#14195=LINE ( 'NONE', #30193, #11111 ) ;
#14203=ORIENTED_EDGE ( 'NONE', *, *, #8142, .F. ) ;
#14204=CIRCLE ( 'NONE', #26099, 32.54542015209055705 ) ;
#14207=ORIENTED_EDGE ( 'NONE', *, *, #9555, .T. ) ;
#14210=VERTEX_POINT ( 'NONE', #13515 ) ;
#14221=PLANE ( 'NONE',  #26638 ) ;
#14227=ORIENTED_EDGE ( 'NONE', *, *, #11704, .T. ) ;
#14231=EDGE_CURVE ( 'NONE', #12281, #29036, #28016, .T. ) ;
#14235=EDGE_CURVE ( 'NONE', #33527, #5237, #3518, .T. ) ;
#14237=EDGE_LOOP ( 'NONE', ( #2401, #25362, #9354, #7923 ) ) ;
#14238=ORIENTED_EDGE ( 'NONE', *, *, #7420, .F. ) ;
#14240=ORIENTED_EDGE ( 'NONE', *, *, #22834, .F. ) ;
#14242=LINE ( 'NONE', #11566, #29086 ) ;
#14248=ORIENTED_EDGE ( 'NONE', *, *, #13222, .T. ) ;
#14256=EDGE_LOOP ( 'NONE', ( #8070, #18243, #17523, #5806, #5910, #11991, #20319, #10579 ) ) ;
#14258=VECTOR ( 'NONE', #10458, 1000.000000000000114 ) ;
#14265=ADVANCED_FACE ( 'NONE', ( #866 ), #17259, .T. ) ;
#14272=CARTESIAN_POINT ( 'NONE',  ( -34.04247984038124031, 16.56841925338182619, -36.68877005347593467 ) ) ;
#14276=VERTEX_POINT ( 'NONE', #6181 ) ;
#14277=LINE ( 'NONE', #2864, #3210 ) ;
#14279=EDGE_CURVE ( 'NONE', #5820, #35091, #17076, .T. ) ;
#14282=PLANE ( 'NONE',  #11594 ) ;
#14291=CYLINDRICAL_SURFACE ( 'NONE', #85, 2.085824230283342740 ) ;
#14293=DIRECTION ( 'NONE',  ( 0.000000000000000000, 1.836970198721029441E-16, -1.000000000000000000 ) ) ;
#14312=FACE_OUTER_BOUND ( 'NONE', #590, .T. ) ;
#14317=DIRECTION ( 'NONE',  ( -0.4684084406997904848, 0.8835120444460226041, -0.000000000000000000 ) ) ;
#14318=CARTESIAN_POINT ( 'NONE',  ( 5.021133111224576062, 18.16264470403145026, -67.50000000000000000 ) ) ;
#14319=ORIENTED_EDGE ( 'NONE', *, *, #16950, .F. ) ;
#14334=DIRECTION ( 'NONE',  ( -0.9766205557100864354, 0.2149704402110247659, -0.000000000000000000 ) ) ;
#14337=VECTOR ( 'NONE', #7773, 1000.000000000000000 ) ;
#14339=LINE ( 'NONE', #19317, #23055 ) ;
#14340=LINE ( 'NONE', #9512, #24595 ) ;
#14346=DIRECTION ( 'NONE',  ( 0.000000000000000000, 1.000000000000000000, 0.000000000000000000 ) ) ;
#14350=EDGE_LOOP ( 'NONE', ( #17029, #29000, #4273, #31292 ) ) ;
#14351=CARTESIAN_POINT ( 'NONE',  ( -32.32899628990712415, -3.747048406849351032, -15.81122994652406355 ) ) ;
#14354=ORIENTED_EDGE ( 'NONE', *, *, #32891, .F. ) ;
#14359=DIRECTION ( 'NONE',  ( -0.9868265225415262520, 0.1617819965527638459, 2.971887063570155659E-17 ) ) ;
#14366=ORIENTED_EDGE ( 'NONE', *, *, #32891, .T. ) ;
#14368=DIRECTION ( 'NONE',  ( 3.697785493223492838E-32, 1.934419779023891545E-16, -1.000000000000000000 ) ) ;
#14370=CARTESIAN_POINT ( 'NONE',  ( 3.235562306570555532E-30, -15.68591377522703745, -67.50000000000000000 ) ) ;
#14378=DIRECTION ( 'NONE',  ( -0.000000000000000000, -1.000000000000000000, -0.000000000000000000 ) ) ;
#14379=DIRECTION ( 'NONE',  ( -0.8276889981568902321, -0.5611870653623829419, 0.000000000000000000 ) ) ;
#14382=ORIENTED_EDGE ( 'NONE', *, *, #32847, .F. ) ;
#14387=ORIENTED_EDGE ( 'NONE', *, *, #22301, .F. ) ;
#14401=CARTESIAN_POINT ( 'NONE',  ( 29.83064097883987742, 23.32756518004832813, 68.31122994652405112 ) ) ;
#14407=CARTESIAN_POINT ( 'NONE',  ( -31.68358972719163091, 7.440061483287530919, 68.31122994652405112 ) ) ;
#14410=VERTEX_POINT ( 'NONE', #25945 ) ;
#14416=LINE ( 'NONE', #25239, #11986 ) ;
#14419=CARTESIAN_POINT ( 'NONE',  ( -35.00000000000000000, 0.5883377166429051286, 15.81122994652406355 ) ) ;
#14420=VERTEX_POINT ( 'NONE', #18302 ) ;
#14424=ORIENTED_EDGE ( 'NONE', *, *, #5213, .T. ) ;
#14425=CARTESIAN_POINT ( 'NONE',  ( 5.021133111224265200, -13.65249191622732816, -67.50000000000000000 ) ) ;
#14426=DIRECTION ( 'NONE',  ( -0.6473862847818281363, -0.7621620551276360178, -1.400068981865441644E-16 ) ) ;
#14428=DIRECTION ( 'NONE',  ( 0.9941379571543594862, 0.1081190184239433083, -0.000000000000000000 ) ) ;
#14432=LINE ( 'NONE', #31265, #23658 ) ;
#14434=AXIS2_PLACEMENT_3D ( 'NONE', #27230, #24204, #4978 ) ;
#14455=ORIENTED_EDGE ( 'NONE', *, *, #4986, .T. ) ;
#14458=CARTESIAN_POINT ( 'NONE',  ( -45.00000000000000000, -46.95407462254104303, 36.69637551990492597 ) ) ;
#14459=CARTESIAN_POINT ( 'NONE',  ( 22.89764159710613001, 6.310691531022070144, -77.50000000000000000 ) ) ;
#14465=ORIENTED_EDGE ( 'NONE', *, *, #30216, .T. ) ;
#14471=VECTOR ( 'NONE', #28437, 1000.000000000000000 ) ;
#14485=CIRCLE ( 'NONE', #2511, 32.54542015209056416 ) ;
#14488=CARTESIAN_POINT ( 'NONE',  ( -5.021133111225196011, -23.57973016998034765, -67.50000000000000000 ) ) ;
#14493=VECTOR ( 'NONE', #5914, 1000.000000000000000 ) ;
#14496=FACE_OUTER_BOUND ( 'NONE', #11150, .T. ) ;
#14499=CARTESIAN_POINT ( 'NONE',  ( -5.021133111224989953, -3.725253662474303784, -67.50000000000000000 ) ) ;
#14501=FACE_OUTER_BOUND ( 'NONE', #12386, .T. ) ;
#14504=EDGE_LOOP ( 'NONE', ( #3438, #12424, #31068, #16510 ) ) ;
#14506=CARTESIAN_POINT ( 'NONE',  ( -5.021133111224886036, 8.235406450278427215, -67.50000000000000000 ) ) ;
#14512=CARTESIAN_POINT ( 'NONE',  ( -18.45373714011839539, 26.80790850550480542, 68.31122994652405112 ) ) ;
#14517=CARTESIAN_POINT ( 'NONE',  ( 0.000000000000000000, 3.524919873834583163E-15, 68.31122994652405112 ) ) ;
#14518=ORIENTED_EDGE ( 'NONE', *, *, #323, .F. ) ;
#14520=DIRECTION ( 'NONE',  ( -1.000000000000000000, 0.000000000000000000, 0.000000000000000000 ) ) ;
#14527=EDGE_CURVE ( 'NONE', #802, #27628, #28787, .T. ) ;
#14533=VECTOR ( 'NONE', #10830, 1000.000000000000000 ) ;
#14538=DIRECTION ( 'NONE',  ( -0.9052067871510964814, -0.3606673485459944151, -0.2247659586956878841 ) ) ;
#14544=ORIENTED_EDGE ( 'NONE', *, *, #18175, .F. ) ;
#14545=VERTEX_POINT ( 'NONE', #27161 ) ;
#14546=LINE ( 'NONE', #9013, #1443 ) ;
#14563=CARTESIAN_POINT ( 'NONE',  ( -30.91434716440808472, 10.17386417614053151, 68.31122994652405112 ) ) ;
#14571=ORIENTED_EDGE ( 'NONE', *, *, #9971, .T. ) ;
#14581=DIRECTION ( 'NONE',  ( 0.4198891015602640997, 0.9075754196709573396, -0.000000000000000000 ) ) ;
#14584=VERTEX_POINT ( 'NONE', #3130 ) ;
#14588=VECTOR ( 'NONE', #18888, 1000.000000000000000 ) ;
#14599=ADVANCED_FACE ( 'NONE', ( #16508 ), #18250, .T. ) ;
#14600=LINE ( 'NONE', #3535, #7878 ) ;
#14603=ORIENTED_EDGE ( 'NONE', *, *, #12592, .T. ) ;
#14604=EDGE_CURVE ( 'NONE', #26369, #22562, #29841, .T. ) ;
#14607=EDGE_CURVE ( 'NONE', #1041, #8787, #5090, .T. ) ;
#14609=ORIENTED_EDGE ( 'NONE', *, *, #26828, .F. ) ;
#14610=VECTOR ( 'NONE', #19849, 1000.000000000000114 ) ;
#14618=ORIENTED_EDGE ( 'NONE', *, *, #27911, .F. ) ;
#14621=EDGE_CURVE ( 'NONE', #17657, #25488, #11335, .T. ) ;
#14624=ORIENTED_EDGE ( 'NONE', *, *, #19419, .T. ) ;
#14627=VECTOR ( 'NONE', #1740, 1000.000000000000000 ) ;
#14630=ORIENTED_EDGE ( 'NONE', *, *, #12555, .T. ) ;
#14631=DIRECTION ( 'NONE',  ( 0.000000000000000000, 1.836970198721029934E-16, -1.000000000000000000 ) ) ;
#14634=CARTESIAN_POINT ( 'NONE',  ( -35.00000000000000000, -4.831299144296466785, -15.81122994652406355 ) ) ;
#14637=CARTESIAN_POINT ( 'NONE',  ( -1.307386931792819285, 37.83772838912472025, -36.68877005347593467 ) ) ;
#14647=DIRECTION ( 'NONE',  ( 1.000000000000000000, 0.000000000000000000, -0.000000000000000000 ) ) ;
#14652=LINE ( 'NONE', #30657, #23639 ) ;
#14655=DIRECTION ( 'NONE',  ( -0.000000000000000000, 1.836970198721029688E-16, -1.000000000000000000 ) ) ;
#14656=ADVANCED_FACE ( 'NONE', ( #29664 ), #32677, .T. ) ;
#14658=ORIENTED_EDGE ( 'NONE', *, *, #557, .T. ) ;
#14659=DIRECTION ( 'NONE',  ( -0.000000000000000000, 1.836970198721029934E-16, -1.000000000000000000 ) ) ;
#14660=DIRECTION ( 'NONE',  ( -0.9818488882034280829, -0.1609659548241205163, 0.1003131203843820873 ) ) ;
#14664=ORIENTED_EDGE ( 'NONE', *, *, #2951, .T. ) ;
#14671=DIRECTION ( 'NONE',  ( 0.000000000000000000, 1.836970198721029441E-16, -1.000000000000000000 ) ) ;
#14674=VECTOR ( 'NONE', #712, 1000.000000000000000 ) ;
#14677=DIRECTION ( 'NONE',  ( 0.1617819965527648451, -0.9868265225415261410, -1.812770913216290044E-16 ) ) ;
#14689=EDGE_CURVE ( 'NONE', #23884, #31849, #22540, .T. ) ;
#14694=LINE ( 'NONE', #25697, #21789 ) ;
#14710=ORIENTED_EDGE ( 'NONE', *, *, #28453, .F. ) ;
#14711=VECTOR ( 'NONE', #18748, 1000.000000000000000 ) ;
#14717=VECTOR ( 'NONE', #27785, 1000.000000000000000 ) ;
#14721=VERTEX_POINT ( 'NONE', #17220 ) ;
#14723=EDGE_CURVE ( 'NONE', #16741, #24257, #19523, .T. ) ;
#14725=DIRECTION ( 'NONE',  ( 0.9635499925192230197, 0.2675283385292205329, 0.000000000000000000 ) ) ;
#14743=ADVANCED_FACE ( 'NONE', ( #12044 ), #5965, .F. ) ;
#14747=DIRECTION ( 'NONE',  ( 0.9868265225415260300, 0.1617819965527650394, -0.000000000000000000 ) ) ;
#14749=ORIENTED_EDGE ( 'NONE', *, *, #34974, .T. ) ;
#14752=DIRECTION ( 'NONE',  ( -0.000000000000000000, 1.836970198721029934E-16, -1.000000000000000000 ) ) ;
#14753=ORIENTED_EDGE ( 'NONE', *, *, #14235, .F. ) ;
#14754=LINE ( 'NONE', #31114, #14471 ) ;
#14755=VECTOR ( 'NONE', #21447, 1000.000000000000000 ) ;
#14771=EDGE_CURVE ( 'NONE', #23775, #15441, #33736, .T. ) ;
#14772=DIRECTION ( 'NONE',  ( -1.000000000000000000, 6.792721752314501023E-48, -3.697785493223492838E-32 ) ) ;
#14773=EDGE_CURVE ( 'NONE', #5171, #26118, #13143, .T. ) ;
#14779=DIRECTION ( 'NONE',  ( -1.000000000000000000, 6.792721752314501023E-48, -3.697785493223492838E-32 ) ) ;
#14786=CARTESIAN_POINT ( 'NONE',  ( 22.89764159710611224, 15.60017778382161424, -87.50000000000000000 ) ) ;
#14788=VERTEX_POINT ( 'NONE', #3476 ) ;
#14798=ORIENTED_EDGE ( 'NONE', *, *, #19174, .T. ) ;
#14799=DIRECTION ( 'NONE',  ( 1.000000000000000000, 0.000000000000000000, 0.000000000000000000 ) ) ;
#14807=DIRECTION ( 'NONE',  ( 0.000000000000000000, -1.000000000000000000, -1.836970198721029934E-16 ) ) ;
#14816=CARTESIAN_POINT ( 'NONE',  ( -37.85301660235036536, 0.7430237821112573027, 68.31122994652405112 ) ) ;
#14820=CARTESIAN_POINT ( 'NONE',  ( -11.83261234297099662, -30.31820670846266097, -36.68877005347593467 ) ) ;
#14826=VECTOR ( 'NONE', #30362, 1000.000000000000114 ) ;
#14848=LINE ( 'NONE', #32415, #19697 ) ;
#14857=CARTESIAN_POINT ( 'NONE',  ( 0.000000000000000000, 3.172845296185191895E-14, -85.22165320886810491 ) ) ;
#14870=VERTEX_POINT ( 'NONE', #1525 ) ;
#14884=ORIENTED_EDGE ( 'NONE', *, *, #31414, .T. ) ;
#14885=DIRECTION ( 'NONE',  ( 0.000000000000000000, 1.000000000000000000, 1.934419779023891545E-16 ) ) ;
#14889=VECTOR ( 'NONE', #16920, 1000.000000000000000 ) ;
#14896=VECTOR ( 'NONE', #6831, 1000.000000000000000 ) ;
#14897=CARTESIAN_POINT ( 'NONE',  ( 32.05156013847309993, -20.15193397489277771, 68.31122994652405112 ) ) ;
#14900=DIRECTION ( 'NONE',  ( 0.7621620551276356847, -0.6473862847818285804, -1.189229312204944401E-16 ) ) ;
#14901=DIRECTION ( 'NONE',  ( 0.000000000000000000, 1.000000000000000000, 0.000000000000000000 ) ) ;
#14910=DIRECTION ( 'NONE',  ( -0.4684084406997904848, -0.8835120444460226041, -0.000000000000000000 ) ) ;
#14921=ADVANCED_FACE ( 'NONE', ( #12735 ), #12916, .F. ) ;
#14925=ORIENTED_EDGE ( 'NONE', *, *, #963, .F. ) ;
#14927=CARTESIAN_POINT ( 'NONE',  ( 0.000000000000000000, 2.281310696040539424E-14, -36.68877005347592757 ) ) ;
#14931=ORIENTED_EDGE ( 'NONE', *, *, #20714, .F. ) ;
#14939=VECTOR ( 'NONE', #19149, 1000.000000000000114 ) ;
#14940=AXIS2_PLACEMENT_3D ( 'NONE', #12374, #31567, #34421 ) ;
#14967=CARTESIAN_POINT ( 'NONE',  ( 27.64943126350854286, -17.16721653852534146, 68.31122994652405112 ) ) ;
#14969=DIRECTION ( 'NONE',  ( 0.1452892791026232089, 0.5232846903699686081, 0.8396809859716046764 ) ) ;
#14970=ADVANCED_FACE ( 'NONE', ( #21437 ), #13782, .F. ) ;
#14972=VERTEX_POINT ( 'NONE', #21779 ) ;
#14973=PLANE ( 'NONE',  #33250 ) ;
#14983=ORIENTED_EDGE ( 'NONE', *, *, #10937, .F. ) ;
#14989=CARTESIAN_POINT ( 'NONE',  ( 22.89764159710613001, 4.274639749586560455, -77.50000000000000000 ) ) ;
#15018=CARTESIAN_POINT ( 'NONE',  ( 12.46788440507149787, 30.06253867087536946, 49.43553178847298568 ) ) ;
#15027=VECTOR ( 'NONE', #30545, 1000.000000000000000 ) ;
#15028=DIRECTION ( 'NONE',  ( 0.000000000000000000, 1.000000000000000000, 0.000000000000000000 ) ) ;
#15032=CARTESIAN_POINT ( 'NONE',  ( 0.000000000000000000, 2.281450406192313828E-14, -36.69637551990492597 ) ) ;
#15034=PLANE ( 'NONE',  #13270 ) ;
#15040=EDGE_CURVE ( 'NONE', #30310, #10803, #5737, .T. ) ;
#15042=DIRECTION ( 'NONE',  ( 1.000000000000000000, 0.000000000000000000, 0.000000000000000000 ) ) ;
#15054=VERTEX_POINT ( 'NONE', #34973 ) ;
#15059=AXIS2_PLACEMENT_3D ( 'NONE', #24357, #13004, #21694 ) ;
#15064=EDGE_LOOP ( 'NONE', ( #24218, #33058, #24887, #1577 ) ) ;
#15066=VECTOR ( 'NONE', #17676, 1000.000000000000114 ) ;
#15069=PLANE ( 'NONE',  #13522 ) ;
#15076=LINE ( 'NONE', #28243, #9205 ) ;
#15083=ORIENTED_EDGE ( 'NONE', *, *, #20395, .F. ) ;
#15106=VECTOR ( 'NONE', #33707, 1000.000000000000000 ) ;
#15107=EDGE_CURVE ( 'NONE', #12737, #22067, #3429, .T. ) ;
#15108=DIRECTION ( 'NONE',  ( 0.000000000000000000, 1.836970198721029441E-16, -1.000000000000000000 ) ) ;
#15111=DIRECTION ( 'NONE',  ( -0.05413890858541543089, -0.9985334138511240409, -0.000000000000000000 ) ) ;
#15116=ORIENTED_EDGE ( 'NONE', *, *, #20040, .F. ) ;
#15117=VECTOR ( 'NONE', #6781, 1000.000000000000000 ) ;
#15120=EDGE_CURVE ( 'NONE', #12035, #2425, #15432, .T. ) ;
#15121=VERTEX_POINT ( 'NONE', #28361 ) ;
#15126=PLANE ( 'NONE',  #21150 ) ;
#15128=CIRCLE ( 'NONE', #32737, 2.033421858999710619 ) ;
#15132=VECTOR ( 'NONE', #28544, 1000.000000000000000 ) ;
#15138=CARTESIAN_POINT ( 'NONE',  ( 1.532562817202168137, 37.83772838912469894, 68.31122994652405112 ) ) ;
#15145=CIRCLE ( 'NONE', #16863, 2.033421858999711951 ) ;
#15151=ADVANCED_FACE ( 'NONE', ( #3263 ), #28182, .F. ) ;
#15152=AXIS2_PLACEMENT_3D ( 'NONE', #33128, #22284, #8568 ) ;
#15154=DIRECTION ( 'NONE',  ( 1.000000000000000000, 0.000000000000000000, 0.000000000000000000 ) ) ;
#15156=VERTEX_POINT ( 'NONE', #14318 ) ;
#15157=LINE ( 'NONE', #12661, #7188 ) ;
#15160=ORIENTED_EDGE ( 'NONE', *, *, #27574, .F. ) ;
#15162=AXIS2_PLACEMENT_3D ( 'NONE', #32267, #21761, #3066 ) ;
#15166=LINE ( 'NONE', #20327, #848 ) ;
#15170=LINE ( 'NONE', #7129, #33210 ) ;
#15175=ADVANCED_FACE ( 'NONE', ( #8963 ), #6268, .T. ) ;
#15176=VECTOR ( 'NONE', #7456, 1000.000000000000000 ) ;
#15177=ORIENTED_EDGE ( 'NONE', *, *, #29976, .T. ) ;
#15178=ORIENTED_EDGE ( 'NONE', *, *, #12306, .T. ) ;
#15179=ORIENTED_EDGE ( 'NONE', *, *, #679, .F. ) ;
#15190=DIRECTION ( 'NONE',  ( 0.000000000000000000, -1.000000000000000000, 0.000000000000000000 ) ) ;
#15202=CARTESIAN_POINT ( 'NONE',  ( 36.86854689046325717, 8.645963718612074800, 68.31122994652405112 ) ) ;
#15205=ADVANCED_FACE ( 'NONE', ( #14496 ), #3786, .F. ) ;
#15207=VECTOR ( 'NONE', #30725, 1000.000000000000000 ) ;
#15219=VECTOR ( 'NONE', #15240, 1000.000000000000114 ) ;
#15220=ORIENTED_EDGE ( 'NONE', *, *, #6212, .F. ) ;
#15224=EDGE_CURVE ( 'NONE', #32413, #1937, #26194, .T. ) ;
#15225=VECTOR ( 'NONE', #25109, 1000.000000000000114 ) ;
#15227=ORIENTED_EDGE ( 'NONE', *, *, #963, .T. ) ;
#15231=CARTESIAN_POINT ( 'NONE',  ( 1.532562817202168137, 37.83772838912472025, -36.68877005347593467 ) ) ;
#15234=LINE ( 'NONE', #32279, #23615 ) ;
#15236=DIRECTION ( 'NONE',  ( 0.6051742151937656855, -0.7960930657056433102, -1.462399237109729307E-16 ) ) ;
#15238=ORIENTED_EDGE ( 'NONE', *, *, #18413, .F. ) ;
#15240=DIRECTION ( 'NONE',  ( 0.1617819965527638459, 0.9868265225415262520, -0.000000000000000000 ) ) ;
#15246=AXIS2_PLACEMENT_3D ( 'NONE', #34744, #10355, #1995 ) ;
#15252=ORIENTED_EDGE ( 'NONE', *, *, #17596, .T. ) ;
#15257=CARTESIAN_POINT ( 'NONE',  ( 23.93847777447632552, 22.04889236939138897, 68.31122994652405112 ) ) ;
#15264=ORIENTED_EDGE ( 'NONE', *, *, #13623, .T. ) ;
#15265=CARTESIAN_POINT ( 'NONE',  ( -25.63124651156763179, 20.05601094782695526, -36.68877005347593467 ) ) ;
#15268=AXIS2_PLACEMENT_3D ( 'NONE', #1434, #31668, #23159 ) ;
#15273=CARTESIAN_POINT ( 'NONE',  ( -34.66645501699844090, -15.21971901163155216, 68.31122994652405112 ) ) ;
#15283=VECTOR ( 'NONE', #20476, 1000.000000000000000 ) ;
#15288=DIRECTION ( 'NONE',  ( 3.697785493223492838E-32, 1.934419779023891545E-16, -1.000000000000000000 ) ) ;
#15291=LINE ( 'NONE', #4560, #34202 ) ;
#15294=ORIENTED_EDGE ( 'NONE', *, *, #11270, .T. ) ;
#15296=DIRECTION ( 'NONE',  ( 1.000000000000000000, 0.000000000000000000, -0.000000000000000000 ) ) ;
#15297=VERTEX_POINT ( 'NONE', #23022 ) ;
#15300=ORIENTED_EDGE ( 'NONE', *, *, #22301, .T. ) ;
#15301=CARTESIAN_POINT ( 'NONE',  ( -35.00000000000000000, 16.36947364650383818, -36.69637551990492597 ) ) ;
#15307=VERTEX_POINT ( 'NONE', #28534 ) ;
#15313=EDGE_CURVE ( 'NONE', #34550, #1890, #22256, .T. ) ;
#15317=DIRECTION ( 'NONE',  ( 0.000000000000000000, 1.836970198721029688E-16, -1.000000000000000000 ) ) ;
#15325=ORIENTED_EDGE ( 'NONE', *, *, #9605, .F. ) ;
#15336=CARTESIAN_POINT ( 'NONE',  ( 5.021133111224473033, 6.201984591278717041, -67.50000000000000000 ) ) ;
#15339=DIRECTION ( 'NONE',  ( -1.000000000000000000, -0.000000000000000000, -0.000000000000000000 ) ) ;
#15356=EDGE_LOOP ( 'NONE', ( #3051, #15841, #10321, #34386 ) ) ;
#15360=FACE_OUTER_BOUND ( 'NONE', #12342, .T. ) ;
#15368=LINE ( 'NONE', #17698, #10133 ) ;
#15371=CARTESIAN_POINT ( 'NONE',  ( -45.00000000000000000, 3.353962854566122864, -15.81122994652406355 ) ) ;
#15374=CARTESIAN_POINT ( 'NONE',  ( 3.985664461616347742E-15, 32.54542015209057126, 76.74945698428001606 ) ) ;
#15379=DIRECTION ( 'NONE',  ( 0.8854131517428557308, -0.2458337514780907229, 0.3944734685057935120 ) ) ;
#15400=EDGE_CURVE ( 'NONE', #22677, #16274, #22229, .T. ) ;
#15411=ADVANCED_FACE ( 'NONE', ( #25054 ), #3179, .T. ) ;
#15416=CARTESIAN_POINT ( 'NONE',  ( 30.45781707305797070, -22.50252913745434924, 68.31122994652405112 ) ) ;
#15425=ORIENTED_EDGE ( 'NONE', *, *, #20034, .F. ) ;
#15432=CIRCLE ( 'NONE', #67, 2.033421858999711507 ) ;
#15435=CARTESIAN_POINT ( 'NONE',  ( -21.41424479178918361, -24.50784553716280101, 68.31122994652405112 ) ) ;
#15441=VERTEX_POINT ( 'NONE', #30414 ) ;
#15444=VECTOR ( 'NONE', #8933, 1000.000000000000000 ) ;
#15451=EDGE_CURVE ( 'NONE', #27734, #30712, #22056, .T. ) ;
#15452=VERTEX_POINT ( 'NONE', #8521 ) ;
#15453=ORIENTED_EDGE ( 'NONE', *, *, #26320, .F. ) ;
#15455=DIRECTION ( 'NONE',  ( 1.000000000000000000, 0.000000000000000000, 0.000000000000000000 ) ) ;
#15457=DIRECTION ( 'NONE',  ( 0.000000000000000000, 1.836970198721029441E-16, -1.000000000000000000 ) ) ;
#15460=PLANE ( 'NONE',  #30648 ) ;
#15472=AXIS2_PLACEMENT_3D ( 'NONE', #2498, #5683, #2850 ) ;
#15480=CARTESIAN_POINT ( 'NONE',  ( 21.24400529595485310, -24.65555945140048522, 68.31122994652405112 ) ) ;
#15485=EDGE_LOOP ( 'NONE', ( #25033, #5935, #17385, #19724 ) ) ;
#15487=VERTEX_POINT ( 'NONE', #6550 ) ;
#15488=DIRECTION ( 'NONE',  ( 0.000000000000000000, 1.836970198721029441E-16, -1.000000000000000000 ) ) ;
#15498=DIRECTION ( 'NONE',  ( 0.6876994588534236508, 0.7259954919231305093, -0.000000000000000000 ) ) ;
#15502=ORIENTED_EDGE ( 'NONE', *, *, #31570, .T. ) ;
#15505=PLANE ( 'NONE',  #11806 ) ;
#15506=CARTESIAN_POINT ( 'NONE',  ( -29.68486519896224962, 23.49918569563710946, 68.31122994652405112 ) ) ;
#15510=CARTESIAN_POINT ( 'NONE',  ( 22.89764159710611224, 13.56412600238610366, -77.50000000000000000 ) ) ;
#15513=VECTOR ( 'NONE', #16745, 1000.000000000000000 ) ;
#15517=CARTESIAN_POINT ( 'NONE',  ( -5.021133111224782120, 16.12922284503173742, -67.50000000000000000 ) ) ;
#15527=EDGE_LOOP ( 'NONE', ( #28302, #25889, #30640, #27497 ) ) ;
#15533=CARTESIAN_POINT ( 'NONE',  ( 0.000000000000000000, 3.524919873834583163E-15, 68.31122994652405112 ) ) ;
#15539=DIRECTION ( 'NONE',  ( 0.05413890858541543089, 0.9985334138511240409, 0.000000000000000000 ) ) ;
#15550=DIRECTION ( 'NONE',  ( -1.000000000000000000, 0.000000000000000000, 0.000000000000000000 ) ) ;
#15552=CARTESIAN_POINT ( 'NONE',  ( 20.62763069236413926, -31.74750072459299588, 49.43553178847298568 ) ) ;
#15555=AXIS2_PLACEMENT_3D ( 'NONE', #12714, #21051, #15737 ) ;
#15557=ORIENTED_EDGE ( 'NONE', *, *, #9565, .F. ) ;
#15568=VERTEX_POINT ( 'NONE', #22934 ) ;
#15579=ORIENTED_EDGE ( 'NONE', *, *, #17357, .T. ) ;
#15580=DIRECTION ( 'NONE',  ( -0.6876994588534225405, 0.7259954919231316195, 0.000000000000000000 ) ) ;
#15582=CARTESIAN_POINT ( 'NONE',  ( 0.000000000000000000, 3.524919873834583163E-15, 68.31122994652405112 ) ) ;
#15583=DIRECTION ( 'NONE',  ( 0.000000000000000000, 0.8486862100397269959, -0.5288966977476834419 ) ) ;
#15603=DIRECTION ( 'NONE',  ( 0.000000000000000000, 1.836970198721029441E-16, -1.000000000000000000 ) ) ;
#15607=CARTESIAN_POINT ( 'NONE',  ( 0.000000000000000000, 45.00000000000000711, -36.68877005347592757 ) ) ;
#15614=VECTOR ( 'NONE', #7275, 1000.000000000000000 ) ;
#15615=EDGE_CURVE ( 'NONE', #10302, #9321, #27912, .T. ) ;
#15617=EDGE_CURVE ( 'NONE', #7575, #17615, #3705, .T. ) ;
#15621=VECTOR ( 'NONE', #8231, 1000.000000000000227 ) ;
#15622=EDGE_LOOP ( 'NONE', ( #5656, #28162, #4355, #30797 ) ) ;
#15624=EDGE_LOOP ( 'NONE', ( #17477, #16785, #33173, #29986 ) ) ;
#15632=VERTEX_POINT ( 'NONE', #10101 ) ;
#15636=CARTESIAN_POINT ( 'NONE',  ( -9.978866888775632660, -5.758675521474011738, -87.50000000000000000 ) ) ;
#15641=VECTOR ( 'NONE', #5097, 1000.000000000000000 ) ;
#15642=DIRECTION ( 'NONE',  ( 0.000000000000000000, 0.000000000000000000, 1.000000000000000000 ) ) ;
#15649=DIRECTION ( 'NONE',  ( 0.000000000000000000, 1.836970198721029441E-16, -1.000000000000000000 ) ) ;
#15651=DIRECTION ( 'NONE',  ( 0.000000000000000000, -0.5288966977476834419, 0.8486862100397269959 ) ) ;
#15657=EDGE_CURVE ( 'NONE', #18691, #2115, #29328, .T. ) ;
#15669=CARTESIAN_POINT ( 'NONE',  ( 0.000000000000000000, 3.524919873834583163E-15, 68.31122994652405112 ) ) ;
#15670=CARTESIAN_POINT ( 'NONE',  ( 0.000000000000000000, -33.69708579775584667, 49.43553178847298568 ) ) ;
#15675=PLANE ( 'NONE',  #1615 ) ;
#15682=EDGE_CURVE ( 'NONE', #20094, #27049, #20787, .T. ) ;
#15685=CARTESIAN_POINT ( 'NONE',  ( -34.04247984038124031, 16.56841925338180488, 68.31122994652405112 ) ) ;
#15689=CARTESIAN_POINT ( 'NONE',  ( -23.78520691327551972, 22.21414650552150860, -36.68877005347593467 ) ) ;
#15690=ORIENTED_EDGE ( 'NONE', *, *, #20572, .T. ) ;
#15692=LINE ( 'NONE', #23330, #27094 ) ;
#15693=ORIENTED_EDGE ( 'NONE', *, *, #3556, .F. ) ;
#15694=VECTOR ( 'NONE', #24097, 1000.000000000000000 ) ;
#15696=CARTESIAN_POINT ( 'NONE',  ( 28.11866956577617316, 16.38733641342591341, 49.43553178847298568 ) ) ;
#15698=CARTESIAN_POINT ( 'NONE',  ( 22.89764159710615132, -1.579009122040560431, -87.50000000000000000 ) ) ;
#15699=EDGE_CURVE ( 'NONE', #10968, #2751, #9776, .T. ) ;
#15700=ADVANCED_FACE ( 'NONE', ( #7771 ), #15817, .F. ) ;
#15709=VECTOR ( 'NONE', #21614, 1000.000000000000114 ) ;
#15714=FACE_OUTER_BOUND ( 'NONE', #33873, .T. ) ;
#15720=PLANE ( 'NONE',  #15246 ) ;
#15733=DIRECTION ( 'NONE',  ( 0.000000000000000000, 1.836970198721029441E-16, -1.000000000000000000 ) ) ;
#15735=EDGE_CURVE ( 'NONE', #28091, #2086, #31911, .T. ) ;
#15737=DIRECTION ( 'NONE',  ( 1.000000000000000000, 0.000000000000000000, 0.000000000000000000 ) ) ;
#15743=ORIENTED_EDGE ( 'NONE', *, *, #17297, .T. ) ;
#15744=LINE ( 'NONE', #34597, #19029 ) ;
#15745=FACE_OUTER_BOUND ( 'NONE', #21103, .T. ) ;
#15750=EDGE_CURVE ( 'NONE', #19356, #31410, #20501, .T. ) ;
#15751=AXIS2_PLACEMENT_3D ( 'NONE', #9685, #26752, #4498 ) ;
#15758=AXIS2_PLACEMENT_3D ( 'NONE', #6418, #28149, #1098 ) ;
#15761=VECTOR ( 'NONE', #15498, 1000.000000000000114 ) ;
#15765=ORIENTED_EDGE ( 'NONE', *, *, #12117, .T. ) ;
#15768=DIRECTION ( 'NONE',  ( 0.000000000000000000, 1.000000000000000000, 0.000000000000000000 ) ) ;
#15779=DIRECTION ( 'NONE',  ( -0.9075754196709575616, -0.4198891015602634891, -0.000000000000000000 ) ) ;
#15782=DIRECTION ( 'NONE',  ( 0.000000000000000000, 1.836970198721029441E-16, -1.000000000000000000 ) ) ;
#15796=DIRECTION ( 'NONE',  ( -0.000000000000000000, 1.000000000000000000, 0.000000000000000000 ) ) ;
#15797=ORIENTED_EDGE ( 'NONE', *, *, #7976, .F. ) ;
#15808=AXIS2_PLACEMENT_3D ( 'NONE', #19882, #6320, #17224 ) ;
#15816=CARTESIAN_POINT ( 'NONE',  ( -37.85301660235036536, 0.7430237821112669616, 15.81122994652406355 ) ) ;
#15817=CYLINDRICAL_SURFACE ( 'NONE', #2371, 2.033421858999711951 ) ;
#15829=ORIENTED_EDGE ( 'NONE', *, *, #3471, .T. ) ;
#15833=CARTESIAN_POINT ( 'NONE',  ( 0.000000000000000000, 45.00000000000000711, -36.68877005347592757 ) ) ;
#15835=ORIENTED_EDGE ( 'NONE', *, *, #27607, .T. ) ;
#15839=ORIENTED_EDGE ( 'NONE', *, *, #7181, .T. ) ;
#15841=ORIENTED_EDGE ( 'NONE', *, *, #19614, .T. ) ;
#15857=PLANE ( 'NONE',  #10527 ) ;
#15861=ORIENTED_EDGE ( 'NONE', *, *, #17553, .F. ) ;
#15864=DIRECTION ( 'NONE',  ( 0.000000000000000000, -1.000000000000000000, -2.132064625830773463E-16 ) ) ;
#15872=LINE ( 'NONE', #4144, #22880 ) ;
#15876=DIRECTION ( 'NONE',  ( 0.000000000000000000, 1.836970198721029688E-16, -1.000000000000000000 ) ) ;
#15877=CARTESIAN_POINT ( 'NONE',  ( -5.021133111224679091, 28.08988295778447508, -67.50000000000000000 ) ) ;
#15878=ADVANCED_FACE ( 'NONE', ( #11342 ), #479, .F. ) ;
#15880=VECTOR ( 'NONE', #8311, 1000.000000000000000 ) ;
#15881=PLANE ( 'NONE',  #5952 ) ;
#15889=EDGE_CURVE ( 'NONE', #32399, #14788, #27697, .T. ) ;
#15892=VERTEX_POINT ( 'NONE', #10637 ) ;
#15903=ORIENTED_EDGE ( 'NONE', *, *, #10444, .T. ) ;
#15906=EDGE_CURVE ( 'NONE', #18186, #20191, #24315, .T. ) ;
#15916=VECTOR ( 'NONE', #21086, 1000.000000000000114 ) ;
#15919=FACE_OUTER_BOUND ( 'NONE', #28515, .T. ) ;
#15921=LINE ( 'NONE', #11269, #19665 ) ;
#15938=ORIENTED_EDGE ( 'NONE', *, *, #11713, .F. ) ;
#15942=DIRECTION ( 'NONE',  ( 0.000000000000000000, 1.836970198721029441E-16, -1.000000000000000000 ) ) ;
#15944=ORIENTED_EDGE ( 'NONE', *, *, #4343, .F. ) ;
#15946=CARTESIAN_POINT ( 'NONE',  ( -37.12776225901827587, -7.411627343331143258, -17.41927665145495041 ) ) ;
#15954=DIRECTION ( 'NONE',  ( 1.000000000000000000, 0.000000000000000000, -0.000000000000000000 ) ) ;
#15957=CARTESIAN_POINT ( 'NONE',  ( -10.00000000000000000, 3.520859547548641820E-15, 87.50000000000000000 ) ) ;
#15959=CARTESIAN_POINT ( 'NONE',  ( -5.021133111224679091, 24.02303923978504940, -67.50000000000000000 ) ) ;
#15963=EDGE_CURVE ( 'NONE', #15487, #29615, #34781, .T. ) ;
#15974=DIRECTION ( 'NONE',  ( -0.000000000000000000, 1.836970198721029934E-16, -1.000000000000000000 ) ) ;
#15975=LINE ( 'NONE', #10263, #5606 ) ;
#15984=DIRECTION ( 'NONE',  ( 1.000000000000000000, 0.000000000000000000, -0.000000000000000000 ) ) ;
#15985=DIRECTION ( 'NONE',  ( 0.000000000000000000, 1.000000000000000000, 0.000000000000000000 ) ) ;
#15989=CARTESIAN_POINT ( 'NONE',  ( -13.53398258527560749, -35.36769364574539765, 68.31122994652405112 ) ) ;
#15990=EDGE_LOOP ( 'NONE', ( #14925, #331, #20416, #32208 ) ) ;
#15996=DIRECTION ( 'NONE',  ( 0.000000000000000000, 1.836970198721029688E-16, -1.000000000000000000 ) ) ;
#16007=PRODUCT_DEFINITION ( 'UNKNOWN', '', #16149, #4991 ) ;
#16013=LINE ( 'NONE', #26848, #5310 ) ;
#16022=ORIENTED_EDGE ( 'NONE', *, *, #32930, .T. ) ;
#16024=DIRECTION ( 'NONE',  ( 0.000000000000000000, -1.836970198721029688E-16, 1.000000000000000000 ) ) ;
#16033=VECTOR ( 'NONE', #24019, 1000.000000000000000 ) ;
#16035=LINE ( 'NONE', #26869, #14889 ) ;
#16038=DIRECTION ( 'NONE',  ( 0.000000000000000000, 1.000000000000000000, 0.000000000000000000 ) ) ;
#16039=EDGE_LOOP ( 'NONE', ( #16459, #19268, #8688, #24721 ) ) ;
#16040=DIRECTION ( 'NONE',  ( 0.000000000000000000, 0.000000000000000000, 1.000000000000000000 ) ) ;
#16042=EDGE_CURVE ( 'NONE', #20191, #22259, #24461, .T. ) ;
#16043=AXIS2_PLACEMENT_3D ( 'NONE', #16514, #22188, #27340 ) ;
#16044=FACE_OUTER_BOUND ( 'NONE', #28763, .T. ) ;
#16061=VERTEX_POINT ( 'NONE', #20235 ) ;
#16070=VERTEX_POINT ( 'NONE', #20749 ) ;
#16071=CARTESIAN_POINT ( 'NONE',  ( 26.97014235612466493, -26.57093094961043533, 49.43553178847298568 ) ) ;
#16077=AXIS2_PLACEMENT_3D ( 'NONE', #3685, #7523, #23564 ) ;
#16079=LINE ( 'NONE', #18225, #29327 ) ;
#16083=CIRCLE ( 'NONE', #725, 32.54542015209056416 ) ;
#16087=CARTESIAN_POINT ( 'NONE',  ( 25.76952721012208158, 19.87802405277947670, 49.43553178847298568 ) ) ;
#16091=DIRECTION ( 'NONE',  ( 0.000000000000000000, 0.000000000000000000, -1.000000000000000000 ) ) ;
#16104=DIRECTION ( 'NONE',  ( -0.000000000000000000, -1.836970198721029688E-16, 1.000000000000000000 ) ) ;
#16105=ORIENTED_EDGE ( 'NONE', *, *, #634, .F. ) ;
#16106=ORIENTED_EDGE ( 'NONE', *, *, #32984, .T. ) ;
#16117=DIRECTION ( 'NONE',  ( -0.000000000000000000, 0.5288966977476834419, -0.8486862100397269959 ) ) ;
#16120=DIRECTION ( 'NONE',  ( 0.2149704402110236556, 0.9766205557100866574, -0.000000000000000000 ) ) ;
#16125=EDGE_CURVE ( 'NONE', #26960, #15297, #5709, .T. ) ;
#16132=AXIS2_PLACEMENT_3D ( 'NONE', #11432, #19976, #30826 ) ;
#16133=DIRECTION ( 'NONE',  ( 0.000000000000000000, -1.000000000000000000, -1.836970198721029441E-16 ) ) ;
#16149=PRODUCT_DEFINITION_FORMATION_WITH_SPECIFIED_SOURCE ( 'ANY', '', #22877, .NOT_KNOWN. ) ;
#16159=PLANE ( 'NONE',  #10086 ) ;
#16162=EDGE_CURVE ( 'NONE', #2097, #32385, #31423, .T. ) ;
#16166=DIRECTION ( 'NONE',  ( 1.000000000000000000, 0.000000000000000000, 0.000000000000000000 ) ) ;
#16169=CARTESIAN_POINT ( 'NONE',  ( 32.30227131129396412, -3.970848902647434286, 49.43553178847298568 ) ) ;
#16170=DIRECTION ( 'NONE',  ( -1.000000000000000000, 0.000000000000000000, 0.000000000000000000 ) ) ;
#16171=ORIENTED_EDGE ( 'NONE', *, *, #7704, .T. ) ;
#16178=CARTESIAN_POINT ( 'NONE',  ( 5.021133111224369117, -5.758675521474011738, -87.50000000000000000 ) ) ;
#16181=ORIENTED_EDGE ( 'NONE', *, *, #18732, .F. ) ;
#16183=LINE ( 'NONE', #32878, #4628 ) ;
#16186=AXIS2_PLACEMENT_3D ( 'NONE', #243, #13772, #16279 ) ;
#16196=CARTESIAN_POINT ( 'NONE',  ( 0.000000000000000000, 3.524919873834583163E-15, 68.31122994652405112 ) ) ;
#16198=ORIENTED_EDGE ( 'NONE', *, *, #2202, .F. ) ;
#16210=VERTEX_POINT ( 'NONE', #34622 ) ;
#16213=EDGE_LOOP ( 'NONE', ( #19863, #3185, #27201, #18533 ) ) ;
#16228=DIRECTION ( 'NONE',  ( 0.000000000000000000, 0.000000000000000000, 1.000000000000000000 ) ) ;
#16231=ORIENTED_EDGE ( 'NONE', *, *, #31224, .F. ) ;
#16238=CARTESIAN_POINT ( 'NONE',  ( -8.267476927982267298, 31.47782073335737962, -36.68877005347593467 ) ) ;
#16239=SHAPE_DEFINITION_REPRESENTATION ( #33659, #30518 ) ;
#16242=LINE ( 'NONE', #21916, #13951 ) ;
#16249=ORIENTED_EDGE ( 'NONE', *, *, #22022, .F. ) ;
#16250=DIRECTION ( 'NONE',  ( 0.7259954919231307313, 0.6876994588534234287, -0.000000000000000000 ) ) ;
#16252=EDGE_CURVE ( 'NONE', #4259, #1639, #32457, .T. ) ;
#16254=DIRECTION ( 'NONE',  ( 0.000000000000000000, 0.000000000000000000, 1.000000000000000000 ) ) ;
#16256=DIRECTION ( 'NONE',  ( -0.4684084406997900407, 0.8835120444460229372, 1.622985295858433783E-16 ) ) ;
#16266=DIRECTION ( 'NONE',  ( 0.000000000000000000, 1.836970198721029441E-16, -1.000000000000000000 ) ) ;
#16268=CARTESIAN_POINT ( 'NONE',  ( 37.71145559917817280, 3.353962854566119756, 68.31122994652405112 ) ) ;
#16273=AXIS2_PLACEMENT_3D ( 'NONE', #14499, #27477, #19663 ) ;
#16274=VERTEX_POINT ( 'NONE', #18959 ) ;
#16275=CARTESIAN_POINT ( 'NONE',  ( 35.63428259149704758, -12.79065496477508823, 49.43553178847298568 ) ) ;
#16278=ORIENTED_EDGE ( 'NONE', *, *, #28453, .T. ) ;
#16279=DIRECTION ( 'NONE',  ( 0.000000000000000000, -1.836970198721029688E-16, 1.000000000000000000 ) ) ;
#16287=CIRCLE ( 'NONE', #3182, 32.54542015209054995 ) ;
#16288=VERTEX_POINT ( 'NONE', #29802 ) ;
#16290=CARTESIAN_POINT ( 'NONE',  ( 5.021133111224265200, -13.65249191622732816, -67.50000000000000000 ) ) ;
#16292=EDGE_CURVE ( 'NONE', #1376, #32413, #30145, .T. ) ;
#16297=AXIS2_PLACEMENT_3D ( 'NONE', #3396, #27434, #33307 ) ;
#16303=VECTOR ( 'NONE', #8089, 1000.000000000000000 ) ;
#16313=CARTESIAN_POINT ( 'NONE',  ( 22.10765473302597073, -12.47301499840863848, -87.50000000000000000 ) ) ;
#16318=CARTESIAN_POINT ( 'NONE',  ( -26.18205399241665177, -19.33143609808334418, -36.68877005347593467 ) ) ;
#16320=VERTEX_POINT ( 'NONE', #8439 ) ;
#16321=ADVANCED_FACE ( 'NONE', ( #24439 ), #21971, .T. ) ;
#16323=EDGE_CURVE ( 'NONE', #33860, #5983, #29979, .T. ) ;
#16324=ORIENTED_EDGE ( 'NONE', *, *, #3450, .T. ) ;
#16327=ORIENTED_EDGE ( 'NONE', *, *, #24601, .F. ) ;
#16331=CARTESIAN_POINT ( 'NONE',  ( 3.235562306570555532E-30, -11.61907005722761532, -67.50000000000000000 ) ) ;
#16332=DIRECTION ( 'NONE',  ( 0.000000000000000000, 1.836970198721029441E-16, -1.000000000000000000 ) ) ;
#16333=ORIENTED_EDGE ( 'NONE', *, *, #3162, .F. ) ;
#16359=VECTOR ( 'NONE', #25194, 1000.000000000000227 ) ;
#16367=EDGE_LOOP ( 'NONE', ( #9064, #6563, #19397, #4294 ) ) ;
#16378=CARTESIAN_POINT ( 'NONE',  ( -37.58721499952019940, -4.609089608337754385, 68.31122994652405112 ) ) ;
#16382=ORIENTED_EDGE ( 'NONE', *, *, #8142, .T. ) ;
#16387=CARTESIAN_POINT ( 'NONE',  ( 25.76952721012208158, 19.87802405277947315, 68.31122994652405112 ) ) ;
#16392=FACE_OUTER_BOUND ( 'NONE', #34434, .T. ) ;
#16402=CYLINDRICAL_SURFACE ( 'NONE', #14434, 44.99999999999997868 ) ;
#16415=ORIENTED_EDGE ( 'NONE', *, *, #14773, .T. ) ;
#16416=ORIENTED_EDGE ( 'NONE', *, *, #1104, .F. ) ;
#16420=EDGE_LOOP ( 'NONE', ( #31507, #31502, #9897, #34554, #30344, #4734, #26971, #3976 ) ) ;
#16421=DIRECTION ( 'NONE',  ( 1.204656189240283493E-16, 0.9836764282395641379, 0.1799463379062031521 ) ) ;
#16425=ORIENTED_EDGE ( 'NONE', *, *, #33309, .F. ) ;
#16427=CARTESIAN_POINT ( 'NONE',  ( 10.17231796313409298, 6.310691531022070144, -77.50000000000000000 ) ) ;
#16433=VECTOR ( 'NONE', #21659, 1000.000000000000000 ) ;
#16434=CARTESIAN_POINT ( 'NONE',  ( -36.47450208408277916, 26.16822801941811605, 52.41980080743829973 ) ) ;
#16437=CARTESIAN_POINT ( 'NONE',  ( -2.791255079241054649, -37.75727539589166071, 68.31122994652405112 ) ) ;
#16443=CYLINDRICAL_SURFACE ( 'NONE', #5325, 2.033421858999711951 ) ;
#16445=CARTESIAN_POINT ( 'NONE',  ( -36.90749871141738936, 3.535880188965249360, 16.10314088816767253 ) ) ;
#16452=LINE ( 'NONE', #16275, #19474 ) ;
#16456=VERTEX_POINT ( 'NONE', #33523 ) ;
#16459=ORIENTED_EDGE ( 'NONE', *, *, #29849, .T. ) ;
#16461=EDGE_CURVE ( 'NONE', #31033, #34772, #3437, .T. ) ;
#16468=LINE ( 'NONE', #25150, #27739 ) ;
#16474=DIRECTION ( 'NONE',  ( 0.000000000000000000, 1.836970198721029441E-16, -1.000000000000000000 ) ) ;
#16475=ORIENTED_EDGE ( 'NONE', *, *, #15451, .F. ) ;
#16477=CARTESIAN_POINT ( 'NONE',  ( 34.58310883014599568, -15.42890216704097206, 68.31122994652405112 ) ) ;
#16483=CARTESIAN_POINT ( 'NONE',  ( -45.00000000000000000, -46.95407462254104303, 36.69637551990492597 ) ) ;
#16484=ORIENTED_EDGE ( 'NONE', *, *, #21002, .T. ) ;
#16500=CARTESIAN_POINT ( 'NONE',  ( 0.000000000000000000, 3.524919873834583163E-15, 68.31122994652405112 ) ) ;
#16501=EDGE_LOOP ( 'NONE', ( #27535, #11283, #21773, #10005 ) ) ;
#16503=LINE ( 'NONE', #30179, #21837 ) ;
#16506=DIRECTION ( 'NONE',  ( -0.000000000000000000, -1.836970198721029688E-16, 1.000000000000000000 ) ) ;
#16507=DIRECTION ( 'NONE',  ( -0.1081190184239421148, 0.9941379571543595972, -0.000000000000000000 ) ) ;
#16508=FACE_OUTER_BOUND ( 'NONE', #10556, .T. ) ;
#16510=ORIENTED_EDGE ( 'NONE', *, *, #9500, .T. ) ;
#16513=DIRECTION ( 'NONE',  ( 0.6051742151937650194, 0.7960930657056437543, 0.000000000000000000 ) ) ;
#16514=CARTESIAN_POINT ( 'NONE',  ( -9.410814080250917257, 36.67205378194064735, 68.31122994652405112 ) ) ;
#16515=CARTESIAN_POINT ( 'NONE',  ( 22.89764159710613001, 4.274639749586562232, -87.50000000000000000 ) ) ;
#16518=CARTESIAN_POINT ( 'NONE',  ( 0.000000000000000000, 2.281310696040539424E-14, -36.68877005347592757 ) ) ;
#16530=ORIENTED_EDGE ( 'NONE', *, *, #3369, .T. ) ;
#16537=EDGE_CURVE ( 'NONE', #32615, #26158, #18056, .T. ) ;
#16538=EDGE_CURVE ( 'NONE', #25782, #26683, #29237, .T. ) ;
#16540=VECTOR ( 'NONE', #34020, 1000.000000000000000 ) ;
#16543=DIRECTION ( 'NONE',  ( -0.7621620551276372391, 0.6473862847818266930, 0.000000000000000000 ) ) ;
#16553=DIRECTION ( 'NONE',  ( 0.000000000000000000, 0.000000000000000000, 1.000000000000000000 ) ) ;
#16555=CARTESIAN_POINT ( 'NONE',  ( 15.04122381213380599, 28.86114964982168019, 49.43553178847298568 ) ) ;
#16556=VERTEX_POINT ( 'NONE', #2004 ) ;
#16559=ORIENTED_EDGE ( 'NONE', *, *, #28844, .T. ) ;
#16562=DIRECTION ( 'NONE',  ( 3.697785493223492838E-32, 1.934419779023891545E-16, -1.000000000000000000 ) ) ;
#16563=ORIENTED_EDGE ( 'NONE', *, *, #22304, .T. ) ;
#16571=LINE ( 'NONE', #11572, #30848 ) ;
#16577=CARTESIAN_POINT ( 'NONE',  ( -5.021133111225196011, -25.61315202898006049, -67.50000000000000000 ) ) ;
#16579=CARTESIAN_POINT ( 'NONE',  ( 21.24400529595486020, -24.65555945140047811, 49.43553178847298568 ) ) ;
#16583=EDGE_CURVE ( 'NONE', #23102, #31704, #31209, .T. ) ;
#16584=CARTESIAN_POINT ( 'NONE',  ( 32.30227131129396412, -3.970848902647434286, 49.43553178847298568 ) ) ;
#16593=AXIS2_PLACEMENT_3D ( 'NONE', #21996, #24641, #22527 ) ;
#16600=LINE ( 'NONE', #30642, #4902 ) ;
#16604=DIRECTION ( 'NONE',  ( 0.000000000000000000, 0.000000000000000000, 1.000000000000000000 ) ) ;
#16608=ADVANCED_FACE ( 'NONE', ( #6986 ), #34754, .F. ) ;
#16612=CARTESIAN_POINT ( 'NONE',  ( 15.04122381213380244, 28.86114964982166597, 68.31122994652405112 ) ) ;
#16617=VECTOR ( 'NONE', #33631, 1000.000000000000000 ) ;
#16623=FACE_OUTER_BOUND ( 'NONE', #17967, .T. ) ;
#16624=VECTOR ( 'NONE', #3543, 1000.000000000000000 ) ;
#16627=VERTEX_POINT ( 'NONE', #20362 ) ;
#16629=EDGE_LOOP ( 'NONE', ( #5967, #30196, #26164, #30298 ) ) ;
#16630=ORIENTED_EDGE ( 'NONE', *, *, #13001, .T. ) ;
#16637=LINE ( 'NONE', #22139, #13534 ) ;
#16639=CARTESIAN_POINT ( 'NONE',  ( -2.216215597024039141, -32.46987467335852529, 68.31122994652405112 ) ) ;
#16652=LINE ( 'NONE', #27835, #26113 ) ;
#16653=ORIENTED_EDGE ( 'NONE', *, *, #14689, .T. ) ;
#16660=ORIENTED_EDGE ( 'NONE', *, *, #17905, .T. ) ;
#16670=ORIENTED_EDGE ( 'NONE', *, *, #33309, .T. ) ;
#16672=VERTEX_POINT ( 'NONE', #12705 ) ;
#16674=FACE_OUTER_BOUND ( 'NONE', #3601, .T. ) ;
#16675=VERTEX_POINT ( 'NONE', #5012 ) ;
#16679=CARTESIAN_POINT ( 'NONE',  ( 0.000000000000000000, -33.69708579775584667, 49.43553178847298568 ) ) ;
#16685=DIRECTION ( 'NONE',  ( 0.000000000000000000, 1.000000000000000000, 0.000000000000000000 ) ) ;
#16686=DIRECTION ( 'NONE',  ( -0.5611870653623813876, 0.8276889981568912313, 0.000000000000000000 ) ) ;
#16696=EDGE_CURVE ( 'NONE', #5869, #16070, #215, .T. ) ;
#16697=CARTESIAN_POINT ( 'NONE',  ( 10.17231796313407344, -3.615060903476078114, -87.50000000000000000 ) ) ;
#16706=ADVANCED_FACE ( 'NONE', ( #10897 ), #5533, .F. ) ;
#16707=ADVANCED_FACE ( 'NONE', ( #2523 ), #13402, .F. ) ;
#16713=ORIENTED_EDGE ( 'NONE', *, *, #14063, .F. ) ;
#16715=AXIS2_PLACEMENT_3D ( 'NONE', #14517, #979, #15042 ) ;
#16724=ORIENTED_EDGE ( 'NONE', *, *, #20395, .T. ) ;
#16727=ORIENTED_EDGE ( 'NONE', *, *, #3485, .F. ) ;
#16741=VERTEX_POINT ( 'NONE', #5704 ) ;
#16745=DIRECTION ( 'NONE',  ( 0.000000000000000000, 1.836970198721029441E-16, -1.000000000000000000 ) ) ;
#16747=CARTESIAN_POINT ( 'NONE',  ( 17.88561705399011714, -27.19023860642122514, 68.31122994652405112 ) ) ;
#16749=AXIS2_PLACEMENT_3D ( 'NONE', #29963, #5911, #5730 ) ;
#16751=LINE ( 'NONE', #27936, #6600 ) ;
#16757=ORIENTED_EDGE ( 'NONE', *, *, #6456, .F. ) ;
#16765=EDGE_CURVE ( 'NONE', #24033, #17068, #5177, .T. ) ;
#16774=VECTOR ( 'NONE', #8865, 1000.000000000000227 ) ;
#16785=ORIENTED_EDGE ( 'NONE', *, *, #7254, .F. ) ;
#16804=CARTESIAN_POINT ( 'NONE',  ( 6.857172176539690689, 37.23415287044793587, 68.31122994652405112 ) ) ;
#16805=( LENGTH_UNIT ( ) NAMED_UNIT ( * ) SI_UNIT ( .MILLI., .METRE. ) );
#16815=FACE_BOUND ( 'NONE', #32897, .T. ) ;
#16819=AXIS2_PLACEMENT_3D ( 'NONE', #9375, #31088, #28414 ) ;
#16827=VECTOR ( 'NONE', #2452, 1000.000000000000000 ) ;
#16828=FACE_OUTER_BOUND ( 'NONE', #17687, .T. ) ;
#16829=ADVANCED_FACE ( 'NONE', ( #6233 ), #14282, .F. ) ;
#16832=LINE ( 'NONE', #22321, #18170 ) ;
#16835=DIRECTION ( 'NONE',  ( 0.000000000000000000, 1.836970198721029441E-16, -1.000000000000000000 ) ) ;
#16838=CARTESIAN_POINT ( 'NONE',  ( 29.82459402470849952, -33.69708579775585378, -36.68877005347594888 ) ) ;
#16839=DIRECTION ( 'NONE',  ( -0.000000000000000000, 1.836970198721029934E-16, -1.000000000000000000 ) ) ;
#16843=DIRECTION ( 'NONE',  ( 0.000000000000000000, 1.836970198721029441E-16, -1.000000000000000000 ) ) ;
#16854=ADVANCED_FACE ( 'NONE', ( #741 ), #19444, .F. ) ;
#16855=ADVANCED_FACE ( 'NONE', ( #8923 ), #30281, .F. ) ;
#16861=DIRECTION ( 'NONE',  ( 0.000000000000000000, 0.000000000000000000, 1.000000000000000000 ) ) ;
#16863=AXIS2_PLACEMENT_3D ( 'NONE', #8393, #5699, #30106 ) ;
#16865=CARTESIAN_POINT ( 'NONE',  ( 37.71145559917817280, 3.353962854566119756, 68.31122994652405112 ) ) ;
#16867=ORIENTED_EDGE ( 'NONE', *, *, #10312, .T. ) ;
#16868=DIRECTION ( 'NONE',  ( -0.8276889981568902321, -0.5611870653623829419, 0.000000000000000000 ) ) ;
#16870=LINE ( 'NONE', #27695, #16359 ) ;
#16874=LINE ( 'NONE', #19531, #29858 ) ;
#16876=CARTESIAN_POINT ( 'NONE',  ( -9.978866888775426602, 18.16264470403145026, -67.50000000000000000 ) ) ;
#16881=CARTESIAN_POINT ( 'NONE',  ( 0.000000000000000000, -33.69708579775585378, -36.68877005347594178 ) ) ;
#16886=DIRECTION ( 'NONE',  ( 0.000000000000000000, 1.836970198721029441E-16, -1.000000000000000000 ) ) ;
#16894=ORIENTED_EDGE ( 'NONE', *, *, #1262, .T. ) ;
#16901=DIRECTION ( 'NONE',  ( 0.000000000000000000, 0.000000000000000000, 1.000000000000000000 ) ) ;
#16903=CARTESIAN_POINT ( 'NONE',  ( -41.91706493227329133, 16.36947364650383818, -36.69637551990492597 ) ) ;
#16919=CARTESIAN_POINT ( 'NONE',  ( -35.00000000000000000, 3.432458613951609561, -15.93718699791188342 ) ) ;
#16920=DIRECTION ( 'NONE',  ( -0.000000000000000000, 1.836970198721029934E-16, -1.000000000000000000 ) ) ;
#16921=VERTEX_POINT ( 'NONE', #6493 ) ;
#16922=VERTEX_POINT ( 'NONE', #146 ) ;
#16923=LINE ( 'NONE', #3365, #4371 ) ;
#16925=LINE ( 'NONE', #21887, #32534 ) ;
#16930=LINE ( 'NONE', #27757, #24209 ) ;
#16934=DIRECTION ( 'NONE',  ( 0.000000000000000000, 1.000000000000000000, 0.000000000000000000 ) ) ;
#16939=ORIENTED_EDGE ( 'NONE', *, *, #2238, .T. ) ;
#16944=VERTEX_POINT ( 'NONE', #24174 ) ;
#16948=EDGE_CURVE ( 'NONE', #8902, #32774, #27027, .T. ) ;
#16950=EDGE_CURVE ( 'NONE', #6786, #20123, #24511, .T. ) ;
#16966=CARTESIAN_POINT ( 'NONE',  ( 36.10877985260814427, 11.38239727801116352, 68.31122994652405112 ) ) ;
#16970=DIRECTION ( 'NONE',  ( 0.000000000000000000, 1.836970198721029688E-16, -1.000000000000000000 ) ) ;
#16971=ORIENTED_EDGE ( 'NONE', *, *, #22413, .F. ) ;
#16974=PLANE ( 'NONE',  #5274 ) ;
#16983=VECTOR ( 'NONE', #30639, 1000.000000000000000 ) ;
#16985=ORIENTED_EDGE ( 'NONE', *, *, #33829, .T. ) ;
#16988=EDGE_CURVE ( 'NONE', #25253, #8062, #786, .T. ) ;
#16992=EDGE_LOOP ( 'NONE', ( #11684, #14544, #13169, #3529 ) ) ;
#16993=ORIENTED_EDGE ( 'NONE', *, *, #20853, .T. ) ;
#17001=ORIENTED_EDGE ( 'NONE', *, *, #15120, .T. ) ;
#17010=AXIS2_PLACEMENT_3D ( 'NONE', #17047, #30372, #11514 ) ;
#17011=LINE ( 'NONE', #19671, #6771 ) ;
#17014=PLANE ( 'NONE',  #12644 ) ;
#17015=ADVANCED_FACE ( 'NONE', ( #22041 ), #29529, .F. ) ;
#17016=DIRECTION ( 'NONE',  ( -1.000000000000000000, 0.000000000000000000, 0.000000000000000000 ) ) ;
#17017=EDGE_CURVE ( 'NONE', #28736, #5918, #16013, .T. ) ;
#17023=VERTEX_POINT ( 'NONE', #18857 ) ;
#17029=ORIENTED_EDGE ( 'NONE', *, *, #8508, .T. ) ;
#17030=DIRECTION ( 'NONE',  ( -0.9868265225415260300, -0.1617819965527648174, 0.000000000000000000 ) ) ;
#17035=ORIENTED_EDGE ( 'NONE', *, *, #31805, .T. ) ;
#17039=AXIS2_PLACEMENT_3D ( 'NONE', #6494, #17568, #9537 ) ;
#17042=ORIENTED_EDGE ( 'NONE', *, *, #34767, .T. ) ;
#17046=PLANE ( 'NONE',  #7224 ) ;
#17047=CARTESIAN_POINT ( 'NONE',  ( 0.000000000000000000, 2.281310696040539424E-14, -36.68877005347592757 ) ) ;
#17048=CARTESIAN_POINT ( 'NONE',  ( 0.000000000000000000, 2.281310696040539424E-14, -36.68877005347594178 ) ) ;
#17057=ORIENTED_EDGE ( 'NONE', *, *, #323, .T. ) ;
#17062=CARTESIAN_POINT ( 'NONE',  ( -35.00000000000000000, -4.184937238521382774, 68.31122994652405112 ) ) ;
#17063=CARTESIAN_POINT ( 'NONE',  ( 8.927936315454010341, -31.29690601358701940, 68.31122994652405112 ) ) ;
#17068=VERTEX_POINT ( 'NONE', #25226 ) ;
#17076=LINE ( 'NONE', #33957, #8550 ) ;
#17080=ORIENTED_EDGE ( 'NONE', *, *, #3946, .T. ) ;
#17086=ORIENTED_EDGE ( 'NONE', *, *, #2823, .T. ) ;
#17091=CARTESIAN_POINT ( 'NONE',  ( 29.82459402470852083, 33.69708579775584667, -49.43553178847298568 ) ) ;
#17102=DIRECTION ( 'NONE',  ( 0.9941379571543594862, 0.1081190184239433083, -0.000000000000000000 ) ) ;
#17112=EDGE_LOOP ( 'NONE', ( #7678, #11680, #12974, #12467 ) ) ;
#17113=ORIENTED_EDGE ( 'NONE', *, *, #7892, .T. ) ;
#17114=AXIS2_PLACEMENT_3D ( 'NONE', #28087, #22928, #25408 ) ;
#17124=PLANE ( 'NONE',  #2190 ) ;
#17126=ORIENTED_EDGE ( 'NONE', *, *, #31834, .F. ) ;
#17128=LINE ( 'NONE', #3046, #20824 ) ;
#17134=DIRECTION ( 'NONE',  ( 0.5611870653623829419, -0.8276889981568901211, -1.520440023423472285E-16 ) ) ;
#17136=CARTESIAN_POINT ( 'NONE',  ( 22.89764159710611224, 17.63622956525712127, -77.50000000000000000 ) ) ;
#17138=VERTEX_POINT ( 'NONE', #8863 ) ;
#17142=FACE_OUTER_BOUND ( 'NONE', #562, .T. ) ;
#17147=ADVANCED_FACE ( 'NONE', ( #22217 ), #27728, .T. ) ;
#17151=VERTEX_POINT ( 'NONE', #22753 ) ;
#17155=EDGE_CURVE ( 'NONE', #12216, #33289, #25044, .T. ) ;
#17158=VECTOR ( 'NONE', #5160, 1000.000000000000000 ) ;
#17169=DIRECTION ( 'NONE',  ( 0.000000000000000000, 1.836970198721029688E-16, -1.000000000000000000 ) ) ;
#17182=DIRECTION ( 'NONE',  ( -1.000000000000000000, 6.792721752314501023E-48, -3.697785493223492838E-32 ) ) ;
#17183=ORIENTED_EDGE ( 'NONE', *, *, #10963, .T. ) ;
#17185=VECTOR ( 'NONE', #24553, 1000.000000000000000 ) ;
#17187=DIRECTION ( 'NONE',  ( 1.000000000000000000, 0.000000000000000000, -0.000000000000000000 ) ) ;
#17190=ADVANCED_FACE ( 'NONE', ( #3691 ), #11904, .F. ) ;
#17202=LINE ( 'NONE', #32833, #10342 ) ;
#17211=ORIENTED_EDGE ( 'NONE', *, *, #6012, .T. ) ;
#17214=ORIENTED_EDGE ( 'NONE', *, *, #6445, .T. ) ;
#17217=DIRECTION ( 'NONE',  ( 0.000000000000000000, -1.000000000000000000, -2.132064625830773463E-16 ) ) ;
#17220=CARTESIAN_POINT ( 'NONE',  ( -37.71145559917817280, 3.353962854566122864, 15.81122994652406355 ) ) ;
#17224=DIRECTION ( 'NONE',  ( 0.000000000000000000, 1.000000000000000000, 1.934419779023891545E-16 ) ) ;
#17237=STYLED_ITEM('',(#35289),#34166);
#17240=CIRCLE ( 'NONE', #7528, 32.54542015209057126 ) ;
#17256=EDGE_CURVE ( 'NONE', #7553, #18186, #12432, .T. ) ;
#17259=PLANE ( 'NONE',  #17114 ) ;
#17262=ORIENTED_EDGE ( 'NONE', *, *, #2309, .T. ) ;
#17265=DIRECTION ( 'NONE',  ( -0.5155538571770218459, 0.8568571761675891629, -0.000000000000000000 ) ) ;
#17268=ORIENTED_EDGE ( 'NONE', *, *, #26717, .F. ) ;
#17270=LINE ( 'NONE', #4045, #3241 ) ;
#17274=CARTESIAN_POINT ( 'NONE',  ( -37.69926482250235722, 3.578808500140873150, 16.17202516343389007 ) ) ;
#17276=ORIENTED_EDGE ( 'NONE', *, *, #19862, .F. ) ;
#17278=CIRCLE ( 'NONE', #15555, 32.54542015209054284 ) ;
#17280=EDGE_LOOP ( 'NONE', ( #4784, #30450, #885, #11025 ) ) ;
#17281=CARTESIAN_POINT ( 'NONE',  ( -35.00000000000000000, -38.34433698000722046, -36.69637551990492597 ) ) ;
#17296=EDGE_CURVE ( 'NONE', #33041, #12035, #25942, .T. ) ;
#17297=EDGE_CURVE ( 'NONE', #27275, #28991, #12258, .T. ) ;
#17298=CARTESIAN_POINT ( 'NONE',  ( 0.000000000000000000, -33.69708579775584667, 49.43553178847298568 ) ) ;
#17304=CARTESIAN_POINT ( 'NONE',  ( 8.485274312747504766, 31.41981051364775013, 68.31122994652405112 ) ) ;
#17310=ORIENTED_EDGE ( 'NONE', *, *, #9489, .T. ) ;
#17323=CARTESIAN_POINT ( 'NONE',  ( -28.00450684652666311, 16.58167570419054115, 68.31122994652405112 ) ) ;
#17333=VECTOR ( 'NONE', #13061, 1000.000000000000000 ) ;
#17338=VECTOR ( 'NONE', #33506, 1000.000000000000227 ) ;
#17341=ADVANCED_FACE ( 'NONE', ( #4548 ), #1896, .T. ) ;
#17345=ORIENTED_EDGE ( 'NONE', *, *, #9991, .T. ) ;
#17355=DIRECTION ( 'NONE',  ( 0.6051742151937647973, -0.7960930657056438653, -0.000000000000000000 ) ) ;
#17357=EDGE_CURVE ( 'NONE', #2971, #13032, #14754, .T. ) ;
#17361=EDGE_LOOP ( 'NONE', ( #6477, #12897, #6944, #14203 ) ) ;
#17372=PLANE ( 'NONE',  #32575 ) ;
#17385=ORIENTED_EDGE ( 'NONE', *, *, #33137, .F. ) ;
#17391=ORIENTED_EDGE ( 'NONE', *, *, #29825, .T. ) ;
#17398=DIRECTION ( 'NONE',  ( 0.000000000000000000, 0.000000000000000000, 1.000000000000000000 ) ) ;
#17401=ORIENTED_EDGE ( 'NONE', *, *, #28256, .T. ) ;
#17404=CARTESIAN_POINT ( 'NONE',  ( 37.86520737902618805, 0.5181781365365116798, 68.31122994652405112 ) ) ;
#17406=CARTESIAN_POINT ( 'NONE',  ( 29.44023756548695658, 13.87360028845404614, 68.31122994652405112 ) ) ;
#17411=DIRECTION ( 'NONE',  ( 1.000000000000000000, 0.000000000000000000, -0.000000000000000000 ) ) ;
#17412=ORIENTED_EDGE ( 'NONE', *, *, #21002, .F. ) ;
#17423=DIRECTION ( 'NONE',  ( 0.000000000000000000, 1.836970198721029441E-16, -1.000000000000000000 ) ) ;
#17424=VECTOR ( 'NONE', #1453, 1000.000000000000000 ) ;
#17428=LINE ( 'NONE', #8854, #31900 ) ;
#17429=LINE ( 'NONE', #3157, #11681 ) ;
#17456=LINE ( 'NONE', #11498, #26577 ) ;
#17458=ORIENTED_EDGE ( 'NONE', *, *, #17256, .F. ) ;
#17460=DIRECTION ( 'NONE',  ( -0.000000000000000000, 1.000000000000000000, -0.000000000000000000 ) ) ;
#17465=CARTESIAN_POINT ( 'NONE',  ( -5.021133111224679091, 28.08988295778447508, -87.50000000000000000 ) ) ;
#17471=CARTESIAN_POINT ( 'NONE',  ( 0.000000000000000000, 3.524919873834583163E-15, 68.31122994652405112 ) ) ;
#17473=AXIS2_PLACEMENT_3D ( 'NONE', #9160, #12205, #6480 ) ;
#17474=ADVANCED_FACE ( 'NONE', ( #10443 ), #4908, .F. ) ;
#17477=ORIENTED_EDGE ( 'NONE', *, *, #13187, .T. ) ;
#17489=LINE ( 'NONE', #14634, #16983 ) ;
#17492=CARTESIAN_POINT ( 'NONE',  ( -35.00000000000000000, 42.49491490430484220, -36.69637551990492597 ) ) ;
#17496=EDGE_LOOP ( 'NONE', ( #12712, #20174, #27967, #22459, #23657, #25320 ) ) ;
#17501=DIRECTION ( 'NONE',  ( 0.000000000000000000, -1.000000000000000000, -1.836970198721029688E-16 ) ) ;
#17503=CARTESIAN_POINT ( 'NONE',  ( 29.63313772848249883, -13.45665341906702395, 49.43553178847298568 ) ) ;
#17507=AXIS2_PLACEMENT_3D ( 'NONE', #24849, #484, #18831 ) ;
#17509=EDGE_CURVE ( 'NONE', #1134, #22879, #27508, .T. ) ;
#17511=CARTESIAN_POINT ( 'NONE',  ( 8.927936315454026328, -31.29690601358698387, -36.68877005347593467 ) ) ;
#17515=CIRCLE ( 'NONE', #29981, 44.99999999999998579 ) ;
#17523=ORIENTED_EDGE ( 'NONE', *, *, #24560, .F. ) ;
#17524=CARTESIAN_POINT ( 'NONE',  ( -34.66645501699844090, -15.21971901163155216, 68.31122994652405112 ) ) ;
#17531=VERTEX_POINT ( 'NONE', #11502 ) ;
#17532=CARTESIAN_POINT ( 'NONE',  ( 8.485274312747499437, 31.41981051364775013, 68.31122994652405112 ) ) ;
#17540=LINE ( 'NONE', #28375, #30696 ) ;
#17547=CARTESIAN_POINT ( 'NONE',  ( 30.98406361983695234, 9.959526819984926505, 68.31122994652405112 ) ) ;
#17549=EDGE_CURVE ( 'NONE', #7713, #23102, #1940, .T. ) ;
#17550=AXIS2_PLACEMENT_3D ( 'NONE', #7144, #24045, #7497 ) ;
#17553=EDGE_CURVE ( 'NONE', #31542, #16320, #16503, .T. ) ;
#17556=LINE ( 'NONE', #6296, #24822 ) ;
#17557=ORIENTED_EDGE ( 'NONE', *, *, #1104, .T. ) ;
#17559=DIRECTION ( 'NONE',  ( 1.000000000000000000, 0.000000000000000000, 0.000000000000000000 ) ) ;
#17561=VECTOR ( 'NONE', #19924, 1000.000000000000227 ) ;
#17563=PLANE ( 'NONE',  #2011 ) ;
#17568=DIRECTION ( 'NONE',  ( 0.000000000000000000, 0.000000000000000000, 1.000000000000000000 ) ) ;
#17569=CIRCLE ( 'NONE', #14174, 2.085824230283342740 ) ;
#17573=ORIENTED_EDGE ( 'NONE', *, *, #15750, .T. ) ;
#17578=DIRECTION ( 'NONE',  ( 0.000000000000000000, -1.000000000000000000, -1.541976423090495633E-16 ) ) ;
#17593=EDGE_CURVE ( 'NONE', #24798, #17629, #8642, .T. ) ;
#17595=VERTEX_POINT ( 'NONE', #3126 ) ;
#17596=EDGE_CURVE ( 'NONE', #2751, #29867, #27859, .T. ) ;
#17601=EDGE_CURVE ( 'NONE', #12010, #22497, #14180, .T. ) ;
#17605=CARTESIAN_POINT ( 'NONE',  ( -37.58721499952019940, -4.609089608337744615, 15.81122994652406355 ) ) ;
#17606=VERTEX_POINT ( 'NONE', #8819 ) ;
#17607=DIRECTION ( 'NONE',  ( 1.097052971696008773E-16, -0.8958117331950891105, -0.4444337280967887160 ) ) ;
#17615=VERTEX_POINT ( 'NONE', #22536 ) ;
#17616=CARTESIAN_POINT ( 'NONE',  ( 5.021133111224265200, -11.61907005722761177, -87.50000000000000000 ) ) ;
#17618=CARTESIAN_POINT ( 'NONE',  ( -37.85301660235036536, 0.7430237821112573027, 68.31122994652405112 ) ) ;
#17627=CARTESIAN_POINT ( 'NONE',  ( 5.021133111224576062, 18.16264470403145026, -67.50000000000000000 ) ) ;
#17628=CARTESIAN_POINT ( 'NONE',  ( 14.14940496480368815, 33.69708579775584667, 49.43553178847298568 ) ) ;
#17629=VERTEX_POINT ( 'NONE', #11328 ) ;
#17631=CARTESIAN_POINT ( 'NONE',  ( -5.491809612354312087, 32.07872192057773475, 68.31122994652405112 ) ) ;
#17633=CARTESIAN_POINT ( 'NONE',  ( 12.46788440507149787, 30.06253867087536946, 49.43553178847298568 ) ) ;
#17637=CARTESIAN_POINT ( 'NONE',  ( -20.02113311122498729, -1.691831803474591833, -67.50000000000000000 ) ) ;
#17639=DIRECTION ( 'NONE',  ( 0.000000000000000000, 1.836970198721029441E-16, -1.000000000000000000 ) ) ;
#17644=ADVANCED_FACE ( 'NONE', ( #13998 ), #24837, .T. ) ;
#17649=CARTESIAN_POINT ( 'NONE',  ( -5.614556921127968003, -37.45022281665699637, 68.31122994652405112 ) ) ;
#17654=EDGE_CURVE ( 'NONE', #20922, #18325, #12218, .T. ) ;
#17657=VERTEX_POINT ( 'NONE', #28399 ) ;
#17659=CARTESIAN_POINT ( 'NONE',  ( -18.07349068442144358, -27.06572199953721736, 68.31122994652405112 ) ) ;
#17661=FACE_OUTER_BOUND ( 'NONE', #633, .T. ) ;
#17663=ORIENTED_EDGE ( 'NONE', *, *, #15735, .F. ) ;
#17666=ORIENTED_EDGE ( 'NONE', *, *, #593, .T. ) ;
#17667=DIRECTION ( 'NONE',  ( 0.000000000000000000, 0.000000000000000000, 1.000000000000000000 ) ) ;
#17669=DIRECTION ( 'NONE',  ( -0.000000000000000000, 1.836970198721029688E-16, -1.000000000000000000 ) ) ;
#17675=VERTEX_POINT ( 'NONE', #6838 ) ;
#17676=DIRECTION ( 'NONE',  ( 0.6051742151937647973, -0.7960930657056438653, -0.000000000000000000 ) ) ;
#17677=AXIS2_PLACEMENT_3D ( 'NONE', #26121, #1737, #28968 ) ;
#17681=ORIENTED_EDGE ( 'NONE', *, *, #13222, .F. ) ;
#17685=ORIENTED_EDGE ( 'NONE', *, *, #2321, .F. ) ;
#17687=EDGE_LOOP ( 'NONE', ( #26020, #22668, #20866, #24926 ) ) ;
#17698=CARTESIAN_POINT ( 'NONE',  ( -20.72055270933793736, 25.09707290294328885, 68.31122994652405112 ) ) ;
#17702=VERTEX_POINT ( 'NONE', #20223 ) ;
#17705=CARTESIAN_POINT ( 'NONE',  ( -37.85301660235036536, 0.7430237821112727348, -15.81122994652406355 ) ) ;
#17713=DIRECTION ( 'NONE',  ( 0.000000000000000000, 1.000000000000000000, 0.000000000000000000 ) ) ;
#17722=AXIS2_PLACEMENT_3D ( 'NONE', #19101, #16256, #21225 ) ;
#17724=VERTEX_POINT ( 'NONE', #20736 ) ;
#17729=ORIENTED_EDGE ( 'NONE', *, *, #8772, .T. ) ;
#17738=ORIENTED_EDGE ( 'NONE', *, *, #3369, .F. ) ;
#17739=ORIENTED_EDGE ( 'NONE', *, *, #6523, .T. ) ;
#17745=CARTESIAN_POINT ( 'NONE',  ( -29.68486519896224962, 23.49918569563713078, -36.68877005347593467 ) ) ;
#17757=VERTEX_POINT ( 'NONE', #15231 ) ;
#17774=CARTESIAN_POINT ( 'NONE',  ( 20.62763069236413926, -31.74750072459299588, 68.31122994652405112 ) ) ;
#17788=VECTOR ( 'NONE', #34322, 1000.000000000000000 ) ;
#17790=AXIS2_PLACEMENT_3D ( 'NONE', #26751, #16091, #18766 ) ;
#17791=CARTESIAN_POINT ( 'NONE',  ( -1.307386931792819285, 37.83772838912472025, -36.68877005347593467 ) ) ;
#17793=LINE ( 'NONE', #28626, #23807 ) ;
#17798=ORIENTED_EDGE ( 'NONE', *, *, #5037, .F. ) ;
#17816=DIRECTION ( 'NONE',  ( -0.8276889981568904542, 0.5611870653623824978, -0.000000000000000000 ) ) ;
#17832=CARTESIAN_POINT ( 'NONE',  ( 3.235562306570555532E-30, -5.758675521474011738, -87.50000000000000000 ) ) ;
#17833=VERTEX_POINT ( 'NONE', #5212 ) ;
#17852=ORIENTED_EDGE ( 'NONE', *, *, #17596, .F. ) ;
#17856=ORIENTED_EDGE ( 'NONE', *, *, #23181, .T. ) ;
#17863=ORIENTED_EDGE ( 'NONE', *, *, #13615, .F. ) ;
#17866=CARTESIAN_POINT ( 'NONE',  ( 14.14940496480368992, 33.69708579775584667, 68.31122994652405112 ) ) ;
#17867=DIRECTION ( 'NONE',  ( 1.000000000000000000, 0.000000000000000000, 0.000000000000000000 ) ) ;
#17870=EDGE_CURVE ( 'NONE', #18461, #29867, #18460, .T. ) ;
#17875=CARTESIAN_POINT ( 'NONE',  ( 3.235562306570555532E-30, -5.758675521474015291, -67.50000000000000000 ) ) ;
#17877=CARTESIAN_POINT ( 'NONE',  ( 5.713835024271039842, 32.03991982186467880, -36.68877005347593467 ) ) ;
#17886=AXIS2_PLACEMENT_3D ( 'NONE', #10846, #21873, #167 ) ;
#17887=DIRECTION ( 'NONE',  ( -0.000000000000000000, 1.836970198721029934E-16, -1.000000000000000000 ) ) ;
#17898=FACE_OUTER_BOUND ( 'NONE', #33671, .T. ) ;
#17903=ORIENTED_EDGE ( 'NONE', *, *, #32337, .F. ) ;
#17905=EDGE_CURVE ( 'NONE', #20006, #16672, #26412, .T. ) ;
#17910=ORIENTED_EDGE ( 'NONE', *, *, #18951, .F. ) ;
#17933=DIRECTION ( 'NONE',  ( 0.6876994588534234287, 0.7259954919231307313, 1.333632083068605180E-16 ) ) ;
#17935=CARTESIAN_POINT ( 'NONE',  ( 34.14795412574902400, 16.36947364650383818, 68.31122994652405112 ) ) ;
#17936=ORIENTED_EDGE ( 'NONE', *, *, #10693, .T. ) ;
#17942=VECTOR ( 'NONE', #13094, 1000.000000000000000 ) ;
#17944=EDGE_CURVE ( 'NONE', #27831, #20735, #27469, .T. ) ;
#17945=CIRCLE ( 'NONE', #511, 32.54542015209054284 ) ;
#17949=VERTEX_POINT ( 'NONE', #11640 ) ;
#17951=DIRECTION ( 'NONE',  ( 0.000000000000000000, -1.000000000000000000, -3.083952846180992253E-16 ) ) ;
#17954=ORIENTED_EDGE ( 'NONE', *, *, #19153, .F. ) ;
#17958=ORIENTED_EDGE ( 'NONE', *, *, #14621, .T. ) ;
#17967=EDGE_LOOP ( 'NONE', ( #31309, #12681, #27639, #32244 ) ) ;
#17969=DIRECTION ( 'NONE',  ( -0.000000000000000000, -1.836970198721029688E-16, 1.000000000000000000 ) ) ;
#17970=VECTOR ( 'NONE', #29982, 1000.000000000000000 ) ;
#17974=CARTESIAN_POINT ( 'NONE',  ( 20.89386240318430055, 24.95297350523386015, 49.43553178847298568 ) ) ;
#17981=VERTEX_POINT ( 'NONE', #6093 ) ;
#17982=CARTESIAN_POINT ( 'NONE',  ( 0.000000000000000000, 10.87635688602997597, 87.50000000000000000 ) ) ;
#17985=VECTOR ( 'NONE', #2905, 1000.000000000000114 ) ;
#17992=EDGE_LOOP ( 'NONE', ( #5159, #28757, #34361, #9552 ) ) ;
#17999=CARTESIAN_POINT ( 'NONE',  ( 0.000000000000000000, 2.281310696040539424E-14, -36.68877005347594178 ) ) ;
#18002=DIRECTION ( 'NONE',  ( -0.000000000000000000, -1.836970198721029688E-16, 1.000000000000000000 ) ) ;
#18007=LINE ( 'NONE', #2130, #29516 ) ;
#18012=VECTOR ( 'NONE', #4885, 1000.000000000000000 ) ;
#18014=DIRECTION ( 'NONE',  ( 0.000000000000000000, 1.836970198721029934E-16, -1.000000000000000000 ) ) ;
#18021=CARTESIAN_POINT ( 'NONE',  ( -29.72561944762171393, -13.25111019240559251, 68.31122994652405112 ) ) ;
#18025=FACE_OUTER_BOUND ( 'NONE', #31954, .T. ) ;
#18031=EDGE_CURVE ( 'NONE', #6803, #28782, #592, .T. ) ;
#18035=EDGE_CURVE ( 'NONE', #9940, #24880, #22134, .T. ) ;
#18050=ORIENTED_EDGE ( 'NONE', *, *, #9076, .F. ) ;
#18052=FACE_OUTER_BOUND ( 'NONE', #12731, .T. ) ;
#18053=AXIS2_PLACEMENT_3D ( 'NONE', #4887, #31942, #7556 ) ;
#18055=CARTESIAN_POINT ( 'NONE',  ( 8.485274312747499437, 31.41981051364776789, -36.68877005347593467 ) ) ;
#18056=LINE ( 'NONE', #4649, #23939 ) ;
#18060=VECTOR ( 'NONE', #13368, 1000.000000000000000 ) ;
#18064=DIRECTION ( 'NONE',  ( 0.000000000000000000, 0.000000000000000000, 1.000000000000000000 ) ) ;
#18076=ORIENTED_EDGE ( 'NONE', *, *, #24364, .T. ) ;
#18083=AXIS2_PLACEMENT_3D ( 'NONE', #23852, #34718, #15876 ) ;
#18087=ORIENTED_EDGE ( 'NONE', *, *, #7254, .T. ) ;
#18088=ORIENTED_EDGE ( 'NONE', *, *, #3992, .F. ) ;
#18089=DIRECTION ( 'NONE',  ( 3.697785493223492838E-32, 1.934419779023891545E-16, -1.000000000000000000 ) ) ;
#18090=ADVANCED_FACE ( 'NONE', ( #14312 ), #65, .F. ) ;
#18094=ORIENTED_EDGE ( 'NONE', *, *, #3992, .T. ) ;
#18098=DIRECTION ( 'NONE',  ( 0.000000000000000000, 0.000000000000000000, 1.000000000000000000 ) ) ;
#18101=DIRECTION ( 'NONE',  ( 0.000000000000000000, 1.836970198721029688E-16, -1.000000000000000000 ) ) ;
#18111=CARTESIAN_POINT ( 'NONE',  ( 0.000000000000000000, 3.524919873834583163E-15, 68.31122994652405112 ) ) ;
#18113=ORIENTED_EDGE ( 'NONE', *, *, #18677, .T. ) ;
#18116=DIRECTION ( 'NONE',  ( 0.000000000000000000, 1.836970198721029441E-16, -1.000000000000000000 ) ) ;
#18117=ORIENTED_EDGE ( 'NONE', *, *, #14604, .T. ) ;
#18121=AXIS2_PLACEMENT_3D ( 'NONE', #26905, #7682, #34750 ) ;
#18142=LINE ( 'NONE', #4221, #27129 ) ;
#18148=LINE ( 'NONE', #32165, #14337 ) ;
#18160=CARTESIAN_POINT ( 'NONE',  ( -8.267476927982267298, 31.47782073335735831, 68.31122994652405112 ) ) ;
#18164=ORIENTED_EDGE ( 'NONE', *, *, #2568, .T. ) ;
#18170=VECTOR ( 'NONE', #24617, 1000.000000000000000 ) ;
#18174=LINE ( 'NONE', #9621, #18689 ) ;
#18175=EDGE_CURVE ( 'NONE', #20191, #13441, #31364, .T. ) ;
#18184=DIRECTION ( 'NONE',  ( -0.000000000000000000, 1.836970198721029688E-16, -1.000000000000000000 ) ) ;
#18186=VERTEX_POINT ( 'NONE', #17524 ) ;
#18193=CARTESIAN_POINT ( 'NONE',  ( 3.235562306570555532E-30, -15.68591377522703745, -67.50000000000000000 ) ) ;
#18195=CIRCLE ( 'NONE', #21019, 32.54542015209057126 ) ;
#18206=ADVANCED_FACE ( 'NONE', ( #952 ), #19999, .F. ) ;
#18207=VERTEX_POINT ( 'NONE', #33684 ) ;
#18217=LINE ( 'NONE', #16071, #383 ) ;
#18225=CARTESIAN_POINT ( 'NONE',  ( -35.00000000000000000, -4.831299144296466785, -15.81122994652406355 ) ) ;
#18228=CARTESIAN_POINT ( 'NONE',  ( 5.713835024271038954, 32.03991982186465748, 49.43553178847298568 ) ) ;
#18231=VECTOR ( 'NONE', #33016, 1000.000000000000000 ) ;
#18243=ORIENTED_EDGE ( 'NONE', *, *, #23285, .F. ) ;
#18244=ORIENTED_EDGE ( 'NONE', *, *, #29347, .T. ) ;
#18249=DIRECTION ( 'NONE',  ( 0.000000000000000000, 1.000000000000000000, 0.000000000000000000 ) ) ;
#18250=CONICAL_SURFACE ( 'NONE', #33553, 32.54542015209054995, 1.389864428407444175 ) ;
#18253=EDGE_LOOP ( 'NONE', ( #20773, #10608, #12473, #13948 ) ) ;
#18256=LINE ( 'NONE', #34089, #3297 ) ;
#18257=EDGE_CURVE ( 'NONE', #18794, #5262, #34564, .T. ) ;
#18258=CARTESIAN_POINT ( 'NONE',  ( 60.00000000000000000, -33.69708579775584667, -49.43553178847298568 ) ) ;
#18264=EDGE_CURVE ( 'NONE', #2764, #30924, #5000, .T. ) ;
#18269=LINE ( 'NONE', #18964, #16303 ) ;
#18277=AXIS2_PLACEMENT_3D ( 'NONE', #32773, #27087, #32594 ) ;
#18279=DIRECTION ( 'NONE',  ( -0.000000000000000000, -1.836970198721029688E-16, 1.000000000000000000 ) ) ;
#18283=EDGE_LOOP ( 'NONE', ( #29994, #20093, #6378, #2658 ) ) ;
#18286=CARTESIAN_POINT ( 'NONE',  ( -34.04247984038124031, 16.56841925338180488, 68.31122994652405112 ) ) ;
#18288=EDGE_LOOP ( 'NONE', ( #2976, #9529, #19653, #30309 ) ) ;
#18290=EDGE_CURVE ( 'NONE', #11221, #15121, #2334, .T. ) ;
#18293=AXIS2_PLACEMENT_3D ( 'NONE', #31856, #10336, #21196 ) ;
#18299=ADVANCED_FACE ( 'NONE', ( #15714 ), #31873, .F. ) ;
#18302=CARTESIAN_POINT ( 'NONE',  ( -20.02113311122488781, 4.168562732279007754, -87.50000000000000000 ) ) ;
#18305=ORIENTED_EDGE ( 'NONE', *, *, #20872, .F. ) ;
#18310=DIRECTION ( 'NONE',  ( 0.000000000000000000, 1.000000000000000000, 0.000000000000000000 ) ) ;
#18311=ADVANCED_FACE ( 'NONE', ( #33772 ), #28867, .F. ) ;
#18313=CARTESIAN_POINT ( 'NONE',  ( 3.235562306570555532E-30, -15.68591377522703745, -67.50000000000000000 ) ) ;
#18315=VERTEX_POINT ( 'NONE', #34741 ) ;
#18325=VERTEX_POINT ( 'NONE', #26722 ) ;
#18326=VECTOR ( 'NONE', #32558, 1000.000000000000000 ) ;
#18331=CARTESIAN_POINT ( 'NONE',  ( -18.07349068442141515, -27.06572199953722446, 68.31122994652405112 ) ) ;
#18332=DIRECTION ( 'NONE',  ( -0.8835120444460228262, 0.4684084406997903183, 0.000000000000000000 ) ) ;
#18347=LINE ( 'NONE', #13000, #15283 ) ;
#18351=ORIENTED_EDGE ( 'NONE', *, *, #18466, .F. ) ;
#18352=CARTESIAN_POINT ( 'NONE',  ( -36.04853892210774546, 11.59936550071286909, 29.04209251724894614 ) ) ;
#18359=ADVANCED_FACE ( 'NONE', ( #15360 ), #26190, .T. ) ;
#18360=DIRECTION ( 'NONE',  ( 0.000000000000000000, 0.000000000000000000, 1.000000000000000000 ) ) ;
#18365=CARTESIAN_POINT ( 'NONE',  ( 5.021133111224576062, 16.12922284503173742, -67.50000000000000000 ) ) ;
#18380=AXIS2_PLACEMENT_3D ( 'NONE', #31560, #29424, #12529 ) ;
#18384=DIRECTION ( 'NONE',  ( 0.000000000000000000, 1.836970198721029441E-16, -1.000000000000000000 ) ) ;
#18399=FACE_OUTER_BOUND ( 'NONE', #32064, .T. ) ;
#18400=PLANE ( 'NONE',  #9439 ) ;
#18407=EDGE_CURVE ( 'NONE', #13218, #29274, #16242, .T. ) ;
#18409=ORIENTED_EDGE ( 'NONE', *, *, #19013, .F. ) ;
#18413=EDGE_CURVE ( 'NONE', #16274, #12217, #18515, .T. ) ;
#18415=EDGE_CURVE ( 'NONE', #10097, #7307, #11410, .T. ) ;
#18426=VERTEX_POINT ( 'NONE', #27248 ) ;
#18432=VERTEX_POINT ( 'NONE', #200 ) ;
#18433=ORIENTED_EDGE ( 'NONE', *, *, #9965, .T. ) ;
#18436=PLANE ( 'NONE',  #31694 ) ;
#18441=CARTESIAN_POINT ( 'NONE',  ( 22.89764159710613001, 8.346743312457579833, -77.50000000000000000 ) ) ;
#18448=LINE ( 'NONE', #29288, #18012 ) ;
#18460=CIRCLE ( 'NONE', #11083, 2.033421858999711951 ) ;
#18461=VERTEX_POINT ( 'NONE', #3036 ) ;
#18463=FACE_OUTER_BOUND ( 'NONE', #18975, .T. ) ;
#18466=EDGE_CURVE ( 'NONE', #15452, #19731, #8027, .T. ) ;
#18475=VERTEX_POINT ( 'NONE', #30271 ) ;
#18479=VECTOR ( 'NONE', #11197, 1000.000000000000000 ) ;
#18485=ORIENTED_EDGE ( 'NONE', *, *, #4792, .T. ) ;
#18486=VERTEX_POINT ( 'NONE', #11598 ) ;
#18509=PLANE ( 'NONE',  #29782 ) ;
#18511=DIRECTION ( 'NONE',  ( 1.000000000000000000, 0.000000000000000000, -0.000000000000000000 ) ) ;
#18513=DIRECTION ( 'NONE',  ( -1.000000000000000000, 0.000000000000000000, 0.000000000000000000 ) ) ;
#18514=ORIENTED_EDGE ( 'NONE', *, *, #4792, .F. ) ;
#18515=CIRCLE ( 'NONE', #22464, 32.54542015209055705 ) ;
#18518=ADVANCED_FACE ( 'NONE', ( #3745 ), #20475, .F. ) ;
#18531=DIRECTION ( 'NONE',  ( 1.000000000000000000, 0.000000000000000000, 0.000000000000000000 ) ) ;
#18533=ORIENTED_EDGE ( 'NONE', *, *, #22869, .T. ) ;
#18534=ORIENTED_EDGE ( 'NONE', *, *, #15750, .F. ) ;
#18535=LINE ( 'NONE', #26692, #11206 ) ;
#18536=VERTEX_POINT ( 'NONE', #17649 ) ;
#18545=DIRECTION ( 'NONE',  ( 1.000000000000000000, 0.000000000000000000, 0.000000000000000000 ) ) ;
#18547=CIRCLE ( 'NONE', #34426, 44.99999999999997158 ) ;
#18549=ADVANCED_FACE ( 'NONE', ( #11952 ), #14973, .F. ) ;
#18551=CARTESIAN_POINT ( 'NONE',  ( 10.17231796313409298, 8.346743312457579833, -77.50000000000000000 ) ) ;
#18553=EDGE_CURVE ( 'NONE', #13770, #14420, #23156, .T. ) ;
#18558=VECTOR ( 'NONE', #12763, 1000.000000000000227 ) ;
#18565=ORIENTED_EDGE ( 'NONE', *, *, #26666, .T. ) ;
#18566=VERTEX_POINT ( 'NONE', #4260 ) ;
#18571=PLANE ( 'NONE',  #17550 ) ;
#18576=CARTESIAN_POINT ( 'NONE',  ( -41.91706493227329133, 16.36947364650383818, -36.69637551990492597 ) ) ;
#18578=CARTESIAN_POINT ( 'NONE',  ( 0.000000000000000000, 3.524919873834583163E-15, 68.31122994652405112 ) ) ;
#18584=DIRECTION ( 'NONE',  ( -0.8854131517428557308, 0.2458337514780905841, 0.3944734685057932899 ) ) ;
#18586=CARTESIAN_POINT ( 'NONE',  ( 31.73435513276361775, 7.220462394039765641, 49.43553178847298568 ) ) ;
#18588=CARTESIAN_POINT ( 'NONE',  ( -12.25939112814508825, 30.14816249862101927, 68.31122994652405112 ) ) ;
#18595=ORIENTED_EDGE ( 'NONE', *, *, #12244, .F. ) ;
#18597=VERTEX_POINT ( 'NONE', #1431 ) ;
#18599=FACE_BOUND ( 'NONE', #23922, .T. ) ;
#18612=FACE_OUTER_BOUND ( 'NONE', #13614, .T. ) ;
#18613=EDGE_CURVE ( 'NONE', #21072, #26369, #28172, .T. ) ;
#18615=DIRECTION ( 'NONE',  ( 0.000000000000000000, 1.000000000000000000, 0.000000000000000000 ) ) ;
#18633=DIRECTION ( 'NONE',  ( 0.3193015301359802827, 0.9476531711828023452, 1.740810634186286145E-16 ) ) ;
#18637=VERTEX_POINT ( 'NONE', #27953 ) ;
#18638=PLANE ( 'NONE',  #20044 ) ;
#18647=CARTESIAN_POINT ( 'NONE',  ( -9.978866888775527855, 4.168562732279004202, -67.50000000000000000 ) ) ;
#18651=VERTEX_POINT ( 'NONE', #12129 ) ;
#18653=ORIENTED_EDGE ( 'NONE', *, *, #20098, .F. ) ;
#18662=LINE ( 'NONE', #18313, #9527 ) ;
#18675=ORIENTED_EDGE ( 'NONE', *, *, #34982, .F. ) ;
#18677=EDGE_CURVE ( 'NONE', #4598, #20852, #34165, .T. ) ;
#18682=CARTESIAN_POINT ( 'NONE',  ( 29.63313772848250238, -13.45665341906703816, 68.31122994652405112 ) ) ;
#18683=FACE_OUTER_BOUND ( 'NONE', #3655, .T. ) ;
#18689=VECTOR ( 'NONE', #26507, 1000.000000000000114 ) ;
#18691=VERTEX_POINT ( 'NONE', #10975 ) ;
#18699=DIRECTION ( 'NONE',  ( -0.000000000000000000, 0.5288966977476834419, -0.8486862100397269959 ) ) ;
#18704=CARTESIAN_POINT ( 'NONE',  ( 0.000000000000000000, 2.281310696040539424E-14, -36.68877005347592757 ) ) ;
#18706=CARTESIAN_POINT ( 'NONE',  ( -35.00000000000000000, 16.36947364650383818, 36.69637551990492597 ) ) ;
#18727=FACE_OUTER_BOUND ( 'NONE', #7209, .T. ) ;
#18732=EDGE_CURVE ( 'NONE', #8317, #1101, #30019, .T. ) ;
#18733=VECTOR ( 'NONE', #23956, 1000.000000000000114 ) ;
#18743=DIRECTION ( 'NONE',  ( 1.000000000000000000, 0.000000000000000000, -0.000000000000000000 ) ) ;
#18744=ORIENTED_EDGE ( 'NONE', *, *, #3073, .F. ) ;
#18748=DIRECTION ( 'NONE',  ( 0.000000000000000000, 1.836970198721029441E-16, -1.000000000000000000 ) ) ;
#18753=CARTESIAN_POINT ( 'NONE',  ( -14.84098889165989377, 28.96462362251111244, 68.31122994652405112 ) ) ;
#18761=DIRECTION ( 'NONE',  ( 0.000000000000000000, 0.000000000000000000, 1.000000000000000000 ) ) ;
#18762=DIRECTION ( 'NONE',  ( 1.000000000000000000, 0.000000000000000000, 0.000000000000000000 ) ) ;
#18766=DIRECTION ( 'NONE',  ( -1.000000000000000000, 0.000000000000000000, -0.000000000000000000 ) ) ;
#18774=FACE_OUTER_BOUND ( 'NONE', #29548, .T. ) ;
#18775=ORIENTED_EDGE ( 'NONE', *, *, #34127, .T. ) ;
#18789=CARTESIAN_POINT ( 'NONE',  ( 5.021133111224679091, 24.02303923978504940, -67.50000000000000000 ) ) ;
#18794=VERTEX_POINT ( 'NONE', #23962 ) ;
#18799=EDGE_CURVE ( 'NONE', #19057, #4259, #34844, .T. ) ;
#18805=AXIS2_PLACEMENT_3D ( 'NONE', #31803, #15288, #15985 ) ;
#18809=EDGE_CURVE ( 'NONE', #22576, #4259, #28048, .T. ) ;
#18812=VERTEX_POINT ( 'NONE', #14005 ) ;
#18822=ORIENTED_EDGE ( 'NONE', *, *, #31224, .T. ) ;
#18826=AXIS2_PLACEMENT_3D ( 'NONE', #20588, #7039, #23604 ) ;
#18831=DIRECTION ( 'NONE',  ( 0.000000000000000000, 0.000000000000000000, 1.000000000000000000 ) ) ;
#18852=EDGE_CURVE ( 'NONE', #29579, #16627, #6501, .T. ) ;
#18853=ORIENTED_EDGE ( 'NONE', *, *, #22212, .T. ) ;
#18854=EDGE_CURVE ( 'NONE', #23681, #14870, #11697, .T. ) ;
#18857=CARTESIAN_POINT ( 'NONE',  ( -9.978866888775733912, -15.68591377522703745, -67.50000000000000000 ) ) ;
#18869=CARTESIAN_POINT ( 'NONE',  ( 8.485274312747504766, 31.41981051364775013, 68.31122994652405112 ) ) ;
#18874=CIRCLE ( 'NONE', #9207, 44.99999999999997158 ) ;
#18877=CARTESIAN_POINT ( 'NONE',  ( 0.000000000000000000, 3.524919873834583163E-15, 68.31122994652405112 ) ) ;
#18878=CARTESIAN_POINT ( 'NONE',  ( 0.000000000000000000, 33.69708579775584667, -36.68877005347592757 ) ) ;
#18879=VERTEX_POINT ( 'NONE', #17404 ) ;
#18888=DIRECTION ( 'NONE',  ( 0.000000000000000000, 1.836970198721029441E-16, -1.000000000000000000 ) ) ;
#18893=ORIENTED_EDGE ( 'NONE', *, *, #26666, .F. ) ;
#18894=VECTOR ( 'NONE', #5754, 1000.000000000000000 ) ;
#18895=CARTESIAN_POINT ( 'NONE',  ( 5.390701026406702567, -37.47456861236020131, 68.31122994652405112 ) ) ;
#18897=VECTOR ( 'NONE', #34860, 1000.000000000000000 ) ;
#18899=ORIENTED_EDGE ( 'NONE', *, *, #5283, .T. ) ;
#18901=EDGE_CURVE ( 'NONE', #1194, #18566, #14546, .T. ) ;
#18906=EDGE_LOOP ( 'NONE', ( #32679, #29743, #23671, #8750, #3578, #3326 ) ) ;
#18907=DIRECTION ( 'NONE',  ( 0.9635499925192230197, -0.2675283385292204774, -0.000000000000000000 ) ) ;
#18918=ORIENTED_EDGE ( 'NONE', *, *, #28306, .T. ) ;
#18919=CARTESIAN_POINT ( 'NONE',  ( 22.89764159710611224, 13.56412600238610544, -87.50000000000000000 ) ) ;
#18924=VECTOR ( 'NONE', #3840, 1000.000000000000000 ) ;
#18927=DIRECTION ( 'NONE',  ( -0.000000000000000000, 1.836970198721029934E-16, -1.000000000000000000 ) ) ;
#18928=DIRECTION ( 'NONE',  ( 0.8568571761675894960, 0.5155538571770215128, -0.000000000000000000 ) ) ;
#18933=ORIENTED_EDGE ( 'NONE', *, *, #9826, .T. ) ;
#18934=FACE_OUTER_BOUND ( 'NONE', #33428, .T. ) ;
#18940=( GEOMETRIC_REPRESENTATION_CONTEXT ( 3 ) GLOBAL_UNCERTAINTY_ASSIGNED_CONTEXT ( ( #1418 ) ) GLOBAL_UNIT_ASSIGNED_CONTEXT ( ( #3776, #9816, #9994 ) ) REPRESENTATION_CONTEXT ( 'NONE', 'WORKASPACE' ) );
#18949=ORIENTED_EDGE ( 'NONE', *, *, #22982, .T. ) ;
#18951=EDGE_CURVE ( 'NONE', #29194, #2425, #1528, .T. ) ;
#18954=EDGE_LOOP ( 'NONE', ( #27284, #14043, #34998, #8566 ) ) ;
#18959=CARTESIAN_POINT ( 'NONE',  ( -25.63124651156763889, 20.05601094782694105, 68.31122994652405112 ) ) ;
#18960=ORIENTED_EDGE ( 'NONE', *, *, #2321, .T. ) ;
#18964=CARTESIAN_POINT ( 'NONE',  ( -35.00000000000000000, -46.95407462254104303, -36.69637551990492597 ) ) ;
#18965=CARTESIAN_POINT ( 'NONE',  ( 10.17231796313411429, 17.63622956525712127, -77.50000000000000000 ) ) ;
#18970=EDGE_LOOP ( 'NONE', ( #17666, #585, #15557, #8488 ) ) ;
#18972=AXIS2_PLACEMENT_3D ( 'NONE', #26791, #26093, #1711 ) ;
#18974=DIRECTION ( 'NONE',  ( -0.6051742151937647973, -0.7960930657056438653, 0.000000000000000000 ) ) ;
#18975=EDGE_LOOP ( 'NONE', ( #19189, #8113, #5218, #26000 ) ) ;
#18985=VERTEX_POINT ( 'NONE', #3998 ) ;
#18988=DIRECTION ( 'NONE',  ( -0.000000000000000000, -1.000000000000000000, -0.000000000000000000 ) ) ;
#18999=VERTEX_POINT ( 'NONE', #20911 ) ;
#19003=DIRECTION ( 'NONE',  ( 0.3193015301359796165, -0.9476531711828025673, 0.000000000000000000 ) ) ;
#19007=LINE ( 'NONE', #34849, #30413 ) ;
#19008=CARTESIAN_POINT ( 'NONE',  ( -39.79673454871243621, -35.10674429148210862, 45.90417104242168733 ) ) ;
#19011=CARTESIAN_POINT ( 'NONE',  ( -25.63124651156763179, 20.05601094782693394, 68.31122994652405112 ) ) ;
#19013=EDGE_CURVE ( 'NONE', #18879, #32399, #3828, .T. ) ;
#19025=DIRECTION ( 'NONE',  ( 0.000000000000000000, 1.000000000000000000, 1.836970198721029688E-16 ) ) ;
#19027=VECTOR ( 'NONE', #3973, 1000.000000000000000 ) ;
#19029=VECTOR ( 'NONE', #34242, 1000.000000000000000 ) ;
#19042=DIRECTION ( 'NONE',  ( 1.000000000000000000, 0.000000000000000000, 0.000000000000000000 ) ) ;
#19045=ORIENTED_EDGE ( 'NONE', *, *, #15735, .T. ) ;
#19048=VECTOR ( 'NONE', #15457, 1000.000000000000000 ) ;
#19052=VECTOR ( 'NONE', #1968, 1000.000000000000000 ) ;
#19057=VERTEX_POINT ( 'NONE', #12394 ) ;
#19058=ADVANCED_FACE ( 'NONE', ( #23246 ), #28581, .F. ) ;
#19059=DIRECTION ( 'NONE',  ( 1.000000000000000000, 0.000000000000000000, 0.000000000000000000 ) ) ;
#19065=CARTESIAN_POINT ( 'NONE',  ( -21.67835495107042476, 31.04982069277124879, -36.68877005347593467 ) ) ;
#19085=ORIENTED_EDGE ( 'NONE', *, *, #32094, .T. ) ;
#19092=DIRECTION ( 'NONE',  ( 1.000000000000000000, 0.000000000000000000, 0.000000000000000000 ) ) ;
#19101=CARTESIAN_POINT ( 'NONE',  ( 29.44023756548695658, 13.87360028845404614, 68.31122994652405112 ) ) ;
#19104=FACE_OUTER_BOUND ( 'NONE', #15527, .T. ) ;
#19112=FACE_OUTER_BOUND ( 'NONE', #6297, .T. ) ;
#19113=DIRECTION ( 'NONE',  ( 0.7621620551276367950, 0.6473862847818272481, -0.000000000000000000 ) ) ;
#19115=EDGE_CURVE ( 'NONE', #16741, #5474, #15128, .T. ) ;
#19116=CARTESIAN_POINT ( 'NONE',  ( -20.02113311122478123, 18.16264470403145381, -87.50000000000000000 ) ) ;
#19121=EDGE_CURVE ( 'NONE', #28732, #34550, #12919, .T. ) ;
#19127=FACE_BOUND ( 'NONE', #27460, .T. ) ;
#19130=DIRECTION ( 'NONE',  ( -0.7960930657056438653, 0.6051742151937650194, 1.111686998345334199E-16 ) ) ;
#19135=AXIS2_PLACEMENT_3D ( 'NONE', #34437, #10398, #32106 ) ;
#19136=EDGE_LOOP ( 'NONE', ( #20003, #6622, #9796, #30877 ) ) ;
#19137=EDGE_LOOP ( 'NONE', ( #9567, #23031, #13634, #24613 ) ) ;
#19143=AXIS2_PLACEMENT_3D ( 'NONE', #30278, #738, #11074 ) ;
#19149=DIRECTION ( 'NONE',  ( 0.000000000000000000, -0.5288966977476834419, -0.8486862100397269959 ) ) ;
#19153=EDGE_CURVE ( 'NONE', #16922, #13770, #35015, .T. ) ;
#19160=ORIENTED_EDGE ( 'NONE', *, *, #16292, .T. ) ;
#19161=CARTESIAN_POINT ( 'NONE',  ( -5.021133111224679091, 26.05646109878476224, -67.50000000000000000 ) ) ;
#19164=ORIENTED_EDGE ( 'NONE', *, *, #19823, .F. ) ;
#19168=CARTESIAN_POINT ( 'NONE',  ( -5.021133111225092982, -15.68591377522703745, -67.50000000000000000 ) ) ;
#19170=ORIENTED_EDGE ( 'NONE', *, *, #17357, .F. ) ;
#19171=VERTEX_POINT ( 'NONE', #13436 ) ;
#19174=EDGE_CURVE ( 'NONE', #15297, #1165, #24269, .T. ) ;
#19176=ADVANCED_FACE ( 'NONE', ( #21083 ), #4688, .F. ) ;
#19177=LINE ( 'NONE', #5607, #11817 ) ;
#19183=CARTESIAN_POINT ( 'NONE',  ( 0.000000000000000000, 2.281310696040539424E-14, -36.68877005347594178 ) ) ;
#19186=CARTESIAN_POINT ( 'NONE',  ( -14.84098889165989377, 28.96462362251111244, 68.31122994652405112 ) ) ;
#19189=ORIENTED_EDGE ( 'NONE', *, *, #8629, .F. ) ;
#19190=CARTESIAN_POINT ( 'NONE',  ( 0.000000000000000000, 3.524919873834583163E-15, 68.31122994652405112 ) ) ;
#19193=ORIENTED_EDGE ( 'NONE', *, *, #1926, .T. ) ;
#19196=ADVANCED_FACE ( 'NONE', ( #24090 ), #7542, .F. ) ;
#19202=ORIENTED_EDGE ( 'NONE', *, *, #10808, .T. ) ;
#19211=EDGE_LOOP ( 'NONE', ( #26270, #13605, #17663, #26337 ) ) ;
#19212=CARTESIAN_POINT ( 'NONE',  ( 24.11848021413632992, 29.19488569250028220, 68.31122994652405112 ) ) ;
#19216=EDGE_CURVE ( 'NONE', #5102, #12124, #433, .T. ) ;
#19225=VECTOR ( 'NONE', #12229, 1000.000000000000000 ) ;
#19227=ORIENTED_EDGE ( 'NONE', *, *, #6958, .F. ) ;
#19239=DIRECTION ( 'NONE',  ( -0.000000000000000000, -1.836970198721029688E-16, 1.000000000000000000 ) ) ;
#19240=LINE ( 'NONE', #15877, #16033 ) ;
#19241=PLANE ( 'NONE',  #4160 ) ;
#19246=DIRECTION ( 'NONE',  ( 1.000000000000000000, 0.000000000000000000, 0.000000000000000000 ) ) ;
#19257=EDGE_CURVE ( 'NONE', #29040, #19647, #3087, .T. ) ;
#19258=VECTOR ( 'NONE', #28872, 1000.000000000000000 ) ;
#19261=EDGE_CURVE ( 'NONE', #26118, #27945, #22319, .T. ) ;
#19268=ORIENTED_EDGE ( 'NONE', *, *, #24823, .F. ) ;
#19270=FACE_OUTER_BOUND ( 'NONE', #24434, .T. ) ;
#19273=CYLINDRICAL_SURFACE ( 'NONE', #2303, 2.033421858999711951 ) ;
#19274=DIRECTION ( 'NONE',  ( 0.000000000000000000, 1.836970198721029441E-16, -1.000000000000000000 ) ) ;
#19277=LINE ( 'NONE', #8745, #10102 ) ;
#19280=DIRECTION ( 'NONE',  ( -0.9941379571543593752, 0.1081190184239433083, 0.000000000000000000 ) ) ;
#19282=PLANE ( 'NONE',  #5347 ) ;
#19290=ORIENTED_EDGE ( 'NONE', *, *, #10876, .F. ) ;
#19304=ORIENTED_EDGE ( 'NONE', *, *, #30830, .T. ) ;
#19309=ADVANCED_FACE ( 'NONE', ( #16828 ), #19839, .F. ) ;
#19315=DIRECTION ( 'NONE',  ( -1.000000000000000000, 6.792721752314501023E-48, -3.697785493223492838E-32 ) ) ;
#19317=CARTESIAN_POINT ( 'NONE',  ( -5.038454199367317088, -32.15304576796697233, 68.31122994652405112 ) ) ;
#19319=FACE_OUTER_BOUND ( 'NONE', #22885, .T. ) ;
#19328=AXIS2_PLACEMENT_3D ( 'NONE', #9099, #30643, #33310 ) ;
#19330=DIRECTION ( 'NONE',  ( -0.2675283385292216987, 0.9635499925192227977, 0.000000000000000000 ) ) ;
#19332=ORIENTED_EDGE ( 'NONE', *, *, #19121, .F. ) ;
#19334=ORIENTED_EDGE ( 'NONE', *, *, #13033, .T. ) ;
#19340=EDGE_CURVE ( 'NONE', #17151, #5081, #31596, .T. ) ;
#19341=VECTOR ( 'NONE', #27597, 1000.000000000000000 ) ;
#19345=EDGE_CURVE ( 'NONE', #319, #11101, #11159, .T. ) ;
#19349=CARTESIAN_POINT ( 'NONE',  ( -5.021133111224782120, 16.12922284503174097, -87.50000000000000000 ) ) ;
#19351=CARTESIAN_POINT ( 'NONE',  ( 0.000000000000000000, 3.524919873834583163E-15, 68.31122994652405112 ) ) ;
#19356=VERTEX_POINT ( 'NONE', #24971 ) ;
#19363=ORIENTED_EDGE ( 'NONE', *, *, #26354, .F. ) ;
#19364=CARTESIAN_POINT ( 'NONE',  ( -5.038454199367317088, -32.15304576796695102, -36.68877005347593467 ) ) ;
#19370=ORIENTED_EDGE ( 'NONE', *, *, #22980, .F. ) ;
#19374=EDGE_CURVE ( 'NONE', #10833, #23287, #12518, .T. ) ;
#19382=CARTESIAN_POINT ( 'NONE',  ( -35.71762877834949990, -12.58147180936567011, 68.31122994652405112 ) ) ;
#19392=DIRECTION ( 'NONE',  ( -0.8568571761675904952, 0.5155538571770196254, 0.000000000000000000 ) ) ;
#19396=ORIENTED_EDGE ( 'NONE', *, *, #30229, .T. ) ;
#19397=ORIENTED_EDGE ( 'NONE', *, *, #30216, .F. ) ;
#19402=ORIENTED_EDGE ( 'NONE', *, *, #858, .F. ) ;
#19404=CARTESIAN_POINT ( 'NONE',  ( -35.00000000000000000, 3.353962854566122864, -15.81122994652406355 ) ) ;
#19410=CARTESIAN_POINT ( 'NONE',  ( -9.144464960067640646, -31.23432620483745836, 68.31122994652405112 ) ) ;
#19419=EDGE_CURVE ( 'NONE', #9979, #10097, #33302, .T. ) ;
#19422=CARTESIAN_POINT ( 'NONE',  ( 0.000000000000000000, -33.69708579775585378, -36.68877005347594178 ) ) ;
#19424=EDGE_CURVE ( 'NONE', #9180, #12202, #6453, .T. ) ;
#19435=DIRECTION ( 'NONE',  ( -0.05413890858541786644, 0.9985334138511238189, 0.000000000000000000 ) ) ;
#19439=VERTEX_POINT ( 'NONE', #15018 ) ;
#19444=PLANE ( 'NONE',  #29185 ) ;
#19445=ORIENTED_EDGE ( 'NONE', *, *, #8629, .T. ) ;
#19447=CARTESIAN_POINT ( 'NONE',  ( 5.021133111224369117, -3.725253662474303784, -67.50000000000000000 ) ) ;
#19451=PLANE ( 'NONE',  #32254 ) ;
#19460=VECTOR ( 'NONE', #5623, 1000.000000000000114 ) ;
#19465=ORIENTED_EDGE ( 'NONE', *, *, #31516, .F. ) ;
#19468=ORIENTED_EDGE ( 'NONE', *, *, #30577, .T. ) ;
#19470=EDGE_LOOP ( 'NONE', ( #252, #23422, #21515, #16894 ) ) ;
#19474=VECTOR ( 'NONE', #27280, 1000.000000000000114 ) ;
#19482=AXIS2_PLACEMENT_3D ( 'NONE', #5584, #449, #8272 ) ;
#19484=CARTESIAN_POINT ( 'NONE',  ( 17.27856612038524631, 33.69708579775584667, 68.31122994652405112 ) ) ;
#19485=CARTESIAN_POINT ( 'NONE',  ( -37.12776225901827587, -7.411627343331159246, 68.31122994652405112 ) ) ;
#19493=CARTESIAN_POINT ( 'NONE',  ( -5.021133111225196011, -25.61315202898006049, -67.50000000000000000 ) ) ;
#19502=EDGE_CURVE ( 'NONE', #10848, #4890, #6632, .T. ) ;
#19503=PLANE ( 'NONE',  #33024 ) ;
#19511=EDGE_CURVE ( 'NONE', #12135, #3029, #14848, .T. ) ;
#19514=EDGE_LOOP ( 'NONE', ( #15177, #32486, #11883, #24128 ) ) ;
#19515=DIRECTION ( 'NONE',  ( 0.000000000000000000, 1.000000000000000000, 0.000000000000000000 ) ) ;
#19516=DIRECTION ( 'NONE',  ( -0.9985334138511239299, 0.05413890858541753337, 0.000000000000000000 ) ) ;
#19517=ORIENTED_EDGE ( 'NONE', *, *, #25004, .T. ) ;
#19518=ORIENTED_EDGE ( 'NONE', *, *, #34922, .F. ) ;
#19521=VECTOR ( 'NONE', #22514, 1000.000000000000114 ) ;
#19523=LINE ( 'NONE', #20052, #25055 ) ;
#19527=LINE ( 'NONE', #8650, #31687 ) ;
#19531=CARTESIAN_POINT ( 'NONE',  ( -8.267476927982267298, 31.47782073335735831, 68.31122994652405112 ) ) ;
#19533=DIRECTION ( 'NONE',  ( -0.2149704402110243495, -0.9766205557100865464, 0.000000000000000000 ) ) ;
#19537=CYLINDRICAL_SURFACE ( 'NONE', #2357, 2.033421858999711951 ) ;
#19542=VERTEX_POINT ( 'NONE', #21399 ) ;
#19546=EDGE_CURVE ( 'NONE', #24034, #2524, #4828, .T. ) ;
#19548=EDGE_CURVE ( 'NONE', #22594, #33860, #8035, .T. ) ;
#19558=ORIENTED_EDGE ( 'NONE', *, *, #1873, .T. ) ;
#19562=DIRECTION ( 'NONE',  ( 0.000000000000000000, 1.836970198721029441E-16, -1.000000000000000000 ) ) ;
#19564=ORIENTED_EDGE ( 'NONE', *, *, #5181, .F. ) ;
#19571=FACE_OUTER_BOUND ( 'NONE', #18970, .T. ) ;
#19573=ORIENTED_EDGE ( 'NONE', *, *, #25091, .T. ) ;
#19580=ORIENTED_EDGE ( 'NONE', *, *, #14028, .T. ) ;
#19588=DIRECTION ( 'NONE',  ( 0.000000000000000000, -1.000000000000000000, -2.132064625830773463E-16 ) ) ;
#19589=CARTESIAN_POINT ( 'NONE',  ( -20.02113311122509032, -11.61907005722761532, -67.50000000000000000 ) ) ;
#19601=ORIENTED_EDGE ( 'NONE', *, *, #13623, .F. ) ;
#19605=VECTOR ( 'NONE', #22624, 1000.000000000000000 ) ;
#19614=EDGE_CURVE ( 'NONE', #29028, #15121, #18217, .T. ) ;
#19621=PLANE ( 'NONE',  #23667 ) ;
#19623=CARTESIAN_POINT ( 'NONE',  ( 10.00000000000000000, 2.296212748401288367E-15, 47.49999999999999289 ) ) ;
#19626=VERTEX_POINT ( 'NONE', #394 ) ;
#19629=LINE ( 'NONE', #11968, #12914 ) ;
#19632=DIRECTION ( 'NONE',  ( 0.000000000000000000, 0.000000000000000000, 1.000000000000000000 ) ) ;
#19635=CARTESIAN_POINT ( 'NONE',  ( 5.021133111224265200, -11.61907005722761532, -67.50000000000000000 ) ) ;
#19638=CIRCLE ( 'NONE', #288, 32.54542015209057126 ) ;
#19642=CARTESIAN_POINT ( 'NONE',  ( -35.00000000000000000, 11.30824010203864916, 28.57494248152496397 ) ) ;
#19643=DIRECTION ( 'NONE',  ( 1.000000000000000000, 0.000000000000000000, 0.000000000000000000 ) ) ;
#19647=VERTEX_POINT ( 'NONE', #11418 ) ;
#19649=VECTOR ( 'NONE', #3276, 1000.000000000000227 ) ;
#19653=ORIENTED_EDGE ( 'NONE', *, *, #3556, .T. ) ;
#19657=ADVANCED_FACE ( 'NONE', ( #19270 ), #8561, .F. ) ;
#19658=ORIENTED_EDGE ( 'NONE', *, *, #7303, .T. ) ;
#19663=DIRECTION ( 'NONE',  ( 0.000000000000000000, 1.000000000000000000, 0.000000000000000000 ) ) ;
#19664=FACE_OUTER_BOUND ( 'NONE', #29630, .T. ) ;
#19665=VECTOR ( 'NONE', #18762, 1000.000000000000000 ) ;
#19669=ORIENTED_EDGE ( 'NONE', *, *, #7009, .T. ) ;
#19670=CARTESIAN_POINT ( 'NONE',  ( -35.00000000000000000, 3.353962854566122864, 15.81122994652406355 ) ) ;
#19671=CARTESIAN_POINT ( 'NONE',  ( 6.857172176539690689, 37.23415287044795718, -36.68877005347593467 ) ) ;
#19673=DIRECTION ( 'NONE',  ( 0.6051742151937650194, -0.7960930657056438653, 0.000000000000000000 ) ) ;
#19674=CARTESIAN_POINT ( 'NONE',  ( -18.38714294329533416, -33.09555747561019245, -36.68877005347593467 ) ) ;
#19682=VECTOR ( 'NONE', #27297, 1000.000000000000000 ) ;
#19686=CARTESIAN_POINT ( 'NONE',  ( 1.532562817202168137, 33.69708579775584667, -36.68877005347592757 ) ) ;
#19697=VECTOR ( 'NONE', #13397, 1000.000000000000000 ) ;
#19698=EDGE_CURVE ( 'NONE', #18691, #32277, #16600, .T. ) ;
#19706=LINE ( 'NONE', #17406, #23731 ) ;
#19708=DIRECTION ( 'NONE',  ( -0.000000000000000000, -0.000000000000000000, 1.000000000000000000 ) ) ;
#19714=FACE_OUTER_BOUND ( 'NONE', #9117, .T. ) ;
#19718=LINE ( 'NONE', #318, #33720 ) ;
#19724=ORIENTED_EDGE ( 'NONE', *, *, #8588, .F. ) ;
#19727=DIRECTION ( 'NONE',  ( -0.9766205557100871015, -0.2149704402110223789, -0.000000000000000000 ) ) ;
#19731=VERTEX_POINT ( 'NONE', #8739 ) ;
#19733=ADVANCED_FACE ( 'NONE', ( #24572 ), #24928, .F. ) ;
#19734=DIRECTION ( 'NONE',  ( -1.000000000000000000, 0.000000000000000000, 0.000000000000000000 ) ) ;
#19742=EDGE_CURVE ( 'NONE', #11336, #22309, #17128, .T. ) ;
#19753=ADVANCED_FACE ( 'NONE', ( #13918 ), #19621, .F. ) ;
#19758=CARTESIAN_POINT ( 'NONE',  ( -9.978866888775426602, 14.09580098603202636, -87.50000000000000000 ) ) ;
#19759=ORIENTED_EDGE ( 'NONE', *, *, #11403, .T. ) ;
#19762=PLANE ( 'NONE',  #11526 ) ;
#19767=CARTESIAN_POINT ( 'NONE',  ( 12.73347502555019162, -33.69708579775584667, 68.31122994652405112 ) ) ;
#19775=VERTEX_POINT ( 'NONE', #8210 ) ;
#19778=ORIENTED_EDGE ( 'NONE', *, *, #222, .T. ) ;
#19784=CARTESIAN_POINT ( 'NONE',  ( -9.978866888775527855, 4.168562732279007754, -87.50000000000000000 ) ) ;
#19792=EDGE_LOOP ( 'NONE', ( #5748, #13660, #25867, #31435, #8631, #29217 ) ) ;
#19793=ADVANCED_FACE ( 'NONE', ( #27784 ), #5529, .F. ) ;
#19794=EDGE_CURVE ( 'NONE', #18985, #27567, #14277, .T. ) ;
#19801=LINE ( 'NONE', #30649, #21490 ) ;
#19807=PLANE ( 'NONE',  #26781 ) ;
#19812=DIRECTION ( 'NONE',  ( 0.000000000000000000, -0.8486862100397269959, 0.5288966977476833309 ) ) ;
#19817=EDGE_CURVE ( 'NONE', #22594, #9350, #15145, .T. ) ;
#19823=EDGE_CURVE ( 'NONE', #16210, #26021, #23162, .T. ) ;
#19831=AXIS2_PLACEMENT_3D ( 'NONE', #14013, #22553, #17411 ) ;
#19837=ORIENTED_EDGE ( 'NONE', *, *, #4722, .T. ) ;
#19838=EDGE_CURVE ( 'NONE', #20533, #10877, #6592, .T. ) ;
#19839=PLANE ( 'NONE',  #6587 ) ;
#19840=PLANE ( 'NONE',  #14112 ) ;
#19841=PLANE ( 'NONE',  #28946 ) ;
#19845=CARTESIAN_POINT ( 'NONE',  ( 21.24400529595486020, -24.65555945140047811, 68.31122994652405112 ) ) ;
#19849=DIRECTION ( 'NONE',  ( 0.9635499925192231307, 0.2675283385292199223, -0.000000000000000000 ) ) ;
#19850=DIRECTION ( 'NONE',  ( -1.000000000000000000, 0.000000000000000000, 0.000000000000000000 ) ) ;
#19851=CARTESIAN_POINT ( 'NONE',  ( 3.235562306570555532E-30, -11.61907005722761532, -67.50000000000000000 ) ) ;
#19862=EDGE_CURVE ( 'NONE', #32966, #4316, #31330, .T. ) ;
#19863=ORIENTED_EDGE ( 'NONE', *, *, #415, .T. ) ;
#19865=DIRECTION ( 'NONE',  ( -0.000000000000000000, -0.000000000000000000, 1.000000000000000000 ) ) ;
#19869=EDGE_CURVE ( 'NONE', #21129, #20981, #28491, .T. ) ;
#19870=ORIENTED_EDGE ( 'NONE', *, *, #13051, .T. ) ;
#19875=DIRECTION ( 'NONE',  ( -1.000000000000000000, 6.792721752314501023E-48, -3.697785493223492838E-32 ) ) ;
#19876=AXIS2_PLACEMENT_3D ( 'NONE', #34742, #26549, #20225 ) ;
#19882=CARTESIAN_POINT ( 'NONE',  ( 3.235562306570555532E-30, 1.325223266901699007E-14, -67.50000000000000000 ) ) ;
#19888=EDGE_LOOP ( 'NONE', ( #16484, #24112, #4817, #4463 ) ) ;
#19892=CARTESIAN_POINT ( 'NONE',  ( -2.216215597024039141, -32.46987467335852529, 68.31122994652405112 ) ) ;
#19896=ORIENTED_EDGE ( 'NONE', *, *, #19502, .F. ) ;
#19898=CARTESIAN_POINT ( 'NONE',  ( -36.04853892210773836, 11.59936550071286376, 68.31122994652405112 ) ) ;
#19902=ORIENTED_EDGE ( 'NONE', *, *, #7865, .F. ) ;
#19909=FACE_OUTER_BOUND ( 'NONE', #22573, .T. ) ;
#19910=ORIENTED_EDGE ( 'NONE', *, *, #6533, .F. ) ;
#19920=CARTESIAN_POINT ( 'NONE',  ( -37.12776225901827587, -7.411627343331159246, 68.31122994652405112 ) ) ;
#19921=ORIENTED_EDGE ( 'NONE', *, *, #6250, .F. ) ;
#19924=DIRECTION ( 'NONE',  ( -0.4684084406997904848, 0.8835120444460226041, 0.000000000000000000 ) ) ;
#19929=VECTOR ( 'NONE', #27072, 1000.000000000000227 ) ;
#19935=DIRECTION ( 'NONE',  ( 0.9635499925192227977, -0.2675283385292215321, -4.914415851915309929E-17 ) ) ;
#19937=CARTESIAN_POINT ( 'NONE',  ( 32.05156013847309993, -20.15193397489277771, 68.31122994652405112 ) ) ;
#19938=EDGE_CURVE ( 'NONE', #8857, #15892, #30813, .T. ) ;
#19939=AXIS2_PLACEMENT_3D ( 'NONE', #19920, #28095, #6893 ) ;
#19955=DIRECTION ( 'NONE',  ( 0.6876994588534230957, 0.7259954919231310644, 0.000000000000000000 ) ) ;
#19960=ORIENTED_EDGE ( 'NONE', *, *, #24314, .F. ) ;
#19961=VERTEX_POINT ( 'NONE', #1091 ) ;
#19965=PLANE ( 'NONE',  #19328 ) ;
#19966=CARTESIAN_POINT ( 'NONE',  ( 5.510910596163087978E-15, 45.00000000000000711, -36.68877005347593467 ) ) ;
#19967=CARTESIAN_POINT ( 'NONE',  ( 5.021133111224162171, -25.61315202898006049, -67.50000000000000000 ) ) ;
#19968=VERTEX_POINT ( 'NONE', #33653 ) ;
#19976=DIRECTION ( 'NONE',  ( 0.3701381553399144542, 0.9289767198167914186, 1.706502549609061988E-16 ) ) ;
#19978=CARTESIAN_POINT ( 'NONE',  ( -35.00000000000000000, -4.831299144296466785, 15.81122994652406355 ) ) ;
#19988=VECTOR ( 'NONE', #28670, 1000.000000000000114 ) ;
#19989=EDGE_CURVE ( 'NONE', #17757, #20342, #28142, .T. ) ;
#19996=DIRECTION ( 'NONE',  ( 0.000000000000000000, 1.000000000000000000, 0.000000000000000000 ) ) ;
#19997=ORIENTED_EDGE ( 'NONE', *, *, #3857, .T. ) ;
#19999=PLANE ( 'NONE',  #30995 ) ;
#20003=ORIENTED_EDGE ( 'NONE', *, *, #21135, .T. ) ;
#20006=VERTEX_POINT ( 'NONE', #28833 ) ;
#20007=ORIENTED_EDGE ( 'NONE', *, *, #7358, .F. ) ;
#20009=CARTESIAN_POINT ( 'NONE',  ( 35.63428259149704758, -12.79065496477508823, 68.31122994652405112 ) ) ;
#20017=EDGE_CURVE ( 'NONE', #10008, #9180, #11775, .T. ) ;
#20018=LINE ( 'NONE', #22153, #33483 ) ;
#20024=DIRECTION ( 'NONE',  ( 0.000000000000000000, 0.000000000000000000, 1.000000000000000000 ) ) ;
#20027=FACE_OUTER_BOUND ( 'NONE', #3966, .T. ) ;
#20029=ORIENTED_EDGE ( 'NONE', *, *, #16765, .F. ) ;
#20034=EDGE_CURVE ( 'NONE', #1172, #4776, #24191, .T. ) ;
#20035=EDGE_CURVE ( 'NONE', #13424, #33264, #18535, .T. ) ;
#20040=EDGE_CURVE ( 'NONE', #802, #5820, #31671, .T. ) ;
#20044=AXIS2_PLACEMENT_3D ( 'NONE', #2760, #10959, #34826 ) ;
#20046=CARTESIAN_POINT ( 'NONE',  ( 37.55078559520313775, -4.831299144296470338, 68.31122994652405112 ) ) ;
#20047=EDGE_LOOP ( 'NONE', ( #31460, #13673, #28363, #31371 ) ) ;
#20048=VERTEX_POINT ( 'NONE', #2478 ) ;
#20052=CARTESIAN_POINT ( 'NONE',  ( 3.235562306570555532E-30, -11.61907005722761532, -67.50000000000000000 ) ) ;
#20056=DIRECTION ( 'NONE',  ( 0.2675283385292205884, -0.9635499925192231307, -1.770012621235684308E-16 ) ) ;
#20072=AXIS2_PLACEMENT_3D ( 'NONE', #3886, #15996, #31815 ) ;
#20074=EDGE_CURVE ( 'NONE', #8590, #9716, #10507, .T. ) ;
#20077=CARTESIAN_POINT ( 'NONE',  ( 32.54460952423470133, 0.2297037030477266373, 68.31122994652405112 ) ) ;
#20092=AXIS2_PLACEMENT_3D ( 'NONE', #2675, #26359, #1976 ) ;
#20093=ORIENTED_EDGE ( 'NONE', *, *, #6737, .F. ) ;
#20094=VERTEX_POINT ( 'NONE', #18352 ) ;
#20098=EDGE_CURVE ( 'NONE', #3490, #16456, #21538, .T. ) ;
#20099=EDGE_CURVE ( 'NONE', #15441, #26021, #1778, .T. ) ;
#20101=DIRECTION ( 'NONE',  ( -1.000000000000000000, 6.792721752314501023E-48, -3.697785493223492838E-32 ) ) ;
#20103=LINE ( 'NONE', #33794, #6640 ) ;
#20104=DIRECTION ( 'NONE',  ( 0.7960930657056439763, 0.6051742151937649083, 1.111686998345333706E-16 ) ) ;
#20106=CARTESIAN_POINT ( 'NONE',  ( -5.021133111225092982, -13.65249191622732816, -67.50000000000000000 ) ) ;
#20107=DIRECTION ( 'NONE',  ( 0.7259954919231307313, 0.6876994588534234287, -0.000000000000000000 ) ) ;
#20121=LINE ( 'NONE', #6748, #16617 ) ;
#20123=VERTEX_POINT ( 'NONE', #21364 ) ;
#20133=EDGE_CURVE ( 'NONE', #27831, #24340, #9972, .T. ) ;
#20137=CARTESIAN_POINT ( 'NONE',  ( -23.93921925319781963, 29.33115633223345142, 68.31122994652405112 ) ) ;
#20140=ORIENTED_EDGE ( 'NONE', *, *, #6124, .F. ) ;
#20142=CIRCLE ( 'NONE', #4760, 10.87635688602997597 ) ;
#20150=CARTESIAN_POINT ( 'NONE',  ( 22.10765473302597073, -14.55883922869198344, -77.50000000000000000 ) ) ;
#20154=DIRECTION ( 'NONE',  ( 0.000000000000000000, 1.836970198721029441E-16, -1.000000000000000000 ) ) ;
#20158=VECTOR ( 'NONE', #7058, 1000.000000000000000 ) ;
#20169=AXIS2_PLACEMENT_3D ( 'NONE', #11370, #5826, #6180 ) ;
#20173=VERTEX_POINT ( 'NONE', #32023 ) ;
#20174=ORIENTED_EDGE ( 'NONE', *, *, #902, .T. ) ;
#20188=DIRECTION ( 'NONE',  ( 0.000000000000000000, -1.000000000000000000, -1.836970198721029934E-16 ) ) ;
#20191=VERTEX_POINT ( 'NONE', #24717 ) ;
#20194=LINE ( 'NONE', #6641, #26466 ) ;
#20196=ADVANCED_FACE ( 'NONE', ( #5315 ), #21878, .F. ) ;
#20203=CARTESIAN_POINT ( 'NONE',  ( -30.76765767668601725, -10.60922306139171667, 68.31122994652405112 ) ) ;
#20208=ORIENTED_EDGE ( 'NONE', *, *, #32655, .T. ) ;
#20211=VECTOR ( 'NONE', #18907, 1000.000000000000227 ) ;
#20212=EDGE_LOOP ( 'NONE', ( #29124, #30010, #28111, #29795 ) ) ;
#20215=VECTOR ( 'NONE', #30024, 1000.000000000000000 ) ;
#20223=CARTESIAN_POINT ( 'NONE',  ( 5.021133111224576062, 14.09580098603202458, -67.50000000000000000 ) ) ;
#20225=DIRECTION ( 'NONE',  ( 1.000000000000000000, 0.000000000000000000, 0.000000000000000000 ) ) ;
#20228=CARTESIAN_POINT ( 'NONE',  ( 0.000000000000000000, 3.524919873834583163E-15, 68.31122994652405112 ) ) ;
#20233=CARTESIAN_POINT ( 'NONE',  ( -37.85301660235036536, 0.7430237821112573027, 68.31122994652405112 ) ) ;
#20235=CARTESIAN_POINT ( 'NONE',  ( -20.02113311122509032, -15.68591377522703745, -67.50000000000000000 ) ) ;
#20255=CYLINDRICAL_SURFACE ( 'NONE', #16077, 44.99999999999997868 ) ;
#20260=VECTOR ( 'NONE', #9317, 1000.000000000000000 ) ;
#20268=LINE ( 'NONE', #34299, #6085 ) ;
#20270=ORIENTED_EDGE ( 'NONE', *, *, #27164, .F. ) ;
#20274=DIRECTION ( 'NONE',  ( 0.000000000000000000, 1.836970198721029688E-16, -1.000000000000000000 ) ) ;
#20286=EDGE_LOOP ( 'NONE', ( #4473, #26560, #5124, #30752 ) ) ;
#20287=VECTOR ( 'NONE', #3144, 1000.000000000000000 ) ;
#20288=CARTESIAN_POINT ( 'NONE',  ( 5.390701026406702567, -37.47456861236020131, 68.31122994652405112 ) ) ;
#20294=CARTESIAN_POINT ( 'NONE',  ( 34.58310883014599568, -15.42890216704097206, 68.31122994652405112 ) ) ;
#20297=EDGE_LOOP ( 'NONE', ( #20821, #18595, #32905, #8148, #4495, #5231, #22582, #6213, #4325, #18534, #34205, #11408, #27848, #11017, #6054, #24346, #30464, #10647, #7818, #92, #4637, #32928, #357, #6729, #17685, #27987, #9574, #14931, #32194, #17798, #21285, #14518, #11910, #35037, #12377, #25947, #6048, #21483, #3362, #23701, #8861, #34528, #25404, #18164, #23310, #25243 ) ) ;
#20305=CIRCLE ( 'NONE', #4344, 2.033421858999711951 ) ;
#20307=CARTESIAN_POINT ( 'NONE',  ( -32.37866696771086339, 3.290334066652078171, 68.31122994652405112 ) ) ;
#20311=CARTESIAN_POINT ( 'NONE',  ( -30.91434716440808472, 10.17386417614053151, 68.31122994652405112 ) ) ;
#20319=ORIENTED_EDGE ( 'NONE', *, *, #17593, .F. ) ;
#20325=LINE ( 'NONE', #14816, #1781 ) ;
#20326=DIRECTION ( 'NONE',  ( 0.9289767198167914186, -0.3701381553399144542, 0.000000000000000000 ) ) ;
#20327=CARTESIAN_POINT ( 'NONE',  ( 0.000000000000000000, -32.54542015209057126, 87.50000000000000000 ) ) ;
#20328=LINE ( 'NONE', #1623, #28188 ) ;
#20334=PLANE ( 'NONE',  #4785 ) ;
#20336=EDGE_CURVE ( 'NONE', #7906, #1533, #20305, .T. ) ;
#20342=VERTEX_POINT ( 'NONE', #17791 ) ;
#20343=VECTOR ( 'NONE', #18988, 1000.000000000000000 ) ;
#20346=VERTEX_POINT ( 'NONE', #14419 ) ;
#20362=CARTESIAN_POINT ( 'NONE',  ( 8.986540508143576744, 33.69708579775584667, -36.68877005347592757 ) ) ;
#20371=DIRECTION ( 'NONE',  ( 0.000000000000000000, 1.836970198721029441E-16, -1.000000000000000000 ) ) ;
#20374=LINE ( 'NONE', #1153, #33265 ) ;
#20378=ORIENTED_EDGE ( 'NONE', *, *, #28651, .F. ) ;
#20380=DIRECTION ( 'NONE',  ( -0.000000000000000000, 1.836970198721029688E-16, -1.000000000000000000 ) ) ;
#20385=VECTOR ( 'NONE', #28827, 1000.000000000000000 ) ;
#20388=ORIENTED_EDGE ( 'NONE', *, *, #27113, .T. ) ;
#20389=EDGE_CURVE ( 'NONE', #24880, #31033, #20103, .T. ) ;
#20390=ORIENTED_EDGE ( 'NONE', *, *, #20872, .T. ) ;
#20391=DIRECTION ( 'NONE',  ( 0.000000000000000000, 1.000000000000000000, 1.934419779023891545E-16 ) ) ;
#20395=EDGE_CURVE ( 'NONE', #33264, #24034, #17270, .T. ) ;
#20414=VECTOR ( 'NONE', #29855, 1000.000000000000000 ) ;
#20416=ORIENTED_EDGE ( 'NONE', *, *, #31153, .F. ) ;
#20418=VERTEX_POINT ( 'NONE', #9592 ) ;
#20425=PLANE ( 'NONE',  #34408 ) ;
#20428=CIRCLE ( 'NONE', #20980, 32.54542015209056416 ) ;
#20437=DIRECTION ( 'NONE',  ( -0.5155538571770215128, 0.8568571761675894960, 1.574021097180117283E-16 ) ) ;
#20438=DIRECTION ( 'NONE',  ( 0.000000000000000000, 1.836970198721030181E-16, -1.000000000000000000 ) ) ;
#20440=ORIENTED_EDGE ( 'NONE', *, *, #15963, .F. ) ;
#20443=EDGE_CURVE ( 'NONE', #18486, #16556, #29508, .T. ) ;
#20451=EDGE_CURVE ( 'NONE', #21855, #17151, #31466, .T. ) ;
#20466=EDGE_CURVE ( 'NONE', #10873, #11323, #34489, .T. ) ;
#20475=PLANE ( 'NONE',  #30406 ) ;
#20476=DIRECTION ( 'NONE',  ( 1.000000000000000000, -0.000000000000000000, -0.000000000000000000 ) ) ;
#20483=DIRECTION ( 'NONE',  ( -1.000000000000000000, -0.000000000000000000, -0.000000000000000000 ) ) ;
#20485=FACE_OUTER_BOUND ( 'NONE', #9398, .T. ) ;
#20488=EDGE_CURVE ( 'NONE', #5474, #25766, #18662, .T. ) ;
#20489=CARTESIAN_POINT ( 'NONE',  ( -5.038454199367317976, -32.15304576796696523, 68.31122994652405112 ) ) ;
#20495=CARTESIAN_POINT ( 'NONE',  ( 4.979875012683824487, -33.69708579775584667, -36.68877005347592757 ) ) ;
#20496=LINE ( 'NONE', #15698, #17424 ) ;
#20497=CARTESIAN_POINT ( 'NONE',  ( 34.14795412574902400, 16.36947364650383818, 68.31122994652405112 ) ) ;
#20501=CIRCLE ( 'NONE', #3514, 32.54542015209057126 ) ;
#20516=CARTESIAN_POINT ( 'NONE',  ( 35.63428259149704758, -12.79065496477508823, 68.31122994652405112 ) ) ;
#20519=VERTEX_POINT ( 'NONE', #20965 ) ;
#20530=CARTESIAN_POINT ( 'NONE',  ( 5.510910596163087978E-15, 45.00000000000000711, -85.22165320886809070 ) ) ;
#20533=VERTEX_POINT ( 'NONE', #26652 ) ;
#20535=DIRECTION ( 'NONE',  ( -0.9476531711828025673, 0.3193015301359797831, 5.865473952658197586E-17 ) ) ;
#20542=DIRECTION ( 'NONE',  ( 0.000000000000000000, 1.000000000000000000, 0.000000000000000000 ) ) ;
#20543=AXIS2_PLACEMENT_3D ( 'NONE', #8994, #19865, #17559 ) ;
#20559=CARTESIAN_POINT ( 'NONE',  ( 22.89764159710615132, -5.651112684911597128, -77.50000000000000000 ) ) ;
#20563=EDGE_LOOP ( 'NONE', ( #28441, #15220, #2926, #12479 ) ) ;
#20564=EDGE_LOOP ( 'NONE', ( #880, #24190, #20029, #11654 ) ) ;
#20571=CARTESIAN_POINT ( 'NONE',  ( 0.000000000000000000, 0.000000000000000000, 0.000000000000000000 ) ) ;
#20572=EDGE_CURVE ( 'NONE', #32765, #28025, #22018, .T. ) ;
#20576=PLANE ( 'NONE',  #27589 ) ;
#20581=CARTESIAN_POINT ( 'NONE',  ( -5.038454199367317088, -32.15304576796697233, 68.31122994652405112 ) ) ;
#20587=ORIENTED_EDGE ( 'NONE', *, *, #34135, .T. ) ;
#20588=CARTESIAN_POINT ( 'NONE',  ( 0.000000000000000000, 6.992329373473909019E-15, 49.43553178847298568 ) ) ;
#20590=EDGE_CURVE ( 'NONE', #4766, #8764, #126, .T. ) ;
#20591=VECTOR ( 'NONE', #13671, 1000.000000000000114 ) ;
#20595=CARTESIAN_POINT ( 'NONE',  ( 0.000000000000000000, 3.172845296185191895E-14, -85.22165320886810491 ) ) ;
#20596=FACE_OUTER_BOUND ( 'NONE', #15624, .T. ) ;
#20608=ORIENTED_EDGE ( 'NONE', *, *, #2089, .T. ) ;
#20615=DIRECTION ( 'NONE',  ( 3.697785493223492838E-32, 1.934419779023891545E-16, -1.000000000000000000 ) ) ;
#20617=CIRCLE ( 'NONE', #34852, 2.036051781435508801 ) ;
#20620=VECTOR ( 'NONE', #16170, 1000.000000000000000 ) ;
#20640=ORIENTED_EDGE ( 'NONE', *, *, #14231, .F. ) ;
#20641=CIRCLE ( 'NONE', #8687, 2.036051781435517682 ) ;
#20645=CARTESIAN_POINT ( 'NONE',  ( 0.000000000000000000, -32.54542015209051442, -87.50000000000000000 ) ) ;
#20652=VECTOR ( 'NONE', #3802, 1000.000000000000000 ) ;
#20656=ORIENTED_EDGE ( 'NONE', *, *, #19838, .T. ) ;
#20663=CARTESIAN_POINT ( 'NONE',  ( -37.71145559917817280, 3.353962854566121088, -15.81122994652406355 ) ) ;
#20664=VECTOR ( 'NONE', #31394, 1000.000000000000114 ) ;
#20669=CARTESIAN_POINT ( 'NONE',  ( 0.000000000000000000, 3.524919873834583163E-15, 68.31122994652405112 ) ) ;
#20673=CARTESIAN_POINT ( 'NONE',  ( -20.72055270933794446, 25.09707290294329951, 68.31122994652405112 ) ) ;
#20674=DIRECTION ( 'NONE',  ( -0.4198891015602644883, -0.9075754196709571175, -0.000000000000000000 ) ) ;
#20681=ADVANCED_FACE ( 'NONE', ( #27342 ), #3139, .F. ) ;
#20685=EDGE_CURVE ( 'NONE', #25215, #29230, #427, .T. ) ;
#20695=EDGE_LOOP ( 'NONE', ( #810, #4457, #5119, #14571 ) ) ;
#20696=DIRECTION ( 'NONE',  ( 0.000000000000000000, 0.000000000000000000, 1.000000000000000000 ) ) ;
#20699=ORIENTED_EDGE ( 'NONE', *, *, #806, .T. ) ;
#20712=CARTESIAN_POINT ( 'NONE',  ( 1.532562817202168137, 33.69708579775584667, 68.31122994652405112 ) ) ;
#20714=EDGE_CURVE ( 'NONE', #22911, #25849, #16452, .T. ) ;
#20720=CYLINDRICAL_SURFACE ( 'NONE', #28636, 2.036051781435517682 ) ;
#20733=CARTESIAN_POINT ( 'NONE',  ( 2.123179190381537129, -33.69708579775584667, 49.43553178847298568 ) ) ;
#20735=VERTEX_POINT ( 'NONE', #34228 ) ;
#20736=CARTESIAN_POINT ( 'NONE',  ( -15.64512930492131382, -28.53829535743844659, -36.68877005347593467 ) ) ;
#20743=ORIENTED_EDGE ( 'NONE', *, *, #24854, .T. ) ;
#20747=PLANE ( 'NONE',  #8974 ) ;
#20749=CARTESIAN_POINT ( 'NONE',  ( 11.62236370382047745, -30.39942490923500529, 49.43553178847298568 ) ) ;
#20758=ORIENTED_EDGE ( 'NONE', *, *, #8700, .T. ) ;
#20759=CARTESIAN_POINT ( 'NONE',  ( -27.76765758629847980, -16.97532223688792996, 68.31122994652405112 ) ) ;
#20761=CARTESIAN_POINT ( 'NONE',  ( -5.021133111224782120, 18.16264470403145026, -67.50000000000000000 ) ) ;
#20763=LINE ( 'NONE', #31609, #27896 ) ;
#20769=EDGE_CURVE ( 'NONE', #8593, #5081, #6813, .T. ) ;
#20773=ORIENTED_EDGE ( 'NONE', *, *, #23109, .T. ) ;
#20776=ORIENTED_EDGE ( 'NONE', *, *, #9970, .T. ) ;
#20778=DIRECTION ( 'NONE',  ( -0.000000000000000000, -1.836970198721029688E-16, 1.000000000000000000 ) ) ;
#20787=LINE ( 'NONE', #29504, #14258 ) ;
#20793=VECTOR ( 'NONE', #26745, 1000.000000000000000 ) ;
#20798=ORIENTED_EDGE ( 'NONE', *, *, #2238, .F. ) ;
#20799=FACE_OUTER_BOUND ( 'NONE', #5429, .T. ) ;
#20801=CARTESIAN_POINT ( 'NONE',  ( 29.44023756548697079, 13.87360028845406212, 49.43553178847298568 ) ) ;
#20802=FACE_OUTER_BOUND ( 'NONE', #24467, .T. ) ;
#20807=AXIS2_PLACEMENT_3D ( 'NONE', #5103, #24488, #4747 ) ;
#20817=CIRCLE ( 'NONE', #19135, 2.033421858999711951 ) ;
#20821=ORIENTED_EDGE ( 'NONE', *, *, #2412, .F. ) ;
#20822=DIRECTION ( 'NONE',  ( 1.000000000000000000, 0.000000000000000000, -0.000000000000000000 ) ) ;
#20824=VECTOR ( 'NONE', #11607, 1000.000000000000000 ) ;
#20826=CARTESIAN_POINT ( 'NONE',  ( -31.87924797510909869, -6.551177101682105430, -36.68877005347593467 ) ) ;
#20827=VERTEX_POINT ( 'NONE', #28883 ) ;
#20833=LINE ( 'NONE', #7645, #27358 ) ;
#20840=PLANE ( 'NONE',  #26415 ) ;
#20845=CARTESIAN_POINT ( 'NONE',  ( 22.89764159710615132, -3.615060903476079890, -77.50000000000000000 ) ) ;
#20848=VECTOR ( 'NONE', #7993, 1000.000000000000227 ) ;
#20852=VERTEX_POINT ( 'NONE', #15374 ) ;
#20853=EDGE_CURVE ( 'NONE', #2524, #10873, #6663, .T. ) ;
#20859=ORIENTED_EDGE ( 'NONE', *, *, #27911, .T. ) ;
#20861=CARTESIAN_POINT ( 'NONE',  ( -37.69926482250235722, 3.578808500140865156, 68.31122994652405112 ) ) ;
#20866=ORIENTED_EDGE ( 'NONE', *, *, #25825, .F. ) ;
#20867=ORIENTED_EDGE ( 'NONE', *, *, #30126, .F. ) ;
#20872=EDGE_CURVE ( 'NONE', #11484, #33608, #33884, .T. ) ;
#20875=DIRECTION ( 'NONE',  ( 1.000000000000000000, 0.000000000000000000, 0.000000000000000000 ) ) ;
#20878=EDGE_LOOP ( 'NONE', ( #10082, #30140, #12175, #32351 ) ) ;
#20879=CARTESIAN_POINT ( 'NONE',  ( 32.05156013847309993, -20.15193397489277771, 68.31122994652405112 ) ) ;
#20883=VECTOR ( 'NONE', #15108, 1000.000000000000000 ) ;
#20898=VECTOR ( 'NONE', #11084, 1000.000000000000000 ) ;
#20901=ADVANCED_FACE ( 'NONE', ( #18399 ), #2348, .F. ) ;
#20902=VERTEX_POINT ( 'NONE', #7689 ) ;
#20904=ORIENTED_EDGE ( 'NONE', *, *, #10859, .T. ) ;
#20911=CARTESIAN_POINT ( 'NONE',  ( -9.410814080250917257, 36.67205378194066867, -36.68877005347593467 ) ) ;
#20913=CARTESIAN_POINT ( 'NONE',  ( 3.235562306570555532E-30, 18.16264470403145026, -67.50000000000000000 ) ) ;
#20922=VERTEX_POINT ( 'NONE', #34757 ) ;
#20932=VECTOR ( 'NONE', #25982, 1000.000000000000000 ) ;
#20944=ORIENTED_EDGE ( 'NONE', *, *, #6523, .F. ) ;
#20960=CARTESIAN_POINT ( 'NONE',  ( 5.021133111224679091, 26.05646109878476224, -67.50000000000000000 ) ) ;
#20963=DIRECTION ( 'NONE',  ( 0.000000000000000000, 1.836970198721029441E-16, -1.000000000000000000 ) ) ;
#20965=CARTESIAN_POINT ( 'NONE',  ( 10.96230482721425403, -16.64466345897532662, -87.50000000000000000 ) ) ;
#20980=AXIS2_PLACEMENT_3D ( 'NONE', #32846, #16506, #17217 ) ;
#20981=VERTEX_POINT ( 'NONE', #29239 ) ;
#20983=LINE ( 'NONE', #31651, #5380 ) ;
#20984=DIRECTION ( 'NONE',  ( 0.000000000000000000, 0.000000000000000000, 1.000000000000000000 ) ) ;
#20986=AXIS2_PLACEMENT_3D ( 'NONE', #12405, #23415, #14901 ) ;
#20990=LINE ( 'NONE', #31828, #34567 ) ;
#20995=ORIENTED_EDGE ( 'NONE', *, *, #18901, .T. ) ;
#20996=LINE ( 'NONE', #4261, #20932 ) ;
#21002=EDGE_CURVE ( 'NONE', #17675, #5983, #32272, .T. ) ;
#21008=VECTOR ( 'NONE', #10441, 1000.000000000000114 ) ;
#21014=CARTESIAN_POINT ( 'NONE',  ( 22.89764159710615132, -3.615060903476079890, -77.50000000000000000 ) ) ;
#21017=LINE ( 'NONE', #4979, #19052 ) ;
#21019=AXIS2_PLACEMENT_3D ( 'NONE', #12836, #6938, #15154 ) ;
#21025=EDGE_CURVE ( 'NONE', #8593, #21855, #30586, .T. ) ;
#21042=DIRECTION ( 'NONE',  ( 0.000000000000000000, -0.000000000000000000, 1.000000000000000000 ) ) ;
#21044=DIRECTION ( 'NONE',  ( -0.9985334138511239299, -0.05413890858541756113, 0.000000000000000000 ) ) ;
#21050=DIRECTION ( 'NONE',  ( -0.5611870653623822758, -0.8276889981568905652, 0.000000000000000000 ) ) ;
#21051=DIRECTION ( 'NONE',  ( -0.000000000000000000, -0.000000000000000000, -1.000000000000000000 ) ) ;
#21058=EDGE_CURVE ( 'NONE', #22052, #11199, #24935, .T. ) ;
#21059=CARTESIAN_POINT ( 'NONE',  ( -37.55078559520313775, -4.831299144296465897, -15.81122994652406355 ) ) ;
#21072=VERTEX_POINT ( 'NONE', #11424 ) ;
#21076=VECTOR ( 'NONE', #9364, 1000.000000000000114 ) ;
#21078=CARTESIAN_POINT ( 'NONE',  ( -34.66645501699844090, -15.21971901163155216, 68.31122994652405112 ) ) ;
#21079=EDGE_CURVE ( 'NONE', #7819, #19171, #19277, .T. ) ;
#21083=FACE_OUTER_BOUND ( 'NONE', #23349, .T. ) ;
#21086=DIRECTION ( 'NONE',  ( -0.9075754196709575616, -0.4198891015602634891, -0.000000000000000000 ) ) ;
#21088=ORIENTED_EDGE ( 'NONE', *, *, #8700, .F. ) ;
#21096=FACE_OUTER_BOUND ( 'NONE', #4250, .T. ) ;
#21097=ORIENTED_EDGE ( 'NONE', *, *, #21902, .T. ) ;
#21101=EDGE_CURVE ( 'NONE', #17981, #8902, #3052, .T. ) ;
#21103=EDGE_LOOP ( 'NONE', ( #29544, #17126, #13174, #26870 ) ) ;
#21108=EDGE_CURVE ( 'NONE', #14721, #5262, #3401, .T. ) ;
#21119=ORIENTED_EDGE ( 'NONE', *, *, #16988, .T. ) ;
#21122=EDGE_CURVE ( 'NONE', #7363, #28204, #19801, .T. ) ;
#21124=LINE ( 'NONE', #2775, #18733 ) ;
#21129=VERTEX_POINT ( 'NONE', #2643 ) ;
#21130=ORIENTED_EDGE ( 'NONE', *, *, #8588, .T. ) ;
#21132=EDGE_CURVE ( 'NONE', #9350, #6574, #13510, .T. ) ;
#21133=DIRECTION ( 'NONE',  ( -0.9985334138511239299, -0.05413890858541774848, 0.000000000000000000 ) ) ;
#21135=EDGE_CURVE ( 'NONE', #18597, #11323, #5301, .T. ) ;
#21145=ADVANCED_FACE ( 'NONE', ( #2118 ), #24177, .T. ) ;
#21150=AXIS2_PLACEMENT_3D ( 'NONE', #15301, #23301, #15651 ) ;
#21158=VERTEX_POINT ( 'NONE', #10491 ) ;
#21161=LINE ( 'NONE', #34879, #2149 ) ;
#21165=EDGE_CURVE ( 'NONE', #28091, #23681, #21161, .T. ) ;
#21170=VECTOR ( 'NONE', #26927, 1000.000000000000000 ) ;
#21172=EDGE_LOOP ( 'NONE', ( #11492, #15944, #24103, #23015 ) ) ;
#21178=VERTEX_POINT ( 'NONE', #21683 ) ;
#21181=CARTESIAN_POINT ( 'NONE',  ( 37.55078559520313775, -4.831299144296470338, 68.31122994652405112 ) ) ;
#21185=DIRECTION ( 'NONE',  ( 0.7621620551276372391, -0.6473862847818265820, -0.000000000000000000 ) ) ;
#21187=DIRECTION ( 'NONE',  ( 1.000000000000000000, 0.000000000000000000, -0.000000000000000000 ) ) ;
#21191=LINE ( 'NONE', #10521, #21359 ) ;
#21196=DIRECTION ( 'NONE',  ( -0.9941379571543593752, -0.1081190184239432944, 0.000000000000000000 ) ) ;
#21211=DIRECTION ( 'NONE',  ( 0.000000000000000000, 1.000000000000000000, 0.000000000000000000 ) ) ;
#21216=VECTOR ( 'NONE', #18116, 1000.000000000000000 ) ;
#21222=CARTESIAN_POINT ( 'NONE',  ( -35.00000000000000000, -46.95407462254104303, 36.69637551990492597 ) ) ;
#21224=DIRECTION ( 'NONE',  ( 0.000000000000000000, 1.836970198721029441E-16, -1.000000000000000000 ) ) ;
#21225=DIRECTION ( 'NONE',  ( -0.8835120444460229372, -0.4684084406997900407, 0.000000000000000000 ) ) ;
#21226=ORIENTED_EDGE ( 'NONE', *, *, #8466, .F. ) ;
#21228=CARTESIAN_POINT ( 'NONE',  ( -28.00450684652666311, 16.58167570419054115, 68.31122994652405112 ) ) ;
#21242=AXIS2_PLACEMENT_3D ( 'NONE', #27309, #16133, #16843 ) ;
#21243=ORIENTED_EDGE ( 'NONE', *, *, #222, .F. ) ;
#21250=DIRECTION ( 'NONE',  ( -0.05413890858541543089, -0.9985334138511240409, -0.000000000000000000 ) ) ;
#21256=AXIS2_PLACEMENT_3D ( 'NONE', #25182, #18089, #14885 ) ;
#21257=CARTESIAN_POINT ( 'NONE',  ( 0.000000000000000000, 3.524919873834583163E-15, 68.31122994652405112 ) ) ;
#21260=ORIENTED_EDGE ( 'NONE', *, *, #23529, .T. ) ;
#21261=EDGE_CURVE ( 'NONE', #18426, #7713, #7624, .T. ) ;
#21265=CARTESIAN_POINT ( 'NONE',  ( -36.80830595996284416, 8.862931941313787476, -24.65111515542802323 ) ) ;
#21268=CARTESIAN_POINT ( 'NONE',  ( 5.021133111224162171, -23.57973016998034765, -67.50000000000000000 ) ) ;
#21275=ORIENTED_EDGE ( 'NONE', *, *, #6665, .F. ) ;
#21276=AXIS2_PLACEMENT_3D ( 'NONE', #14488, #15317, #26147 ) ;
#21285=ORIENTED_EDGE ( 'NONE', *, *, #16162, .F. ) ;
#21290=ORIENTED_EDGE ( 'NONE', *, *, #21135, .F. ) ;
#21292=CARTESIAN_POINT ( 'NONE',  ( 10.00000000000000000, 2.296212748401288367E-15, 47.49999999999999289 ) ) ;
#21308=ORIENTED_EDGE ( 'NONE', *, *, #23486, .F. ) ;
#21313=DIRECTION ( 'NONE',  ( -0.4198891015602651544, 0.9075754196709567845, 0.000000000000000000 ) ) ;
#21316=CARTESIAN_POINT ( 'NONE',  ( -1.307386931792819285, 37.83772838912469894, 68.31122994652405112 ) ) ;
#21319=CARTESIAN_POINT ( 'NONE',  ( 0.000000000000000000, 3.524919873834583163E-15, 68.31122994652405112 ) ) ;
#21330=DIRECTION ( 'NONE',  ( 0.000000000000000000, 1.836970198721029688E-16, -1.000000000000000000 ) ) ;
#21333=AXIS2_PLACEMENT_3D ( 'NONE', #31222, #22516, #6288 ) ;
#21338=EDGE_LOOP ( 'NONE', ( #2556, #1855, #19465, #35011 ) ) ;
#21339=CARTESIAN_POINT ( 'NONE',  ( 32.30227131129396412, -3.970848902647437395, 68.31122994652405112 ) ) ;
#21359=VECTOR ( 'NONE', #2672, 1000.000000000000227 ) ;
#21360=CARTESIAN_POINT ( 'NONE',  ( 22.10765473302597073, -12.47301499840864025, -77.50000000000000000 ) ) ;
#21364=CARTESIAN_POINT ( 'NONE',  ( 37.09133285470120711, -7.633836879289874311, 68.31122994652405112 ) ) ;
#21366=CARTESIAN_POINT ( 'NONE',  ( -35.00000000000000000, 42.49491490430484220, 36.69637551990492597 ) ) ;
#21371=DIRECTION ( 'NONE',  ( 0.000000000000000000, 1.836970198721029688E-16, -1.000000000000000000 ) ) ;
#21375=CARTESIAN_POINT ( 'NONE',  ( -10.84269519964070305, -36.27449394610876965, -36.68877005347593467 ) ) ;
#21390=VECTOR ( 'NONE', #20483, 1000.000000000000000 ) ;
#21397=EDGE_LOOP ( 'NONE', ( #4714, #24406, #26374, #29962 ) ) ;
#21399=CARTESIAN_POINT ( 'NONE',  ( -32.54223829851970606, 0.4550817492056113966, 68.31122994652405112 ) ) ;
#21400=LINE ( 'NONE', #30107, #31722 ) ;
#21404=CARTESIAN_POINT ( 'NONE',  ( -36.80830595996284416, 8.862931941313773265, 68.31122994652405112 ) ) ;
#21406=ORIENTED_EDGE ( 'NONE', *, *, #2039, .F. ) ;
#21415=EDGE_CURVE ( 'NONE', #22892, #21604, #27091, .T. ) ;
#21416=DIRECTION ( 'NONE',  ( -1.000000000000000000, 0.000000000000000000, 0.000000000000000000 ) ) ;
#21417=LINE ( 'NONE', #8411, #20793 ) ;
#21425=PLANE ( 'NONE',  #15162 ) ;
#21431=VERTEX_POINT ( 'NONE', #16612 ) ;
#21437=FACE_OUTER_BOUND ( 'NONE', #23311, .T. ) ;
#21440=CARTESIAN_POINT ( 'NONE',  ( 5.021133111224162171, -25.61315202898006049, -67.50000000000000000 ) ) ;
#21441=CYLINDRICAL_SURFACE ( 'NONE', #24295, 2.033421858999711507 ) ;
#21447=DIRECTION ( 'NONE',  ( 0.000000000000000000, 1.836970198721029441E-16, -1.000000000000000000 ) ) ;
#21448=VERTEX_POINT ( 'NONE', #6237 ) ;
#21454=EDGE_LOOP ( 'NONE', ( #17910, #11056, #23189, #19658 ) ) ;
#21460=ORIENTED_EDGE ( 'NONE', *, *, #25872, .F. ) ;
#21465=VECTOR ( 'NONE', #12708, 1000.000000000000000 ) ;
#21472=EDGE_CURVE ( 'NONE', #30456, #17724, #22811, .T. ) ;
#21483=ORIENTED_EDGE ( 'NONE', *, *, #4722, .F. ) ;
#21485=EDGE_LOOP ( 'NONE', ( #5887, #12363, #19445, #7353, #27921, #18744 ) ) ;
#21488=DIRECTION ( 'NONE',  ( -0.9766205557100864354, 0.2149704402110247659, -0.000000000000000000 ) ) ;
#21490=VECTOR ( 'NONE', #27263, 1000.000000000000000 ) ;
#21492=LINE ( 'NONE', #2093, #8247 ) ;
#21498=LINE ( 'NONE', #5458, #3193 ) ;
#21499=CARTESIAN_POINT ( 'NONE',  ( 22.89764159710615132, -1.579009122040562207, -77.50000000000000000 ) ) ;
#21500=VECTOR ( 'NONE', #434, 1000.000000000000000 ) ;
#21506=ADVANCED_FACE ( 'NONE', ( #33129 ), #572, .T. ) ;
#21515=ORIENTED_EDGE ( 'NONE', *, *, #19216, .T. ) ;
#21517=ORIENTED_EDGE ( 'NONE', *, *, #23900, .F. ) ;
#21521=ORIENTED_EDGE ( 'NONE', *, *, #30700, .T. ) ;
#21524=VECTOR ( 'NONE', #29757, 1000.000000000000000 ) ;
#21527=CARTESIAN_POINT ( 'NONE',  ( -41.91891556802573859, 16.36473396058513785, -36.68877005347594178 ) ) ;
#21530=EDGE_CURVE ( 'NONE', #18207, #16944, #26393, .T. ) ;
#21533=CARTESIAN_POINT ( 'NONE',  ( 5.021133111224162171, -23.57973016998034765, -87.50000000000000000 ) ) ;
#21534=VECTOR ( 'NONE', #19708, 1000.000000000000000 ) ;
#21535=EDGE_CURVE ( 'NONE', #24033, #33864, #19629, .T. ) ;
#21538=LINE ( 'NONE', #31840, #15761 ) ;
#21540=DIRECTION ( 'NONE',  ( -0.000000000000000000, 0.5288966977476834419, -0.8486862100397269959 ) ) ;
#21545=CARTESIAN_POINT ( 'NONE',  ( 0.000000000000000000, 3.524919873834583163E-15, 68.31122994652405112 ) ) ;
#21546=CARTESIAN_POINT ( 'NONE',  ( -25.63124651156763179, 20.05601094782695526, -36.68877005347593467 ) ) ;
#21549=LINE ( 'NONE', #19410, #34203 ) ;
#21555=DIRECTION ( 'NONE',  ( 1.000000000000000000, 0.000000000000000000, -0.000000000000000000 ) ) ;
#21556=FACE_OUTER_BOUND ( 'NONE', #34076, .T. ) ;
#21560=DIRECTION ( 'NONE',  ( 0.000000000000000000, 1.000000000000000000, 0.000000000000000000 ) ) ;
#21570=EDGE_CURVE ( 'NONE', #8463, #26131, #15157, .T. ) ;
#21572=DIRECTION ( 'NONE',  ( 0.000000000000000000, 1.836970198721029688E-16, -1.000000000000000000 ) ) ;
#21576=FACE_OUTER_BOUND ( 'NONE', #10138, .T. ) ;
#21577=EDGE_CURVE ( 'NONE', #2206, #31947, #15692, .T. ) ;
#21587=LINE ( 'NONE', #23728, #23174 ) ;
#21593=ORIENTED_EDGE ( 'NONE', *, *, #23673, .F. ) ;
#21594=PLANE ( 'NONE',  #9367 ) ;
#21602=ORIENTED_EDGE ( 'NONE', *, *, #27957, .T. ) ;
#21604=VERTEX_POINT ( 'NONE', #23849 ) ;
#21606=DIRECTION ( 'NONE',  ( 3.697785493223492838E-32, 1.934419779023891545E-16, -1.000000000000000000 ) ) ;
#21612=EDGE_LOOP ( 'NONE', ( #7343, #28315, #7649, #2596 ) ) ;
#21613=VERTEX_POINT ( 'NONE', #20663 ) ;
#21614=DIRECTION ( 'NONE',  ( 0.4198891015602645438, -0.9075754196709570065, -0.000000000000000000 ) ) ;
#21639=CARTESIAN_POINT ( 'NONE',  ( 22.89764159710615132, -5.651112684911597128, -77.50000000000000000 ) ) ;
#21640=CARTESIAN_POINT ( 'NONE',  ( 1.991296462759138297, -32.48444414290483451, 49.43553178847298568 ) ) ;
#21642=EDGE_LOOP ( 'NONE', ( #16630, #31910, #29685, #28349 ) ) ;
#21643=DIRECTION ( 'NONE',  ( 0.000000000000000000, 1.000000000000000000, 0.000000000000000000 ) ) ;
#21649=ORIENTED_EDGE ( 'NONE', *, *, #2532, .F. ) ;
#21651=AXIS2_PLACEMENT_3D ( 'NONE', #29642, #5240, #26974 ) ;
#21652=DIRECTION ( 'NONE',  ( -0.000000000000000000, 1.836970198721029934E-16, -1.000000000000000000 ) ) ;
#21659=DIRECTION ( 'NONE',  ( 0.000000000000000000, 1.836970198721029441E-16, -1.000000000000000000 ) ) ;
#21660=ORIENTED_EDGE ( 'NONE', *, *, #24854, .F. ) ;
#21662=CARTESIAN_POINT ( 'NONE',  ( -32.17792593279633451, -19.96555837188923022, 68.31122994652405112 ) ) ;
#21668=ORIENTED_EDGE ( 'NONE', *, *, #31613, .F. ) ;
#21678=ORIENTED_EDGE ( 'NONE', *, *, #21530, .T. ) ;
#21683=CARTESIAN_POINT ( 'NONE',  ( 22.10765473302597073, -12.47301499840864025, -77.50000000000000000 ) ) ;
#21686=CARTESIAN_POINT ( 'NONE',  ( 32.05156013847311414, -20.15193397489275640, 49.43553178847298568 ) ) ;
#21690=EDGE_CURVE ( 'NONE', #8215, #18536, #28497, .T. ) ;
#21694=DIRECTION ( 'NONE',  ( 0.000000000000000000, 1.000000000000000000, 0.000000000000000000 ) ) ;
#21696=VECTOR ( 'NONE', #9554, 1000.000000000000114 ) ;
#21707=CARTESIAN_POINT ( 'NONE',  ( 10.96230482721425403, -12.47301499840864025, -77.50000000000000000 ) ) ;
#21714=CARTESIAN_POINT ( 'NONE',  ( -35.00000000000000000, -7.062798427011562019, 68.31122994652405112 ) ) ;
#21717=DIRECTION ( 'NONE',  ( -0.000000000000000000, 1.836970198721029688E-16, -1.000000000000000000 ) ) ;
#21723=AXIS2_PLACEMENT_3D ( 'NONE', #31429, #29289, #4886 ) ;
#21731=ORIENTED_EDGE ( 'NONE', *, *, #27033, .F. ) ;
#21742=LINE ( 'NONE', #11420, #7903 ) ;
#21750=AXIS2_PLACEMENT_3D ( 'NONE', #19892, #3669, #28063 ) ;
#21758=ORIENTED_EDGE ( 'NONE', *, *, #1292, .F. ) ;
#21761=DIRECTION ( 'NONE',  ( -1.000000000000000000, 0.000000000000000000, 0.000000000000000000 ) ) ;
#21764=EDGE_CURVE ( 'NONE', #27865, #30543, #34493, .T. ) ;
#21773=ORIENTED_EDGE ( 'NONE', *, *, #20769, .F. ) ;
#21778=DIRECTION ( 'NONE',  ( 0.000000000000000000, 1.000000000000000000, 0.000000000000000000 ) ) ;
#21779=CARTESIAN_POINT ( 'NONE',  ( -5.021133111225196011, -25.61315202898005694, -87.50000000000000000 ) ) ;
#21784=DIRECTION ( 'NONE',  ( 0.000000000000000000, 1.000000000000000000, 0.000000000000000000 ) ) ;
#21787=EDGE_LOOP ( 'NONE', ( #14382, #21119, #2949, #14749 ) ) ;
#21789=VECTOR ( 'NONE', #30864, 1000.000000000000114 ) ;
#21812=ORIENTED_EDGE ( 'NONE', *, *, #23181, .F. ) ;
#21821=DIRECTION ( 'NONE',  ( 0.000000000000000000, -0.8486862100397269959, 0.5288966977476833309 ) ) ;
#21825=CARTESIAN_POINT ( 'NONE',  ( -35.00000000000000000, -46.95407462254104303, -36.69637551990492597 ) ) ;
#21826=CARTESIAN_POINT ( 'NONE',  ( -12.25939112814508825, 30.14816249862102637, 68.31122994652405112 ) ) ;
#21829=CARTESIAN_POINT ( 'NONE',  ( 31.83311414508813897, -6.771795677801495827, 68.31122994652405112 ) ) ;
#21834=LINE ( 'NONE', #2791, #13173 ) ;
#21837=VECTOR ( 'NONE', #6137, 1000.000000000000000 ) ;
#21839=EDGE_LOOP ( 'NONE', ( #24171, #12758, #14387, #23352 ) ) ;
#21848=ORIENTED_EDGE ( 'NONE', *, *, #15400, .F. ) ;
#21851=PLANE ( 'NONE',  #8254 ) ;
#21854=CIRCLE ( 'NONE', #12206, 44.99999999999998579 ) ;
#21855=VERTEX_POINT ( 'NONE', #24896 ) ;
#21856=ORIENTED_EDGE ( 'NONE', *, *, #18407, .T. ) ;
#21858=DIRECTION ( 'NONE',  ( 0.000000000000000000, -0.8486862100397269959, -0.5288966977476834419 ) ) ;
#21860=CARTESIAN_POINT ( 'NONE',  ( -9.978866888775632660, -5.758675521474015291, -67.50000000000000000 ) ) ;
#21873=DIRECTION ( 'NONE',  ( 3.697785493223492838E-32, 1.934419779023891545E-16, -1.000000000000000000 ) ) ;
#21875=VERTEX_POINT ( 'NONE', #27578 ) ;
#21878=CYLINDRICAL_SURFACE ( 'NONE', #410, 2.033421858999711951 ) ;
#21879=ORIENTED_EDGE ( 'NONE', *, *, #6070, .F. ) ;
#21886=EDGE_CURVE ( 'NONE', #28031, #28204, #28108, .T. ) ;
#21887=CARTESIAN_POINT ( 'NONE',  ( 6.078604839177344843, 33.69708579775584667, 68.31122994652405112 ) ) ;
#21897=CARTESIAN_POINT ( 'NONE',  ( -14.84098889165990620, 28.96462362251114087, 68.31122994652405112 ) ) ;
#21902=EDGE_CURVE ( 'NONE', #9877, #3883, #16923, .T. ) ;
#21908=ORIENTED_EDGE ( 'NONE', *, *, #6665, .T. ) ;
#21911=ADVANCED_FACE ( 'NONE', ( #25430 ), #360, .F. ) ;
#21916=CARTESIAN_POINT ( 'NONE',  ( 21.85761591200894216, 30.91355005303805825, 68.31122994652405112 ) ) ;
#21918=VECTOR ( 'NONE', #18002, 1000.000000000000000 ) ;
#21927=FACE_OUTER_BOUND ( 'NONE', #19888, .T. ) ;
#21931=LINE ( 'NONE', #10901, #29909 ) ;
#21943=DIRECTION ( 'NONE',  ( -0.000000000000000000, -0.000000000000000000, 1.000000000000000000 ) ) ;
#21948=EDGE_LOOP ( 'NONE', ( #23934, #29666, #12450, #3906 ) ) ;
#21951=CARTESIAN_POINT ( 'NONE',  ( 25.76952721012208514, 19.87802405277947315, 68.31122994652405112 ) ) ;
#21971=CYLINDRICAL_SURFACE ( 'NONE', #8013, 32.54542015209057126 ) ;
#21973=EDGE_CURVE ( 'NONE', #15156, #6016, #32297, .T. ) ;
#21978=VECTOR ( 'NONE', #30520, 1000.000000000000000 ) ;
#21979=LINE ( 'NONE', #2920, #14610 ) ;
#21994=DIRECTION ( 'NONE',  ( -1.000000000000000000, 0.000000000000000000, -0.000000000000000000 ) ) ;
#21996=CARTESIAN_POINT ( 'NONE',  ( 0.000000000000000000, -33.69708579775584667, 49.43553178847298568 ) ) ;
#22002=VERTEX_POINT ( 'NONE', #4053 ) ;
#22003=EDGE_LOOP ( 'NONE', ( #30666, #33991, #25586, #31359 ) ) ;
#22007=LINE ( 'NONE', #27862, #33362 ) ;
#22010=VERTEX_POINT ( 'NONE', #7919 ) ;
#22017=CARTESIAN_POINT ( 'NONE',  ( -30.91434716440808472, 10.17386417614055105, -36.68877005347593467 ) ) ;
#22018=LINE ( 'NONE', #30376, #25418 ) ;
#22022=EDGE_CURVE ( 'NONE', #8902, #18426, #23772, .T. ) ;
#22026=AXIS2_PLACEMENT_3D ( 'NONE', #2614, #13482, #32505 ) ;
#22027=AXIS2_PLACEMENT_3D ( 'NONE', #14989, #17501, #1275 ) ;
#22028=ADVANCED_FACE ( 'NONE', ( #21096 ), #26785, .F. ) ;
#22029=CARTESIAN_POINT ( 'NONE',  ( -20.02113311122488781, 8.235406450278427215, -67.50000000000000000 ) ) ;
#22030=EDGE_LOOP ( 'NONE', ( #8607, #2576, #27155, #7036 ) ) ;
#22036=CARTESIAN_POINT ( 'NONE',  ( -32.54223829851967764, 0.4550817492056293823, -36.68877005347593467 ) ) ;
#22041=FACE_OUTER_BOUND ( 'NONE', #27864, .T. ) ;
#22043=EDGE_LOOP ( 'NONE', ( #11978, #32395, #6532, #3587 ) ) ;
#22044=DIRECTION ( 'NONE',  ( -0.1081190184239421148, 0.9941379571543595972, -0.000000000000000000 ) ) ;
#22051=ORIENTED_EDGE ( 'NONE', *, *, #6576, .F. ) ;
#22052=VERTEX_POINT ( 'NONE', #268 ) ;
#22054=DIRECTION ( 'NONE',  ( 0.5155538571770196254, 0.8568571761675904952, 1.574021097180118762E-16 ) ) ;
#22055=EDGE_CURVE ( 'NONE', #20418, #26158, #24626, .T. ) ;
#22056=LINE ( 'NONE', #32899, #27374 ) ;
#22062=VERTEX_POINT ( 'NONE', #10946 ) ;
#22066=DIRECTION ( 'NONE',  ( 0.000000000000000000, 1.000000000000000000, 0.000000000000000000 ) ) ;
#22067=VERTEX_POINT ( 'NONE', #13796 ) ;
#22073=CARTESIAN_POINT ( 'NONE',  ( -9.978866888775632660, -5.758675521474015291, -67.50000000000000000 ) ) ;
#22074=DIRECTION ( 'NONE',  ( 0.000000000000000000, 1.836970198721029934E-16, -1.000000000000000000 ) ) ;
#22077=AXIS2_PLACEMENT_3D ( 'NONE', #31659, #33992, #28996 ) ;
#22083=DIRECTION ( 'NONE',  ( -0.9868265225415260300, 0.1617819965527647341, 0.000000000000000000 ) ) ;
#22085=EDGE_LOOP ( 'NONE', ( #25671, #32158, #17863, #7355 ) ) ;
#22087=AXIS2_PLACEMENT_3D ( 'NONE', #18877, #32906, #29549 ) ;
#22095=ADVANCED_FACE ( 'NONE', ( #19319 ), #2749, .T. ) ;
#22102=ORIENTED_EDGE ( 'NONE', *, *, #11395, .F. ) ;
#22106=DIRECTION ( 'NONE',  ( 1.000000000000000000, 0.000000000000000000, 0.000000000000000000 ) ) ;
#22121=VECTOR ( 'NONE', #23080, 1000.000000000000000 ) ;
#22131=CARTESIAN_POINT ( 'NONE',  ( -5.021133111225092982, -15.68591377522703390, -87.50000000000000000 ) ) ;
#22134=LINE ( 'NONE', #425, #14493 ) ;
#22135=EDGE_CURVE ( 'NONE', #24766, #2999, #616, .T. ) ;
#22139=CARTESIAN_POINT ( 'NONE',  ( -34.66645501699844090, -15.21971901163153440, -36.68877005347593467 ) ) ;
#22141=ORIENTED_EDGE ( 'NONE', *, *, #5632, .T. ) ;
#22149=EDGE_LOOP ( 'NONE', ( #31501, #11949, #33285, #3915 ) ) ;
#22153=CARTESIAN_POINT ( 'NONE',  ( 3.235562306570555532E-30, -5.758675521474011738, -87.50000000000000000 ) ) ;
#22155=DIRECTION ( 'NONE',  ( 0.000000000000000000, 1.836970198721029441E-16, -1.000000000000000000 ) ) ;
#22161=DIRECTION ( 'NONE',  ( 0.000000000000000000, 1.000000000000000000, 0.000000000000000000 ) ) ;
#22178=DIRECTION ( 'NONE',  ( 1.000000000000000000, 0.000000000000000000, 0.000000000000000000 ) ) ;
#22186=DIRECTION ( 'NONE',  ( -0.6051742151937647973, -0.7960930657056438653, -0.000000000000000000 ) ) ;
#22187=FACE_OUTER_BOUND ( 'NONE', #29715, .T. ) ;
#22188=DIRECTION ( 'NONE',  ( 0.2149704402110223789, -0.9766205557100871015, -1.794022856297801510E-16 ) ) ;
#22210=ORIENTED_EDGE ( 'NONE', *, *, #18415, .T. ) ;
#22211=EDGE_CURVE ( 'NONE', #13343, #1565, #14694, .T. ) ;
#22212=EDGE_CURVE ( 'NONE', #29973, #21178, #25341, .T. ) ;
#22214=VECTOR ( 'NONE', #17423, 1000.000000000000000 ) ;
#22217=FACE_OUTER_BOUND ( 'NONE', #25159, .T. ) ;
#22220=ADVANCED_FACE ( 'NONE', ( #28551 ), #15034, .F. ) ;
#22229=LINE ( 'NONE', #8694, #27941 ) ;
#22234=ORIENTED_EDGE ( 'NONE', *, *, #24689, .F. ) ;
#22243=VECTOR ( 'NONE', #32226, 1000.000000000000000 ) ;
#22246=ORIENTED_EDGE ( 'NONE', *, *, #121, .T. ) ;
#22255=CARTESIAN_POINT ( 'NONE',  ( 21.24400529595485310, -24.65555945140048522, 68.31122994652405112 ) ) ;
#22256=CIRCLE ( 'NONE', #663, 32.54542015209054284 ) ;
#22257=EDGE_CURVE ( 'NONE', #29402, #28782, #30695, .T. ) ;
#22258=EDGE_CURVE ( 'NONE', #20922, #3555, #12366, .T. ) ;
#22259=VERTEX_POINT ( 'NONE', #20203 ) ;
#22261=ORIENTED_EDGE ( 'NONE', *, *, #16948, .T. ) ;
#22278=LINE ( 'NONE', #19623, #32343 ) ;
#22284=DIRECTION ( 'NONE',  ( 0.000000000000000000, 0.000000000000000000, 1.000000000000000000 ) ) ;
#22290=LINE ( 'NONE', #19635, #749 ) ;
#22298=FACE_OUTER_BOUND ( 'NONE', #28180, .T. ) ;
#22301=EDGE_CURVE ( 'NONE', #32774, #7713, #14340, .T. ) ;
#22302=ADVANCED_FACE ( 'NONE', ( #25162 ), #17372, .T. ) ;
#22304=EDGE_CURVE ( 'NONE', #33409, #7560, #791, .T. ) ;
#22305=ORIENTED_EDGE ( 'NONE', *, *, #16461, .F. ) ;
#22309=VERTEX_POINT ( 'NONE', #9147 ) ;
#22315=DIRECTION ( 'NONE',  ( 3.697785493223492838E-32, 1.934419779023891545E-16, -1.000000000000000000 ) ) ;
#22319=LINE ( 'NONE', #960, #29905 ) ;
#22321=CARTESIAN_POINT ( 'NONE',  ( 10.17231796313407344, -5.651112684911598016, -77.50000000000000000 ) ) ;
#22327=ORIENTED_EDGE ( 'NONE', *, *, #14607, .T. ) ;
#22328=PLANE ( 'NONE',  #32761 ) ;
#22332=FACE_OUTER_BOUND ( 'NONE', #25323, .T. ) ;
#22339=VERTEX_POINT ( 'NONE', #28198 ) ;
#22343=DIRECTION ( 'NONE',  ( -0.6876994588534230957, -0.7259954919231310644, 0.000000000000000000 ) ) ;
#22344=ADVANCED_FACE ( 'NONE', ( #33709 ), #6469, .T. ) ;
#22345=ADVANCED_FACE ( 'NONE', ( #22695 ), #6646, .F. ) ;
#22348=EDGE_CURVE ( 'NONE', #12803, #23775, #17278, .T. ) ;
#22355=CARTESIAN_POINT ( 'NONE',  ( 8.927936315454028104, -31.29690601358700519, 49.43553178847298568 ) ) ;
#22366=DIRECTION ( 'NONE',  ( -0.000000000000000000, -0.000000000000000000, -1.000000000000000000 ) ) ;
#22369=AXIS2_PLACEMENT_3D ( 'NONE', #18021, #23334, #12323 ) ;
#22384=DIRECTION ( 'NONE',  ( 1.000000000000000000, 0.000000000000000000, 0.000000000000000000 ) ) ;
#22395=ORIENTED_EDGE ( 'NONE', *, *, #31333, .F. ) ;
#22401=ORIENTED_EDGE ( 'NONE', *, *, #8282, .F. ) ;
#22403=DIRECTION ( 'NONE',  ( 0.000000000000000000, 1.836970198721029441E-16, -1.000000000000000000 ) ) ;
#22408=DIRECTION ( 'NONE',  ( -0.3193015301359803382, -0.9476531711828023452, 0.000000000000000000 ) ) ;
#22413=EDGE_CURVE ( 'NONE', #11793, #20827, #7335, .T. ) ;
#22416=ORIENTED_EDGE ( 'NONE', *, *, #27963, .T. ) ;
#22422=VECTOR ( 'NONE', #14659, 1000.000000000000000 ) ;
#22423=DIRECTION ( 'NONE',  ( -0.000000000000000000, -1.000000000000000000, -0.000000000000000000 ) ) ;
#22429=LINE ( 'NONE', #19937, #30907 ) ;
#22448=ORIENTED_EDGE ( 'NONE', *, *, #11309, .F. ) ;
#22459=ORIENTED_EDGE ( 'NONE', *, *, #16696, .F. ) ;
#22464=AXIS2_PLACEMENT_3D ( 'NONE', #8384, #24395, #27777 ) ;
#22465=DIRECTION ( 'NONE',  ( 0.000000000000000000, 1.000000000000000000, 1.836970198721029688E-16 ) ) ;
#22478=ORIENTED_EDGE ( 'NONE', *, *, #32337, .T. ) ;
#22485=VECTOR ( 'NONE', #13476, 1000.000000000000000 ) ;
#22486=ORIENTED_EDGE ( 'NONE', *, *, #2636, .T. ) ;
#22497=VERTEX_POINT ( 'NONE', #26916 ) ;
#22500=VECTOR ( 'NONE', #25478, 1000.000000000000000 ) ;
#22503=CARTESIAN_POINT ( 'NONE',  ( 24.90835164106607635, -28.52396285516520891, 49.43553178847298568 ) ) ;
#22514=DIRECTION ( 'NONE',  ( -0.1081190184239417262, -0.9941379571543595972, 0.000000000000000000 ) ) ;
#22516=DIRECTION ( 'NONE',  ( 0.4684084406997896521, 0.8835120444460232703, 1.622985295858434769E-16 ) ) ;
#22517=AXIS2_PLACEMENT_3D ( 'NONE', #25505, #28876, #15190 ) ;
#22527=DIRECTION ( 'NONE',  ( 0.000000000000000000, -0.000000000000000000, -1.000000000000000000 ) ) ;
#22536=CARTESIAN_POINT ( 'NONE',  ( 32.40067729534749219, 3.066020821660475626, 49.43553178847298568 ) ) ;
#22540=LINE ( 'NONE', #11689, #14826 ) ;
#22546=DIRECTION ( 'NONE',  ( 0.8835120444460229372, 0.4684084406997900407, 0.000000000000000000 ) ) ;
#22553=DIRECTION ( 'NONE',  ( 0.000000000000000000, 0.000000000000000000, 1.000000000000000000 ) ) ;
#22562=VERTEX_POINT ( 'NONE', #1276 ) ;
#22571=CARTESIAN_POINT ( 'NONE',  ( -31.87924797510909869, -6.551177101682105430, -36.68877005347593467 ) ) ;
#22573=EDGE_LOOP ( 'NONE', ( #27315, #18050, #24329, #32987 ) ) ;
#22575=DIRECTION ( 'NONE',  ( -0.000000000000000000, 1.836970198721029934E-16, -1.000000000000000000 ) ) ;
#22576=VERTEX_POINT ( 'NONE', #27795 ) ;
#22580=CARTESIAN_POINT ( 'NONE',  ( -35.00000000000000000, 3.432458613951602011, 68.31122994652405112 ) ) ;
#22582=ORIENTED_EDGE ( 'NONE', *, *, #19546, .F. ) ;
#22587=AXIS2_PLACEMENT_3D ( 'NONE', #1316, #26206, #20875 ) ;
#22592=ORIENTED_EDGE ( 'NONE', *, *, #31930, .T. ) ;
#22594=VERTEX_POINT ( 'NONE', #22991 ) ;
#22608=FACE_OUTER_BOUND ( 'NONE', #23366, .T. ) ;
#22613=PLANE ( 'NONE',  #6527 ) ;
#22616=ADVANCED_FACE ( 'NONE', ( #6777 ), #19807, .T. ) ;
#22618=VECTOR ( 'NONE', #1237, 1000.000000000000000 ) ;
#22624=DIRECTION ( 'NONE',  ( -1.000000000000000000, -0.000000000000000000, -0.000000000000000000 ) ) ;
#22625=EDGE_CURVE ( 'NONE', #9821, #1704, #6602, .T. ) ;
#22626=EDGE_CURVE ( 'NONE', #7363, #22339, #20325, .T. ) ;
#22632=CARTESIAN_POINT ( 'NONE',  ( 17.27856612038527118, 33.69708579775584667, 49.43553178847298568 ) ) ;
#22637=LINE ( 'NONE', #1440, #14717 ) ;
#22641=VECTOR ( 'NONE', #1444, 1000.000000000000114 ) ;
#22645=ADVANCED_FACE ( 'NONE', ( #17142 ), #31001, .T. ) ;
#22650=CARTESIAN_POINT ( 'NONE',  ( 0.000000000000000000, -33.69708579775584667, 49.43553178847298568 ) ) ;
#22651=ADVANCED_FACE ( 'NONE', ( #6069 ), #14291, .F. ) ;
#22652=PLANE ( 'NONE',  #16132 ) ;
#22655=CARTESIAN_POINT ( 'NONE',  ( 32.30227131129396412, -3.970848902647437395, 68.31122994652405112 ) ) ;
#22658=ORIENTED_EDGE ( 'NONE', *, *, #19424, .F. ) ;
#22662=ORIENTED_EDGE ( 'NONE', *, *, #21530, .F. ) ;
#22668=ORIENTED_EDGE ( 'NONE', *, *, #11761, .F. ) ;
#22671=VERTEX_POINT ( 'NONE', #26525 ) ;
#22677=VERTEX_POINT ( 'NONE', #15506 ) ;
#22679=CARTESIAN_POINT ( 'NONE',  ( -32.37866696771086339, 3.290334066652079947, 68.31122994652405112 ) ) ;
#22682=CARTESIAN_POINT ( 'NONE',  ( 5.021133111224679091, 28.08988295778447508, -67.50000000000000000 ) ) ;
#22684=LINE ( 'NONE', #19484, #21500 ) ;
#22688=ORIENTED_EDGE ( 'NONE', *, *, #34026, .F. ) ;
#22689=DIRECTION ( 'NONE',  ( 0.000000000000000000, -1.000000000000000000, -3.083952846180992253E-16 ) ) ;
#22695=FACE_OUTER_BOUND ( 'NONE', #16420, .T. ) ;
#22707=EDGE_CURVE ( 'NONE', #28991, #20852, #3483, .T. ) ;
#22730=FACE_OUTER_BOUND ( 'NONE', #21397, .T. ) ;
#22740=ORIENTED_EDGE ( 'NONE', *, *, #15107, .F. ) ;
#22742=LINE ( 'NONE', #3335, #2008 ) ;
#22743=CARTESIAN_POINT ( 'NONE',  ( 3.235562306570555532E-30, 18.16264470403145026, -67.50000000000000000 ) ) ;
#22752=VERTEX_POINT ( 'NONE', #34186 ) ;
#22753=CARTESIAN_POINT ( 'NONE',  ( -5.021133111224989953, -5.758675521474015291, -67.50000000000000000 ) ) ;
#22757=ORIENTED_EDGE ( 'NONE', *, *, #7099, .T. ) ;
#22758=ORIENTED_EDGE ( 'NONE', *, *, #23338, .F. ) ;
#22760=EDGE_CURVE ( 'NONE', #22002, #17949, #31515, .T. ) ;
#22764=ORIENTED_EDGE ( 'NONE', *, *, #634, .T. ) ;
#22766=CARTESIAN_POINT ( 'NONE',  ( 37.09133285470120711, -7.633836879289870758, 49.43553178847298568 ) ) ;
#22768=CARTESIAN_POINT ( 'NONE',  ( 3.235562306570555532E-30, 4.168562732279007754, -87.50000000000000000 ) ) ;
#22775=ORIENTED_EDGE ( 'NONE', *, *, #34767, .F. ) ;
#22778=DIRECTION ( 'NONE',  ( 0.000000000000000000, 1.836970198721029441E-16, -1.000000000000000000 ) ) ;
#22790=VECTOR ( 'NONE', #15942, 1000.000000000000000 ) ;
#22796=CARTESIAN_POINT ( 'NONE',  ( -23.46927268871044348, -22.54767421130285143, 68.31122994652405112 ) ) ;
#22806=AXIS2_PLACEMENT_3D ( 'NONE', #1156, #8804, #14346 ) ;
#22811=LINE ( 'NONE', #28331, #30510 ) ;
#22826=ORIENTED_EDGE ( 'NONE', *, *, #24897, .F. ) ;
#22834=EDGE_CURVE ( 'NONE', #15568, #16675, #21549, .T. ) ;
#22840=AXIS2_PLACEMENT_3D ( 'NONE', #25325, #14677, #25502 ) ;
#22856=DIRECTION ( 'NONE',  ( 0.000000000000000000, -0.5288966977476834419, -0.8486862100397269959 ) ) ;
#22860=VECTOR ( 'NONE', #25255, 1000.000000000000114 ) ;
#22861=CARTESIAN_POINT ( 'NONE',  ( 5.021133111224369117, -1.691831803474591833, -67.50000000000000000 ) ) ;
#22863=ADVANCED_FACE ( 'NONE', ( #2841 ), #27056, .T. ) ;
#22865=EDGE_CURVE ( 'NONE', #8883, #9321, #2670, .T. ) ;
#22869=EDGE_CURVE ( 'NONE', #12655, #2863, #24377, .T. ) ;
#22877=PRODUCT ( 'motor', 'motor', '', ( #552 ) ) ;
#22879=VERTEX_POINT ( 'NONE', #30250 ) ;
#22880=VECTOR ( 'NONE', #26699, 1000.000000000000114 ) ;
#22881=EDGE_CURVE ( 'NONE', #6216, #23009, #19240, .T. ) ;
#22885=EDGE_LOOP ( 'NONE', ( #12746, #18113, #8344, #1660, #62, #27691, #6631, #18899, #17183, #25850, #3420, #3851, #25677, #2664, #25896, #1270, #19837, #7962, #25796, #22327, #27111, #27184, #10393, #18918, #23531, #24556, #31268, #3203, #2892, #19363, #6042, #2516, #1987, #13806, #9097, #12762, #15835, #21275, #10805, #15300, #28993, #1343, #6670, #33567, #17573, #834, #15938, #869, #16993, #23135, #14710, #14884, #7223, #21226, #6302, #19085, #8383, #6374, #7795, #298, #33971, #9105 ) ) ;
#22886=EDGE_LOOP ( 'NONE', ( #26676, #15861, #32580, #18485 ) ) ;
#22890=DIRECTION ( 'NONE',  ( 0.05413890858541786644, -0.9985334138511238189, 0.000000000000000000 ) ) ;
#22892=VERTEX_POINT ( 'NONE', #27404 ) ;
#22894=CARTESIAN_POINT ( 'NONE',  ( 0.000000000000000000, 2.281310696040539424E-14, -36.68877005347592757 ) ) ;
#22900=ORIENTED_EDGE ( 'NONE', *, *, #32929, .F. ) ;
#22906=ORIENTED_EDGE ( 'NONE', *, *, #1684, .T. ) ;
#22908=AXIS2_PLACEMENT_3D ( 'NONE', #3011, #27226, #33089 ) ;
#22910=DIRECTION ( 'NONE',  ( 0.4684084406997904848, -0.8835120444460226041, 0.000000000000000000 ) ) ;
#22911=VERTEX_POINT ( 'NONE', #33274 ) ;
#22916=FACE_OUTER_BOUND ( 'NONE', #24290, .T. ) ;
#22921=CYLINDRICAL_SURFACE ( 'NONE', #9093, 2.033421858999711951 ) ;
#22928=DIRECTION ( 'NONE',  ( 3.697785493223492838E-32, 1.934419779023891545E-16, -1.000000000000000000 ) ) ;
#22932=ORIENTED_EDGE ( 'NONE', *, *, #415, .F. ) ;
#22933=CARTESIAN_POINT ( 'NONE',  ( -20.02113311122509032, -13.65249191622732816, -67.50000000000000000 ) ) ;
#22934=CARTESIAN_POINT ( 'NONE',  ( -9.144464960067645976, -31.23432620483747968, 68.31122994652405112 ) ) ;
#22938=CARTESIAN_POINT ( 'NONE',  ( -37.12776225901827587, -7.411627343331139706, -36.68877005347593467 ) ) ;
#22939=ORIENTED_EDGE ( 'NONE', *, *, #31983, .T. ) ;
#22958=VECTOR ( 'NONE', #17669, 1000.000000000000000 ) ;
#22969=VERTEX_POINT ( 'NONE', #539 ) ;
#22973=LINE ( 'NONE', #28486, #15614 ) ;
#22980=EDGE_CURVE ( 'NONE', #20852, #28991, #29660, .T. ) ;
#22981=VECTOR ( 'NONE', #19042, 1000.000000000000000 ) ;
#22982=EDGE_CURVE ( 'NONE', #27216, #18999, #3723, .T. ) ;
#22987=LINE ( 'NONE', #10112, #18897 ) ;
#22991=CARTESIAN_POINT ( 'NONE',  ( -9.978866888775632660, -1.691831803474591833, -67.50000000000000000 ) ) ;
#22992=LINE ( 'NONE', #17323, #33152 ) ;
#22994=DIRECTION ( 'NONE',  ( -0.6876994588534237618, -0.7259954919231303982, 0.000000000000000000 ) ) ;
#22996=EDGE_CURVE ( 'NONE', #21875, #33864, #11575, .T. ) ;
#22999=ORIENTED_EDGE ( 'NONE', *, *, #17256, .T. ) ;
#23004=ADVANCED_FACE ( 'NONE', ( #22608 ), #9071, .F. ) ;
#23009=VERTEX_POINT ( 'NONE', #17465 ) ;
#23015=ORIENTED_EDGE ( 'NONE', *, *, #17654, .T. ) ;
#23017=DIRECTION ( 'NONE',  ( 0.000000000000000000, -1.836970198721029688E-16, 1.000000000000000000 ) ) ;
#23022=CARTESIAN_POINT ( 'NONE',  ( 5.021133111224162171, -25.61315202898006049, -67.50000000000000000 ) ) ;
#23029=DIRECTION ( 'NONE',  ( 0.000000000000000000, 1.836970198721029934E-16, -1.000000000000000000 ) ) ;
#23031=ORIENTED_EDGE ( 'NONE', *, *, #494, .T. ) ;
#23042=DIRECTION ( 'NONE',  ( -0.000000000000000000, 1.836970198721029688E-16, -1.000000000000000000 ) ) ;
#23055=VECTOR ( 'NONE', #27485, 1000.000000000000000 ) ;
#23056=PLANE ( 'NONE',  #33051 ) ;
#23058=VERTEX_POINT ( 'NONE', #17982 ) ;
#23059=ADVANCED_FACE ( 'NONE', ( #4409 ), #31476, .T. ) ;
#23063=CARTESIAN_POINT ( 'NONE',  ( 3.235562306570555532E-30, 1.325223266901699007E-14, -67.50000000000000000 ) ) ;
#23066=DIRECTION ( 'NONE',  ( -0.000000000000000000, 1.836970198721029688E-16, -1.000000000000000000 ) ) ;
#23068=ADVANCED_FACE ( 'NONE', ( #28984 ), #15126, .F. ) ;
#23069=CARTESIAN_POINT ( 'NONE',  ( -5.021133111225092982, -13.65249191622732816, -67.50000000000000000 ) ) ;
#23075=ORIENTED_EDGE ( 'NONE', *, *, #12545, .T. ) ;
#23076=DIRECTION ( 'NONE',  ( -1.000000000000000000, 6.792721752314501023E-48, -3.697785493223492838E-32 ) ) ;
#23079=EDGE_CURVE ( 'NONE', #18985, #10479, #34680, .T. ) ;
#23080=DIRECTION ( 'NONE',  ( 0.000000000000000000, 1.836970198721029441E-16, -1.000000000000000000 ) ) ;
#23086=AXIS2_PLACEMENT_3D ( 'NONE', #34229, #31890, #7873 ) ;
#23087=CARTESIAN_POINT ( 'NONE',  ( 31.73435513276359643, 7.220462394039750542, 68.31122994652405112 ) ) ;
#23101=CARTESIAN_POINT ( 'NONE',  ( -35.00000000000000000, -4.184937238521367675, -15.81122994652403513 ) ) ;
#23102=VERTEX_POINT ( 'NONE', #20801 ) ;
#23109=EDGE_CURVE ( 'NONE', #13030, #640, #29159, .T. ) ;
#23118=VERTEX_POINT ( 'NONE', #23136 ) ;
#23124=PLANE ( 'NONE',  #19939 ) ;
#23135=ORIENTED_EDGE ( 'NONE', *, *, #29781, .F. ) ;
#23136=CARTESIAN_POINT ( 'NONE',  ( -35.00000000000000000, 16.36947364650383818, 36.69637551990492597 ) ) ;
#23140=DIRECTION ( 'NONE',  ( 0.8568571761675890519, -0.5155538571770220679, -9.470570714698675251E-17 ) ) ;
#23155=ORIENTED_EDGE ( 'NONE', *, *, #6154, .F. ) ;
#23156=LINE ( 'NONE', #19784, #34391 ) ;
#23157=DIRECTION ( 'NONE',  ( 0.000000000000000000, 0.000000000000000000, 1.000000000000000000 ) ) ;
#23159=DIRECTION ( 'NONE',  ( 1.000000000000000000, 0.000000000000000000, 0.000000000000000000 ) ) ;
#23161=VERTEX_POINT ( 'NONE', #10993 ) ;
#23162=LINE ( 'NONE', #33478, #27657 ) ;
#23164=LINE ( 'NONE', #6413, #19988 ) ;
#23170=DIRECTION ( 'NONE',  ( -0.8835120444460224931, -0.4684084406997908179, 0.000000000000000000 ) ) ;
#23173=AXIS2_PLACEMENT_3D ( 'NONE', #18753, #2525, #36 ) ;
#23174=VECTOR ( 'NONE', #26566, 1000.000000000000000 ) ;
#23181=EDGE_CURVE ( 'NONE', #6717, #24229, #26662, .T. ) ;
#23186=AXIS2_PLACEMENT_3D ( 'NONE', #12176, #9313, #25324 ) ;
#23187=PLANE ( 'NONE',  #27840 ) ;
#23188=ORIENTED_EDGE ( 'NONE', *, *, #1881, .F. ) ;
#23189=ORIENTED_EDGE ( 'NONE', *, *, #13235, .T. ) ;
#23198=ORIENTED_EDGE ( 'NONE', *, *, #10444, .F. ) ;
#23201=CARTESIAN_POINT ( 'NONE',  ( 0.000000000000000000, 2.296212748401288367E-15, 87.50000000000000000 ) ) ;
#23204=DIRECTION ( 'NONE',  ( -0.000000000000000000, 1.836970198721029934E-16, -1.000000000000000000 ) ) ;
#23213=PLANE ( 'NONE',  #33077 ) ;
#23235=EDGE_CURVE ( 'NONE', #10833, #6717, #33577, .T. ) ;
#23238=VECTOR ( 'NONE', #14772, 1000.000000000000000 ) ;
#23240=FACE_OUTER_BOUND ( 'NONE', #25765, .T. ) ;
#23244=EDGE_CURVE ( 'NONE', #3078, #12010, #6163, .T. ) ;
#23246=FACE_OUTER_BOUND ( 'NONE', #4506, .T. ) ;
#23255=ORIENTED_EDGE ( 'NONE', *, *, #29181, .T. ) ;
#23258=EDGE_CURVE ( 'NONE', #10055, #32960, #27713, .T. ) ;
#23262=CARTESIAN_POINT ( 'NONE',  ( 34.14795412574902400, 16.36947364650384529, 49.43553178847298568 ) ) ;
#23272=ORIENTED_EDGE ( 'NONE', *, *, #5419, .F. ) ;
#23281=PLANE ( 'NONE',  #24254 ) ;
#23285=EDGE_CURVE ( 'NONE', #7553, #23884, #6522, .T. ) ;
#23287=VERTEX_POINT ( 'NONE', #19898 ) ;
#23292=DIRECTION ( 'NONE',  ( -0.5611870653623824978, 0.8276889981568904542, 1.520440023423473517E-16 ) ) ;
#23295=ORIENTED_EDGE ( 'NONE', *, *, #21577, .T. ) ;
#23298=EDGE_LOOP ( 'NONE', ( #23871, #10849, #8454, #13873, #28521, #19960, #15502, #30291 ) ) ;
#23301=DIRECTION ( 'NONE',  ( -0.000000000000000000, 0.8486862100397269959, 0.5288966977476834419 ) ) ;
#23304=VECTOR ( 'NONE', #24300, 1000.000000000000114 ) ;
#23310=ORIENTED_EDGE ( 'NONE', *, *, #442, .F. ) ;
#23311=EDGE_LOOP ( 'NONE', ( #19573, #19202, #13993, #11864 ) ) ;
#23322=LINE ( 'NONE', #34168, #29242 ) ;
#23328=CARTESIAN_POINT ( 'NONE',  ( 22.89764159710613001, 6.310691531022070144, -77.50000000000000000 ) ) ;
#23330=CARTESIAN_POINT ( 'NONE',  ( 3.235562306570555532E-30, 24.02303923978505296, -87.50000000000000000 ) ) ;
#23333=CARTESIAN_POINT ( 'NONE',  ( -11.83261234297099662, -30.31820670846267873, 68.31122994652405112 ) ) ;
#23334=DIRECTION ( 'NONE',  ( -0.3701381553399144542, 0.9289767198167914186, 1.706502549609061988E-16 ) ) ;
#23338=EDGE_CURVE ( 'NONE', #20533, #32765, #20763, .T. ) ;
#23341=CARTESIAN_POINT ( 'NONE',  ( -20.02113311122509032, -15.68591377522703745, -67.50000000000000000 ) ) ;
#23346=EDGE_LOOP ( 'NONE', ( #29259, #19564, #9794, #12682, #31800, #34816, #17276, #30791, #24563, #8803, #177, #2284 ) ) ;
#23349=EDGE_LOOP ( 'NONE', ( #28362, #26890, #27399, #20007 ) ) ;
#23352=ORIENTED_EDGE ( 'NONE', *, *, #16948, .F. ) ;
#23356=PLANE ( 'NONE',  #29462 ) ;
#23366=EDGE_LOOP ( 'NONE', ( #22757, #17903, #8242, #1291 ) ) ;
#23370=CARTESIAN_POINT ( 'NONE',  ( -9.978866888775632660, -3.725253662474300231, -87.50000000000000000 ) ) ;
#23372=CARTESIAN_POINT ( 'NONE',  ( -2.791255079241054649, -37.75727539589166071, 68.31122994652405112 ) ) ;
#23382=VECTOR ( 'NONE', #8628, 1000.000000000000000 ) ;
#23392=ORIENTED_EDGE ( 'NONE', *, *, #30950, .T. ) ;
#23407=CARTESIAN_POINT ( 'NONE',  ( -25.07182831876307105, -28.36910952062232738, -36.68877005347593467 ) ) ;
#23411=DIRECTION ( 'NONE',  ( -0.8276889981568904542, 0.5611870653623824978, 0.000000000000000000 ) ) ;
#23415=DIRECTION ( 'NONE',  ( 0.000000000000000000, 1.836970198721029688E-16, -1.000000000000000000 ) ) ;
#23422=ORIENTED_EDGE ( 'NONE', *, *, #32394, .T. ) ;
#23434=CARTESIAN_POINT ( 'NONE',  ( -35.00000000000000000, -46.95407462254104303, 36.69637551990492597 ) ) ;
#23435=EDGE_CURVE ( 'NONE', #14210, #22879, #24114, .T. ) ;
#23444=CARTESIAN_POINT ( 'NONE',  ( -29.34345171400087793, 14.07715221144534823, 68.31122994652405112 ) ) ;
#23445=ORIENTED_EDGE ( 'NONE', *, *, #11998, .T. ) ;
#23449=CARTESIAN_POINT ( 'NONE',  ( 24.11848021413634768, 29.19488569250030352, 49.43553178847298568 ) ) ;
#23450=DIRECTION ( 'NONE',  ( 0.000000000000000000, 0.000000000000000000, 1.000000000000000000 ) ) ;
#23452=DIRECTION ( 'NONE',  ( 0.000000000000000000, 1.836970198721029688E-16, -1.000000000000000000 ) ) ;
#23453=AXIS2_PLACEMENT_3D ( 'NONE', #7172, #1504, #31057 ) ;
#23460=EDGE_LOOP ( 'NONE', ( #30743, #19045, #23198, #7766 ) ) ;
#23461=CARTESIAN_POINT ( 'NONE',  ( 24.90835164106607280, -28.52396285516520891, 68.31122994652405112 ) ) ;
#23468=DIRECTION ( 'NONE',  ( 0.000000000000000000, -1.000000000000000000, -2.132064625830773463E-16 ) ) ;
#23469=DIRECTION ( 'NONE',  ( 0.000000000000000000, 1.000000000000000000, 0.000000000000000000 ) ) ;
#23472=ORIENTED_EDGE ( 'NONE', *, *, #7099, .F. ) ;
#23473=AXIS2_PLACEMENT_3D ( 'NONE', #28065, #6695, #22910 ) ;
#23477=ORIENTED_EDGE ( 'NONE', *, *, #24691, .F. ) ;
#23478=EDGE_CURVE ( 'NONE', #21604, #16288, #8098, .T. ) ;
#23486=EDGE_CURVE ( 'NONE', #2835, #18207, #29477, .T. ) ;
#23495=PLANE ( 'NONE',  #2814 ) ;
#23497=ORIENTED_EDGE ( 'NONE', *, *, #11670, .T. ) ;
#23508=CARTESIAN_POINT ( 'NONE',  ( 0.000000000000000000, 3.524919873834583163E-15, 68.31122994652405112 ) ) ;
#23512=FACE_OUTER_BOUND ( 'NONE', #30840, .T. ) ;
#23517=VECTOR ( 'NONE', #22044, 1000.000000000000000 ) ;
#23522=CIRCLE ( 'NONE', #11035, 2.033421858999711507 ) ;
#23526=ORIENTED_EDGE ( 'NONE', *, *, #32010, .T. ) ;
#23527=ORIENTED_EDGE ( 'NONE', *, *, #6773, .F. ) ;
#23529=EDGE_CURVE ( 'NONE', #3883, #8463, #1756, .T. ) ;
#23531=ORIENTED_EDGE ( 'NONE', *, *, #5037, .T. ) ;
#23539=CARTESIAN_POINT ( 'NONE',  ( 10.00000000000000000, 2.296212748401288367E-15, 87.50000000000000000 ) ) ;
#23540=DIRECTION ( 'NONE',  ( -1.000000000000000000, 0.000000000000000000, 0.000000000000000000 ) ) ;
#23547=EDGE_CURVE ( 'NONE', #29867, #11190, #28342, .T. ) ;
#23551=DIRECTION ( 'NONE',  ( 3.697785493223492838E-32, 1.934419779023891545E-16, -1.000000000000000000 ) ) ;
#23560=FACE_OUTER_BOUND ( 'NONE', #5739, .T. ) ;
#23562=AXIS2_PLACEMENT_3D ( 'NONE', #16196, #23661, #7446 ) ;
#23564=DIRECTION ( 'NONE',  ( 0.000000000000000000, -1.000000000000000000, -3.083952846180991760E-16 ) ) ;
#23575=ORIENTED_EDGE ( 'NONE', *, *, #21570, .T. ) ;
#23582=ORIENTED_EDGE ( 'NONE', *, *, #6965, .F. ) ;
#23592=CARTESIAN_POINT ( 'NONE',  ( -43.31669544645773584, 30.33919503331657808, 6.106833536353696523 ) ) ;
#23594=ORIENTED_EDGE ( 'NONE', *, *, #2027, .F. ) ;
#23595=PLANE ( 'NONE',  #13953 ) ;
#23597=ORIENTED_EDGE ( 'NONE', *, *, #22760, .T. ) ;
#23598=CARTESIAN_POINT ( 'NONE',  ( -34.66645501699844090, -15.21971901163155216, 68.31122994652405112 ) ) ;
#23603=VERTEX_POINT ( 'NONE', #3934 ) ;
#23604=DIRECTION ( 'NONE',  ( 1.000000000000000000, 0.000000000000000000, 0.000000000000000000 ) ) ;
#23611=AXIS2_PLACEMENT_3D ( 'NONE', #31745, #5040, #34254 ) ;
#23612=LINE ( 'NONE', #7394, #29864 ) ;
#23615=VECTOR ( 'NONE', #7190, 1000.000000000000000 ) ;
#23621=DIRECTION ( 'NONE',  ( 0.000000000000000000, 0.000000000000000000, 1.000000000000000000 ) ) ;
#23638=ORIENTED_EDGE ( 'NONE', *, *, #16252, .T. ) ;
#23639=VECTOR ( 'NONE', #5897, 1000.000000000000000 ) ;
#23641=EDGE_CURVE ( 'NONE', #8202, #12737, #3770, .T. ) ;
#23644=ORIENTED_EDGE ( 'NONE', *, *, #10963, .F. ) ;
#23646=EDGE_LOOP ( 'NONE', ( #25720, #8288, #16757, #18409 ) ) ;
#23652=CARTESIAN_POINT ( 'NONE',  ( 11.62236370382047923, -30.39942490923500884, 49.43553178847298568 ) ) ;
#23654=VERTEX_POINT ( 'NONE', #33670 ) ;
#23657=ORIENTED_EDGE ( 'NONE', *, *, #27957, .F. ) ;
#23658=VECTOR ( 'NONE', #24729, 1000.000000000000114 ) ;
#23659=CARTESIAN_POINT ( 'NONE',  ( 3.235562306570555532E-30, 18.16264470403145381, -87.50000000000000000 ) ) ;
#23661=DIRECTION ( 'NONE',  ( -0.000000000000000000, -0.000000000000000000, -1.000000000000000000 ) ) ;
#23667=AXIS2_PLACEMENT_3D ( 'NONE', #13568, #24759, #32941 ) ;
#23669=PLANE ( 'NONE',  #11299 ) ;
#23671=ORIENTED_EDGE ( 'NONE', *, *, #18809, .F. ) ;
#23673=EDGE_CURVE ( 'NONE', #4640, #4766, #23691, .T. ) ;
#23677=LINE ( 'NONE', #29192, #27818 ) ;
#23681=VERTEX_POINT ( 'NONE', #31689 ) ;
#23691=LINE ( 'NONE', #29021, #23902 ) ;
#23697=VECTOR ( 'NONE', #26472, 999.9999999999998863 ) ;
#23701=ORIENTED_EDGE ( 'NONE', *, *, #32961, .F. ) ;
#23703=ORIENTED_EDGE ( 'NONE', *, *, #15224, .T. ) ;
#23707=DIRECTION ( 'NONE',  ( 0.9985334138511239299, 0.05413890858541756113, -0.000000000000000000 ) ) ;
#23712=ORIENTED_EDGE ( 'NONE', *, *, #21058, .F. ) ;
#23717=VECTOR ( 'NONE', #5583, 1000.000000000000000 ) ;
#23721=CARTESIAN_POINT ( 'NONE',  ( -30.76765767668600660, -10.60922306139172555, 68.31122994652405112 ) ) ;
#23722=ORIENTED_EDGE ( 'NONE', *, *, #10375, .T. ) ;
#23723=DIRECTION ( 'NONE',  ( 3.697785493223492838E-32, 1.934419779023891545E-16, -1.000000000000000000 ) ) ;
#23728=CARTESIAN_POINT ( 'NONE',  ( 22.10765473302597073, -16.64466345897532662, -77.50000000000000000 ) ) ;
#23731=VECTOR ( 'NONE', #22546, 1000.000000000000114 ) ;
#23734=DIRECTION ( 'NONE',  ( -0.000000000000000000, 1.836970198721029688E-16, -1.000000000000000000 ) ) ;
#23741=ADVANCED_FACE ( 'NONE', ( #34369 ), #28680, .F. ) ;
#23747=VECTOR ( 'NONE', #11256, 1000.000000000000000 ) ;
#23750=EDGE_CURVE ( 'NONE', #26118, #8857, #9813, .T. ) ;
#23752=CARTESIAN_POINT ( 'NONE',  ( -25.14484813934701535, 2.898127806110619709, -15.07978102403234644 ) ) ;
#23763=CARTESIAN_POINT ( 'NONE',  ( -17.07420202168509604, 33.79163469797341435, 68.31122994652405112 ) ) ;
#23765=ORIENTED_EDGE ( 'NONE', *, *, #15313, .F. ) ;
#23772=LINE ( 'NONE', #34630, #33371 ) ;
#23775=VERTEX_POINT ( 'NONE', #26172 ) ;
#23779=DIRECTION ( 'NONE',  ( -0.6473862847818285804, 0.7621620551276356847, 0.000000000000000000 ) ) ;
#23784=ADVANCED_FACE ( 'NONE', ( #18025 ), #26357, .F. ) ;
#23794=ORIENTED_EDGE ( 'NONE', *, *, #19013, .T. ) ;
#23807=VECTOR ( 'NONE', #4227, 1000.000000000000114 ) ;
#23812=ORIENTED_EDGE ( 'NONE', *, *, #28529, .T. ) ;
#23816=ORIENTED_EDGE ( 'NONE', *, *, #21058, .T. ) ;
#23818=CARTESIAN_POINT ( 'NONE',  ( 27.64943126350855707, -17.16721653852535212, 68.31122994652405112 ) ) ;
#23820=CARTESIAN_POINT ( 'NONE',  ( 3.235562306570555532E-30, 8.235406450278427215, -67.50000000000000000 ) ) ;
#23834=DIRECTION ( 'NONE',  ( 0.000000000000000000, 1.836970198721029441E-16, -1.000000000000000000 ) ) ;
#23849=CARTESIAN_POINT ( 'NONE',  ( 22.89764159710613001, 8.346743312457579833, -77.50000000000000000 ) ) ;
#23852=CARTESIAN_POINT ( 'NONE',  ( 22.10765473302597073, -16.64466345897532662, -77.50000000000000000 ) ) ;
#23857=DIRECTION ( 'NONE',  ( 0.000000000000000000, 1.000000000000000000, 0.000000000000000000 ) ) ;
#23858=DIRECTION ( 'NONE',  ( -1.000000000000000000, -0.000000000000000000, -0.000000000000000000 ) ) ;
#23861=ADVANCED_FACE ( 'NONE', ( #5154 ), #32747, .F. ) ;
#23871=ORIENTED_EDGE ( 'NONE', *, *, #21886, .F. ) ;
#23874=DIRECTION ( 'NONE',  ( 0.000000000000000000, 1.000000000000000000, 0.000000000000000000 ) ) ;
#23875=FACE_OUTER_BOUND ( 'NONE', #31783, .T. ) ;
#23881=LINE ( 'NONE', #2002, #9641 ) ;
#23882=LINE ( 'NONE', #21404, #5146 ) ;
#23884=VERTEX_POINT ( 'NONE', #11393 ) ;
#23889=AXIS2_PLACEMENT_3D ( 'NONE', #30016, #5608, #13306 ) ;
#23893=FACE_OUTER_BOUND ( 'NONE', #14504, .T. ) ;
#23896=CARTESIAN_POINT ( 'NONE',  ( 3.235562306570555532E-30, -15.68591377522703390, -87.50000000000000000 ) ) ;
#23900=EDGE_CURVE ( 'NONE', #32940, #6803, #5678, .T. ) ;
#23902=VECTOR ( 'NONE', #29211, 1000.000000000000000 ) ;
#23905=FACE_BOUND ( 'NONE', #26948, .T. ) ;
#23907=EDGE_LOOP ( 'NONE', ( #4111, #23794, #24816, #17080 ) ) ;
#23912=CARTESIAN_POINT ( 'NONE',  ( -48.14940018563182633, -31.98399783210736302, 40.89330243838653445 ) ) ;
#23921=CARTESIAN_POINT ( 'NONE',  ( 27.64943126350854286, -17.16721653852533791, 49.43553178847298568 ) ) ;
#23922=EDGE_LOOP ( 'NONE', ( #14238, #1747, #23155, #18822 ) ) ;
#23927=CARTESIAN_POINT ( 'NONE',  ( -36.80830595996284416, 8.862931941313773265, 68.31122994652405112 ) ) ;
#23934=ORIENTED_EDGE ( 'NONE', *, *, #19862, .T. ) ;
#23939=VECTOR ( 'NONE', #23540, 1000.000000000000000 ) ;
#23951=CIRCLE ( 'NONE', #13180, 32.54542015209055705 ) ;
#23953=LINE ( 'NONE', #32488, #21008 ) ;
#23956=DIRECTION ( 'NONE',  ( -0.6876994588534233177, 0.7259954919231308423, 0.000000000000000000 ) ) ;
#23959=ORIENTED_EDGE ( 'NONE', *, *, #2532, .T. ) ;
#23960=ORIENTED_EDGE ( 'NONE', *, *, #6081, .F. ) ;
#23962=CARTESIAN_POINT ( 'NONE',  ( -37.69926482250235722, 3.578808500140865156, 68.31122994652405112 ) ) ;
#23968=DIRECTION ( 'NONE',  ( 0.000000000000000000, 1.000000000000000000, 0.000000000000000000 ) ) ;
#23971=DIRECTION ( 'NONE',  ( 0.2149704402110236556, -0.9766205557100866574, -0.000000000000000000 ) ) ;
#23972=LINE ( 'NONE', #29509, #12464 ) ;
#23976=CARTESIAN_POINT ( 'NONE',  ( -35.00000000000000000, -12.29554237047777576, -20.46290632209285576 ) ) ;
#23985=DIRECTION ( 'NONE',  ( -0.000000000000000000, 1.836970198721029934E-16, -1.000000000000000000 ) ) ;
#23988=VERTEX_POINT ( 'NONE', #17637 ) ;
#23989=EDGE_LOOP ( 'NONE', ( #20388, #9125, #31154, #8375 ) ) ;
#24016=DIRECTION ( 'NONE',  ( -0.000000000000000000, -0.000000000000000000, -1.000000000000000000 ) ) ;
#24019=DIRECTION ( 'NONE',  ( -0.000000000000000000, 1.836970198721029934E-16, -1.000000000000000000 ) ) ;
#24024=CONICAL_SURFACE ( 'NONE', #28594, 32.54542015209057126, 1.110254297872109275 ) ;
#24026=VECTOR ( 'NONE', #14293, 1000.000000000000000 ) ;
#24028=CARTESIAN_POINT ( 'NONE',  ( 0.000000000000000000, 2.296212748401288367E-15, 47.49999999999999289 ) ) ;
#24031=DIRECTION ( 'NONE',  ( 0.000000000000000000, -1.000000000000000000, -2.132064625830773463E-16 ) ) ;
#24033=VERTEX_POINT ( 'NONE', #29166 ) ;
#24034=VERTEX_POINT ( 'NONE', #26312 ) ;
#24039=ORIENTED_EDGE ( 'NONE', *, *, #22869, .F. ) ;
#24041=CARTESIAN_POINT ( 'NONE',  ( -9.978866888775733912, -13.65249191622732816, -67.50000000000000000 ) ) ;
#24045=DIRECTION ( 'NONE',  ( 0.000000000000000000, 0.000000000000000000, 1.000000000000000000 ) ) ;
#24060=CARTESIAN_POINT ( 'NONE',  ( 25.76952721012208158, 19.87802405277947315, 68.31122994652405112 ) ) ;
#24063=ADVANCED_FACE ( 'NONE', ( #7433 ), #34148, .T. ) ;
#24065=PLANE ( 'NONE',  #9361 ) ;
#24072=FACE_OUTER_BOUND ( 'NONE', #23346, .T. ) ;
#24074=AXIS2_PLACEMENT_3D ( 'NONE', #8453, #14160, #32650 ) ;
#24081=FACE_BOUND ( 'NONE', #6565, .T. ) ;
#24088=ORIENTED_EDGE ( 'NONE', *, *, #3893, .F. ) ;
#24090=FACE_OUTER_BOUND ( 'NONE', #2244, .T. ) ;
#24091=CIRCLE ( 'NONE', #17886, 2.033421858999711951 ) ;
#24094=CARTESIAN_POINT ( 'NONE',  ( 60.00000000000000000, -33.69708579775584667, -49.43553178847298568 ) ) ;
#24097=DIRECTION ( 'NONE',  ( -0.000000000000000000, -1.000000000000000000, -0.000000000000000000 ) ) ;
#24099=ADVANCED_FACE ( 'NONE', ( #12980 ), #9607, .F. ) ;
#24103=ORIENTED_EDGE ( 'NONE', *, *, #22258, .F. ) ;
#24104=AXIS2_PLACEMENT_3D ( 'NONE', #29787, #2727, #2550 ) ;
#24110=VERTEX_POINT ( 'NONE', #15480 ) ;
#24111=CARTESIAN_POINT ( 'NONE',  ( -21.67835495107042476, 31.04982069277122747, 68.31122994652405112 ) ) ;
#24112=ORIENTED_EDGE ( 'NONE', *, *, #3849, .F. ) ;
#24114=LINE ( 'NONE', #2584, #5147 ) ;
#24115=EDGE_CURVE ( 'NONE', #16456, #10877, #30187, .T. ) ;
#24116=VECTOR ( 'NONE', #2730, 1000.000000000000000 ) ;
#24128=ORIENTED_EDGE ( 'NONE', *, *, #2432, .T. ) ;
#24137=ORIENTED_EDGE ( 'NONE', *, *, #31930, .F. ) ;
#24143=LINE ( 'NONE', #21316, #3114 ) ;
#24152=FACE_OUTER_BOUND ( 'NONE', #4442, .T. ) ;
#24153=EDGE_CURVE ( 'NONE', #8593, #22052, #16183, .T. ) ;
#24154=DIRECTION ( 'NONE',  ( 0.000000000000000000, 1.836970198721029688E-16, -1.000000000000000000 ) ) ;
#24155=ORIENTED_EDGE ( 'NONE', *, *, #7340, .T. ) ;
#24157=VECTOR ( 'NONE', #11394, 1000.000000000000227 ) ;
#24158=DIRECTION ( 'NONE',  ( 0.000000000000000000, 1.000000000000000000, 0.000000000000000000 ) ) ;
#24168=EDGE_CURVE ( 'NONE', #2999, #28220, #13154, .T. ) ;
#24171=ORIENTED_EDGE ( 'NONE', *, *, #22022, .T. ) ;
#24173=VECTOR ( 'NONE', #34235, 1000.000000000000114 ) ;
#24174=CARTESIAN_POINT ( 'NONE',  ( 22.10765473302597073, -16.64466345897532307, -87.50000000000000000 ) ) ;
#24177=PLANE ( 'NONE',  #14103 ) ;
#24181=CARTESIAN_POINT ( 'NONE',  ( -41.91768190017683793, 16.36789378607383583, -36.69384042039221328 ) ) ;
#24187=VECTOR ( 'NONE', #19113, 1000.000000000000114 ) ;
#24190=ORIENTED_EDGE ( 'NONE', *, *, #28764, .F. ) ;
#24191=LINE ( 'NONE', #32207, #8351 ) ;
#24193=DIRECTION ( 'NONE',  ( 0.000000000000000000, 1.000000000000000000, 0.000000000000000000 ) ) ;
#24196=VECTOR ( 'NONE', #24800, 1000.000000000000000 ) ;
#24203=DIRECTION ( 'NONE',  ( 0.000000000000000000, 1.836970198721029441E-16, -1.000000000000000000 ) ) ;
#24204=DIRECTION ( 'NONE',  ( -0.000000000000000000, -1.836970198721029688E-16, 1.000000000000000000 ) ) ;
#24205=CARTESIAN_POINT ( 'NONE',  ( -31.87924797510909869, -6.551177101682124970, 68.31122994652405112 ) ) ;
#24207=LINE ( 'NONE', #35086, #13359 ) ;
#24209=VECTOR ( 'NONE', #11760, 1000.000000000000000 ) ;
#24218=ORIENTED_EDGE ( 'NONE', *, *, #19345, .F. ) ;
#24222=ORIENTED_EDGE ( 'NONE', *, *, #32251, .T. ) ;
#24228=ORIENTED_EDGE ( 'NONE', *, *, #13468, .T. ) ;
#24229=VERTEX_POINT ( 'NONE', #5470 ) ;
#24236=ORIENTED_EDGE ( 'NONE', *, *, #33174, .F. ) ;
#24244=CARTESIAN_POINT ( 'NONE',  ( -5.021133111224886036, 4.168562732279004202, -67.50000000000000000 ) ) ;
#24253=ORIENTED_EDGE ( 'NONE', *, *, #20572, .F. ) ;
#24254=AXIS2_PLACEMENT_3D ( 'NONE', #17774, #20437, #25944 ) ;
#24257=VERTEX_POINT ( 'NONE', #2277 ) ;
#24258=DIRECTION ( 'NONE',  ( 0.000000000000000000, -1.000000000000000000, -2.132064625830773463E-16 ) ) ;
#24262=ADVANCED_FACE ( 'NONE', ( #34869 ), #10481, .F. ) ;
#24265=DIRECTION ( 'NONE',  ( -0.2149704402110236556, -0.9766205557100866574, 0.000000000000000000 ) ) ;
#24268=ORIENTED_EDGE ( 'NONE', *, *, #13615, .T. ) ;
#24269=LINE ( 'NONE', #21440, #2599 ) ;
#24271=CARTESIAN_POINT ( 'NONE',  ( -35.00000000000000000, -4.831299144296466785, 15.81122994652406355 ) ) ;
#24275=CARTESIAN_POINT ( 'NONE',  ( -1.307386931792819285, 32.51914993179681090, -36.68877005347593467 ) ) ;
#24277=ORIENTED_EDGE ( 'NONE', *, *, #4625, .F. ) ;
#24278=DIRECTION ( 'NONE',  ( -0.2675283385292199778, 0.9635499925192232418, 1.770012621235684061E-16 ) ) ;
#24281=CARTESIAN_POINT ( 'NONE',  ( 3.235562306570555532E-30, 14.09580098603202458, -67.50000000000000000 ) ) ;
#24286=CARTESIAN_POINT ( 'NONE',  ( 37.86520737902618805, 0.5181781365365116798, 68.31122994652405112 ) ) ;
#24290=EDGE_LOOP ( 'NONE', ( #11100, #15116, #16327, #3530 ) ) ;
#24295=AXIS2_PLACEMENT_3D ( 'NONE', #7725, #29624, #21784 ) ;
#24300=DIRECTION ( 'NONE',  ( 0.1081190184239419622, -0.9941379571543595972, 0.000000000000000000 ) ) ;
#24314=EDGE_CURVE ( 'NONE', #21613, #29231, #17428, .T. ) ;
#24315=LINE ( 'NONE', #13331, #26738 ) ;
#24317=VECTOR ( 'NONE', #1079, 1000.000000000000000 ) ;
#24321=DIRECTION ( 'NONE',  ( -0.2675283385292215321, -0.9635499925192227977, -0.000000000000000000 ) ) ;
#24329=ORIENTED_EDGE ( 'NONE', *, *, #21025, .F. ) ;
#24332=DIRECTION ( 'NONE',  ( 0.000000000000000000, 1.836970198721029688E-16, -1.000000000000000000 ) ) ;
#24340=VERTEX_POINT ( 'NONE', #27719 ) ;
#24344=DIRECTION ( 'NONE',  ( -0.9635499925192230197, -0.2675283385292204774, -0.000000000000000000 ) ) ;
#24346=ORIENTED_EDGE ( 'NONE', *, *, #24747, .F. ) ;
#24357=CARTESIAN_POINT ( 'NONE',  ( -5.021133111225092982, -13.65249191622732461, -87.50000000000000000 ) ) ;
#24358=CARTESIAN_POINT ( 'NONE',  ( 0.000000000000000000, 3.524919873834583163E-15, 68.31122994652405112 ) ) ;
#24364=EDGE_CURVE ( 'NONE', #19626, #10008, #14030, .T. ) ;
#24377=LINE ( 'NONE', #21714, #18326 ) ;
#24380=CIRCLE ( 'NONE', #9631, 2.036051781435508801 ) ;
#24385=CIRCLE ( 'NONE', #13602, 32.54542015209057126 ) ;
#24395=DIRECTION ( 'NONE',  ( -0.000000000000000000, -0.000000000000000000, -1.000000000000000000 ) ) ;
#24398=DIRECTION ( 'NONE',  ( 1.000000000000000000, 0.000000000000000000, 0.000000000000000000 ) ) ;
#24400=ORIENTED_EDGE ( 'NONE', *, *, #11367, .F. ) ;
#24402=DIRECTION ( 'NONE',  ( 0.000000000000000000, 0.000000000000000000, 1.000000000000000000 ) ) ;
#24403=CARTESIAN_POINT ( 'NONE',  ( 0.000000000000000000, 6.992329373473909019E-15, 49.43553178847298568 ) ) ;
#24404=CARTESIAN_POINT ( 'NONE',  ( -5.021133111224989953, -1.691831803474591833, -67.50000000000000000 ) ) ;
#24406=ORIENTED_EDGE ( 'NONE', *, *, #7221, .F. ) ;
#24414=DIRECTION ( 'NONE',  ( 0.000000000000000000, 1.000000000000000000, 0.000000000000000000 ) ) ;
#24427=FACE_BOUND ( 'NONE', #12679, .T. ) ;
#24434=EDGE_LOOP ( 'NONE', ( #2616, #11058, #6667, #27333 ) ) ;
#24438=DIRECTION ( 'NONE',  ( 1.000000000000000000, 0.000000000000000000, 0.000000000000000000 ) ) ;
#24439=FACE_OUTER_BOUND ( 'NONE', #4127, .T. ) ;
#24440=ORIENTED_EDGE ( 'NONE', *, *, #806, .F. ) ;
#24453=LINE ( 'NONE', #16483, #7029 ) ;
#24461=CIRCLE ( 'NONE', #26765, 32.54542015209055705 ) ;
#24464=EDGE_LOOP ( 'NONE', ( #9050, #17729, #31427, #18853 ) ) ;
#24467=EDGE_LOOP ( 'NONE', ( #34988, #21260, #23575, #10652, #22740, #4408, #7382, #26539, #24440, #19164, #19517, #15227, #286, #11307, #29263, #34965, #431, #31934, #35044, #2005, #2157, #33771, #33143, #14354, #25606, #18653, #8602, #15425, #13475, #6630, #16105, #2682, #25546, #34028, #3320, #1536, #26419, #2, #27151, #32099, #25832, #19518, #3641, #22658, #2994, #31245, #28397, #21812, #18088, #27590, #31286, #22775, #3465, #4169, #24277, #34747, #28252, #32539, #22305, #29742, #1301, #20867, #27242, #34755, #3006, #31725, #28183, #10357, #8955, #23472, #28141, #22051, #29877, #28210, #31024, #8168, #26939, #26693, #3400, #25974, #28321, #27145, #33942, #32304 ) ) ;
#24472=CIRCLE ( 'NONE', #13703, 32.54542015209057126 ) ;
#24474=VERTEX_POINT ( 'NONE', #15265 ) ;
#24482=LINE ( 'NONE', #11516, #29301 ) ;
#24485=EDGE_LOOP ( 'NONE', ( #32568, #16181, #3116, #15178 ) ) ;
#24486=AXIS2_PLACEMENT_3D ( 'NONE', #32419, #3050, #10731 ) ;
#24488=DIRECTION ( 'NONE',  ( 0.000000000000000000, 1.836970198721029688E-16, -1.000000000000000000 ) ) ;
#24491=DIRECTION ( 'NONE',  ( 0.000000000000000000, 0.000000000000000000, -1.000000000000000000 ) ) ;
#24499=EDGE_CURVE ( 'NONE', #7307, #9877, #18874, .T. ) ;
#24503=CARTESIAN_POINT ( 'NONE',  ( -45.00000000000000000, 16.36947364650383818, 36.69637551990492597 ) ) ;
#24506=LINE ( 'NONE', #22036, #20591 ) ;
#24511=LINE ( 'NONE', #32359, #7571 ) ;
#24514=VECTOR ( 'NONE', #9053, 1000.000000000000000 ) ;
#24529=VERTEX_POINT ( 'NONE', #25752 ) ;
#24535=EDGE_LOOP ( 'NONE', ( #13462, #25741, #3309, #14798 ) ) ;
#24543=DIRECTION ( 'NONE',  ( 0.000000000000000000, -1.000000000000000000, -1.836970198721029934E-16 ) ) ;
#24550=VECTOR ( 'NONE', #19727, 1000.000000000000114 ) ;
#24551=ORIENTED_EDGE ( 'NONE', *, *, #5654, .F. ) ;
#24552=VECTOR ( 'NONE', #11845, 1000.000000000000000 ) ;
#24553=DIRECTION ( 'NONE',  ( -1.000000000000000000, 0.000000000000000000, 0.000000000000000000 ) ) ;
#24556=ORIENTED_EDGE ( 'NONE', *, *, #11807, .F. ) ;
#24558=ORIENTED_EDGE ( 'NONE', *, *, #25837, .F. ) ;
#24560=EDGE_CURVE ( 'NONE', #22259, #7553, #6870, .T. ) ;
#24563=ORIENTED_EDGE ( 'NONE', *, *, #23435, .F. ) ;
#24565=LINE ( 'NONE', #32762, #33500 ) ;
#24566=ADVANCED_FACE ( 'NONE', ( #10790 ), #11146, .T. ) ;
#24570=ORIENTED_EDGE ( 'NONE', *, *, #7181, .F. ) ;
#24572=FACE_OUTER_BOUND ( 'NONE', #30428, .T. ) ;
#24575=CARTESIAN_POINT ( 'NONE',  ( 10.17231796313409298, 4.274639749586561344, -77.50000000000000000 ) ) ;
#24581=CARTESIAN_POINT ( 'NONE',  ( 22.89764159710613001, 8.346743312457579833, -77.50000000000000000 ) ) ;
#24591=EDGE_LOOP ( 'NONE', ( #23295, #27656, #10744, #17391 ) ) ;
#24593=LINE ( 'NONE', #5029, #21170 ) ;
#24595=VECTOR ( 'NONE', #20371, 1000.000000000000000 ) ;
#24601=EDGE_CURVE ( 'NONE', #22010, #802, #32659, .T. ) ;
#24602=AXIS2_PLACEMENT_3D ( 'NONE', #28940, #32303, #12761 ) ;
#24613=ORIENTED_EDGE ( 'NONE', *, *, #21415, .T. ) ;
#24617=DIRECTION ( 'NONE',  ( -0.000000000000000000, 1.836970198721029688E-16, -1.000000000000000000 ) ) ;
#24618=DIRECTION ( 'NONE',  ( 0.000000000000000000, 1.000000000000000000, 0.000000000000000000 ) ) ;
#24620=LINE ( 'NONE', #19670, #17970 ) ;
#24624=DIRECTION ( 'NONE',  ( 0.000000000000000000, 0.000000000000000000, 1.000000000000000000 ) ) ;
#24625=LINE ( 'NONE', #19493, #6372 ) ;
#24626=LINE ( 'NONE', #27487, #23717 ) ;
#24631=AXIS2_PLACEMENT_3D ( 'NONE', #6205, #14069, #3724 ) ;
#24638=ORIENTED_EDGE ( 'NONE', *, *, #20488, .T. ) ;
#24641=DIRECTION ( 'NONE',  ( 0.000000000000000000, -1.000000000000000000, 0.000000000000000000 ) ) ;
#24643=ORIENTED_EDGE ( 'NONE', *, *, #5479, .T. ) ;
#24646=EDGE_CURVE ( 'NONE', #1704, #16210, #5248, .T. ) ;
#24654=PLANE ( 'NONE',  #31701 ) ;
#24657=LINE ( 'NONE', #16679, #31650 ) ;
#24669=DIRECTION ( 'NONE',  ( 0.000000000000000000, -1.000000000000000000, -2.132064625830773463E-16 ) ) ;
#24670=ORIENTED_EDGE ( 'NONE', *, *, #15699, .F. ) ;
#24671=DIRECTION ( 'NONE',  ( 0.000000000000000000, -1.000000000000000000, 0.000000000000000000 ) ) ;
#24672=DIRECTION ( 'NONE',  ( 0.9476531711828023452, -0.3193015301359802827, -0.000000000000000000 ) ) ;
#24679=VECTOR ( 'NONE', #4870, 1000.000000000000114 ) ;
#24684=ADVANCED_FACE ( 'NONE', ( #7750 ), #18638, .F. ) ;
#24688=FACE_OUTER_BOUND ( 'NONE', #21338, .T. ) ;
#24689=EDGE_CURVE ( 'NONE', #640, #6216, #32513, .T. ) ;
#24691=EDGE_CURVE ( 'NONE', #28031, #18691, #25175, .T. ) ;
#24692=ORIENTED_EDGE ( 'NONE', *, *, #7180, .T. ) ;
#24696=ORIENTED_EDGE ( 'NONE', *, *, #11309, .T. ) ;
#24701=CARTESIAN_POINT ( 'NONE',  ( -9.144464960067640646, -31.23432620483745836, 68.31122994652405112 ) ) ;
#24704=EDGE_LOOP ( 'NONE', ( #659, #34802, #26453, #11982 ) ) ;
#24715=ORIENTED_EDGE ( 'NONE', *, *, #14028, .F. ) ;
#24717=CARTESIAN_POINT ( 'NONE',  ( -29.72561944762172814, -13.25111019240559962, 68.31122994652405112 ) ) ;
#24721=ORIENTED_EDGE ( 'NONE', *, *, #25872, .T. ) ;
#24729=DIRECTION ( 'NONE',  ( 0.9635499925192231307, 0.2675283385292199223, 0.000000000000000000 ) ) ;
#24730=VECTOR ( 'NONE', #18384, 1000.000000000000000 ) ;
#24735=EDGE_CURVE ( 'NONE', #7560, #30758, #30345, .T. ) ;
#24737=ORIENTED_EDGE ( 'NONE', *, *, #30391, .T. ) ;
#24738=CARTESIAN_POINT ( 'NONE',  ( 10.17231796313411429, 15.60017778382161246, -77.50000000000000000 ) ) ;
#24741=VECTOR ( 'NONE', #21250, 1000.000000000000000 ) ;
#24747=EDGE_CURVE ( 'NONE', #6860, #18426, #17202, .T. ) ;
#24749=EDGE_CURVE ( 'NONE', #7373, #18794, #3459, .T. ) ;
#24754=AXIS2_PLACEMENT_3D ( 'NONE', #34087, #7194, #9701 ) ;
#24759=DIRECTION ( 'NONE',  ( -1.000000000000000000, 0.000000000000000000, 0.000000000000000000 ) ) ;
#24760=LINE ( 'NONE', #1053, #17561 ) ;
#24761=VECTOR ( 'NONE', #1143, 1000.000000000000000 ) ;
#24762=DIRECTION ( 'NONE',  ( 0.000000000000000000, -1.000000000000000000, -2.132064625830773463E-16 ) ) ;
#24763=CARTESIAN_POINT ( 'NONE',  ( 8.485274312747506542, 31.41981051364776434, 49.43553178847298568 ) ) ;
#24766=VERTEX_POINT ( 'NONE', #13989 ) ;
#24767=CARTESIAN_POINT ( 'NONE',  ( 3.235562306570555532E-30, -1.691831803474588058, -87.50000000000000000 ) ) ;
#24771=VECTOR ( 'NONE', #14070, 1000.000000000000000 ) ;
#24775=CARTESIAN_POINT ( 'NONE',  ( 3.235562306570555532E-30, 4.168562732279004202, -67.50000000000000000 ) ) ;
#24782=LINE ( 'NONE', #3589, #30878 ) ;
#24786=VECTOR ( 'NONE', #32691, 1000.000000000000000 ) ;
#24793=ORIENTED_EDGE ( 'NONE', *, *, #23079, .F. ) ;
#24795=VECTOR ( 'NONE', #10785, 1000.000000000000000 ) ;
#24797=DIRECTION ( 'NONE',  ( 0.9476531711828030113, 0.3193015301359780622, -0.000000000000000000 ) ) ;
#24798=VERTEX_POINT ( 'NONE', #23976 ) ;
#24800=DIRECTION ( 'NONE',  ( -0.000000000000000000, 1.836970198721029934E-16, -1.000000000000000000 ) ) ;
#24802=CARTESIAN_POINT ( 'NONE',  ( -35.00000000000000000, 0.000000000000000000, 0.000000000000000000 ) ) ;
#24810=DIRECTION ( 'NONE',  ( -0.3193015301359797276, 0.9476531711828024562, -0.000000000000000000 ) ) ;
#24815=DIRECTION ( 'NONE',  ( -1.000000000000000000, 6.792721752314501023E-48, -3.697785493223492838E-32 ) ) ;
#24816=ORIENTED_EDGE ( 'NONE', *, *, #15889, .T. ) ;
#24818=CARTESIAN_POINT ( 'NONE',  ( 18.63894936814906345, 26.67946662374789213, 49.43553178847298568 ) ) ;
#24822=VECTOR ( 'NONE', #33901, 1000.000000000000000 ) ;
#24823=EDGE_CURVE ( 'NONE', #5474, #26209, #22987, .T. ) ;
#24830=VECTOR ( 'NONE', #12654, 1000.000000000000000 ) ;
#24835=EDGE_LOOP ( 'NONE', ( #20743, #2779, #26709, #4906 ) ) ;
#24837=PLANE ( 'NONE',  #21256 ) ;
#24848=AXIS2_PLACEMENT_3D ( 'NONE', #3999, #20056, #14725 ) ;
#24849=CARTESIAN_POINT ( 'NONE',  ( 60.00000000000000000, 0.000000000000000000, 0.000000000000000000 ) ) ;
#24854=EDGE_CURVE ( 'NONE', #20519, #2835, #13785, .T. ) ;
#24865=EDGE_LOOP ( 'NONE', ( #24715, #25240, #6039, #18933 ) ) ;
#24880=VERTEX_POINT ( 'NONE', #12971 ) ;
#24881=ORIENTED_EDGE ( 'NONE', *, *, #3805, .T. ) ;
#24882=ORIENTED_EDGE ( 'NONE', *, *, #13880, .T. ) ;
#24887=ORIENTED_EDGE ( 'NONE', *, *, #22625, .T. ) ;
#24894=ORIENTED_EDGE ( 'NONE', *, *, #19115, .T. ) ;
#24896=CARTESIAN_POINT ( 'NONE',  ( 5.021133111224369117, -5.758675521474015291, -67.50000000000000000 ) ) ;
#24897=EDGE_CURVE ( 'NONE', #30310, #8215, #33081, .T. ) ;
#24907=VECTOR ( 'NONE', #22403, 1000.000000000000000 ) ;
#24926=ORIENTED_EDGE ( 'NONE', *, *, #11212, .T. ) ;
#24928=PLANE ( 'NONE',  #19143 ) ;
#24932=DIRECTION ( 'NONE',  ( 0.000000000000000000, -1.000000000000000000, -1.836970198721029934E-16 ) ) ;
#24935=LINE ( 'NONE', #24767, #23747 ) ;
#24938=ORIENTED_EDGE ( 'NONE', *, *, #22625, .F. ) ;
#24943=DIRECTION ( 'NONE',  ( 0.5155538571770218459, -0.8568571761675891629, 0.000000000000000000 ) ) ;
#24944=CARTESIAN_POINT ( 'NONE',  ( 0.000000000000000000, 3.524919873834583163E-15, 68.31122994652405112 ) ) ;
#24949=DIRECTION ( 'NONE',  ( 0.1617819965527638737, 0.9868265225415262520, -0.000000000000000000 ) ) ;
#24958=VECTOR ( 'NONE', #1363, 1000.000000000000114 ) ;
#24959=ORIENTED_EDGE ( 'NONE', *, *, #25825, .T. ) ;
#24960=CARTESIAN_POINT ( 'NONE',  ( -20.02113311122498729, -3.725253662474303784, -67.50000000000000000 ) ) ;
#24963=CARTESIAN_POINT ( 'NONE',  ( 6.857172176539690689, 37.23415287044793587, 68.31122994652405112 ) ) ;
#24965=AXIS2_PLACEMENT_3D ( 'NONE', #19485, #3435, #30323 ) ;
#24971=CARTESIAN_POINT ( 'NONE',  ( 28.11866956577617316, 16.38733641342591341, 49.43553178847298568 ) ) ;
#24972=LINE ( 'NONE', #5741, #6131 ) ;
#24979=ORIENTED_EDGE ( 'NONE', *, *, #18852, .T. ) ;
#24980=CARTESIAN_POINT ( 'NONE',  ( 0.000000000000000000, 3.524919873834583163E-15, 68.31122994652405112 ) ) ;
#24983=EDGE_CURVE ( 'NONE', #9821, #18812, #33038, .T. ) ;
#24994=CARTESIAN_POINT ( 'NONE',  ( 27.64943126350854286, -17.16721653852534146, 68.31122994652405112 ) ) ;
#24996=ORIENTED_EDGE ( 'NONE', *, *, #11270, .F. ) ;
#24999=CARTESIAN_POINT ( 'NONE',  ( -5.021133111225196011, -23.57973016998034765, -87.50000000000000000 ) ) ;
#25003=DIRECTION ( 'NONE',  ( 0.3193015301359796165, -0.9476531711828025673, 0.000000000000000000 ) ) ;
#25004=EDGE_CURVE ( 'NONE', #16210, #18812, #11175, .T. ) ;
#25006=EDGE_CURVE ( 'NONE', #594, #15054, #14019, .T. ) ;
#25013=DIRECTION ( 'NONE',  ( -4.043477172016612439E-17, 0.000000000000000000, -1.000000000000000000 ) ) ;
#25014=CARTESIAN_POINT ( 'NONE',  ( -9.978866888775527855, 8.235406450278427215, -67.50000000000000000 ) ) ;
#25023=DIRECTION ( 'NONE',  ( -0.000000000000000000, 1.836970198721029934E-16, -1.000000000000000000 ) ) ;
#25028=ORIENTED_EDGE ( 'NONE', *, *, #16538, .F. ) ;
#25033=ORIENTED_EDGE ( 'NONE', *, *, #27882, .T. ) ;
#25037=ORIENTED_EDGE ( 'NONE', *, *, #25438, .F. ) ;
#25041=VECTOR ( 'NONE', #14910, 1000.000000000000227 ) ;
#25044=LINE ( 'NONE', #25405, #23517 ) ;
#25054=FACE_OUTER_BOUND ( 'NONE', #26181, .T. ) ;
#25055=VECTOR ( 'NONE', #28403, 1000.000000000000000 ) ;
#25063=FACE_OUTER_BOUND ( 'NONE', #18253, .T. ) ;
#25074=CARTESIAN_POINT ( 'NONE',  ( 0.000000000000000000, 1.974842713994612024E-15, 76.74945698428001606 ) ) ;
#25076=CARTESIAN_POINT ( 'NONE',  ( -34.04247984038124031, 16.56841925338180488, 68.31122994652405112 ) ) ;
#25091=EDGE_CURVE ( 'NONE', #17595, #22671, #12241, .T. ) ;
#25096=VECTOR ( 'NONE', #4574, 1000.000000000000000 ) ;
#25103=DIRECTION ( 'NONE',  ( 0.000000000000000000, 1.836970198721029441E-16, -1.000000000000000000 ) ) ;
#25109=DIRECTION ( 'NONE',  ( 0.02866416272524433678, 0.5286793732840951998, 0.8483374835754913246 ) ) ;
#25115=DIRECTION ( 'NONE',  ( 0.1081190184239433222, 0.9941379571543594862, 1.826201800709962632E-16 ) ) ;
#25121=AXIS2_PLACEMENT_3D ( 'NONE', #10862, #24016, #18545 ) ;
#25122=AXIS2_PLACEMENT_3D ( 'NONE', #25643, #10285, #1272 ) ;
#25125=LINE ( 'NONE', #4107, #15066 ) ;
#25131=EDGE_CURVE ( 'NONE', #32765, #34117, #33756, .T. ) ;
#25132=ORIENTED_EDGE ( 'NONE', *, *, #11713, .T. ) ;
#25135=EDGE_LOOP ( 'NONE', ( #7064, #31363, #16416, #532, #20904 ) ) ;
#25149=DIRECTION ( 'NONE',  ( 0.000000000000000000, 0.000000000000000000, 1.000000000000000000 ) ) ;
#25150=CARTESIAN_POINT ( 'NONE',  ( 3.235562306570555532E-30, 18.16264470403145381, -87.50000000000000000 ) ) ;
#25159=EDGE_LOOP ( 'NONE', ( #29120, #12469, #24222, #26229 ) ) ;
#25162=FACE_OUTER_BOUND ( 'NONE', #34011, .T. ) ;
#25173=AXIS2_PLACEMENT_3D ( 'NONE', #30300, #11438, #19643 ) ;
#25175=LINE ( 'NONE', #14351, #31956 ) ;
#25178=ORIENTED_EDGE ( 'NONE', *, *, #30977, .F. ) ;
#25179=CARTESIAN_POINT ( 'NONE',  ( -26.18205399241666953, -19.33143609808337615, 68.31122994652405112 ) ) ;
#25182=CARTESIAN_POINT ( 'NONE',  ( 3.235562306570555532E-30, 1.325223266901699007E-14, -67.50000000000000000 ) ) ;
#25190=ADVANCED_FACE ( 'NONE', ( #25740 ), #33571, .F. ) ;
#25192=DIRECTION ( 'NONE',  ( 0.000000000000000000, 0.000000000000000000, -1.000000000000000000 ) ) ;
#25194=DIRECTION ( 'NONE',  ( -0.7621620551276359068, 0.6473862847818281363, 0.000000000000000000 ) ) ;
#25195=DIRECTION ( 'NONE',  ( 0.000000000000000000, 1.836970198721029441E-16, -1.000000000000000000 ) ) ;
#25215=VERTEX_POINT ( 'NONE', #15957 ) ;
#25217=DIRECTION ( 'NONE',  ( 0.000000000000000000, 1.836970198721029688E-16, -1.000000000000000000 ) ) ;
#25218=CARTESIAN_POINT ( 'NONE',  ( -20.02113311122488781, 6.201984591278717041, -67.50000000000000000 ) ) ;
#25225=ORIENTED_EDGE ( 'NONE', *, *, #3162, .T. ) ;
#25226=CARTESIAN_POINT ( 'NONE',  ( -9.978866888775733912, -15.68591377522703390, -87.50000000000000000 ) ) ;
#25228=PLANE ( 'NONE',  #33242 ) ;
#25232=EDGE_CURVE ( 'NONE', #16675, #33409, #16083, .T. ) ;
#25239=CARTESIAN_POINT ( 'NONE',  ( 3.235562306570555532E-30, -15.68591377522703390, -87.50000000000000000 ) ) ;
#25240=ORIENTED_EDGE ( 'NONE', *, *, #13051, .F. ) ;
#25243=ORIENTED_EDGE ( 'NONE', *, *, #6012, .F. ) ;
#25247=ORIENTED_EDGE ( 'NONE', *, *, #29604, .T. ) ;
#25253=VERTEX_POINT ( 'NONE', #26437 ) ;
#25255=DIRECTION ( 'NONE',  ( -0.9766205557100871015, -0.2149704402110223789, -0.000000000000000000 ) ) ;
#25289=LINE ( 'NONE', #32772, #13123 ) ;
#25299=ADVANCED_FACE ( 'NONE', ( #12759 ), #29469, .F. ) ;
#25302=EDGE_CURVE ( 'NONE', #32722, #31704, #31430, .T. ) ;
#25303=FACE_OUTER_BOUND ( 'NONE', #30884, .T. ) ;
#25306=VECTOR ( 'NONE', #14747, 1000.000000000000227 ) ;
#25311=LINE ( 'NONE', #6079, #22422 ) ;
#25318=CARTESIAN_POINT ( 'NONE',  ( -37.12776225901827587, -7.411627343331159246, 15.81122994652406355 ) ) ;
#25320=ORIENTED_EDGE ( 'NONE', *, *, #11761, .T. ) ;
#25323=EDGE_LOOP ( 'NONE', ( #30314, #34497, #21668, #2296 ) ) ;
#25324=DIRECTION ( 'NONE',  ( 0.000000000000000000, -1.000000000000000000, -2.132064625830773463E-16 ) ) ;
#25325=CARTESIAN_POINT ( 'NONE',  ( -32.32899628990712415, -3.747048406849366131, 68.31122994652405112 ) ) ;
#25331=DIRECTION ( 'NONE',  ( 0.000000000000000000, 1.836970198721029934E-16, -1.000000000000000000 ) ) ;
#25341=LINE ( 'NONE', #9674, #20652 ) ;
#25352=AXIS2_PLACEMENT_3D ( 'NONE', #27090, #3402, #11425 ) ;
#25362=ORIENTED_EDGE ( 'NONE', *, *, #20336, .T. ) ;
#25374=DIRECTION ( 'NONE',  ( 0.000000000000000000, 0.8486862100397269959, -0.5288966977476834419 ) ) ;
#25375=AXIS2_PLACEMENT_3D ( 'NONE', #24980, #24624, #17187 ) ;
#25388=EDGE_CURVE ( 'NONE', #6490, #29803, #17240, .T. ) ;
#25394=ADVANCED_FACE ( 'NONE', ( #11306 ), #27664, .F. ) ;
#25404=ORIENTED_EDGE ( 'NONE', *, *, #34834, .F. ) ;
#25405=CARTESIAN_POINT ( 'NONE',  ( 4.815661544189684840, -32.18716788982703747, -36.68877005347593467 ) ) ;
#25408=DIRECTION ( 'NONE',  ( 0.000000000000000000, 1.000000000000000000, 1.934419779023891545E-16 ) ) ;
#25416=AXIS2_PLACEMENT_3D ( 'NONE', #14425, #11569, #14062 ) ;
#25418=VECTOR ( 'NONE', #2958, 1000.000000000000000 ) ;
#25423=DIRECTION ( 'NONE',  ( 3.697785493223492838E-32, 1.934419779023891545E-16, -1.000000000000000000 ) ) ;
#25429=ORIENTED_EDGE ( 'NONE', *, *, #565, .F. ) ;
#25430=FACE_OUTER_BOUND ( 'NONE', #16039, .T. ) ;
#25437=ADVANCED_FACE ( 'NONE', ( #29637 ), #5233, .F. ) ;
#25438=EDGE_CURVE ( 'NONE', #2751, #7906, #13450, .T. ) ;
#25462=DIRECTION ( 'NONE',  ( -1.000000000000000000, -0.000000000000000000, -0.000000000000000000 ) ) ;
#25468=VECTOR ( 'NONE', #23834, 1000.000000000000000 ) ;
#25473=PLANE ( 'NONE',  #22027 ) ;
#25474=DIRECTION ( 'NONE',  ( 0.000000000000000000, 0.000000000000000000, 1.000000000000000000 ) ) ;
#25476=CIRCLE ( 'NONE', #18121, 32.54542015209055705 ) ;
#25478=DIRECTION ( 'NONE',  ( 0.000000000000000000, 1.836970198721029441E-16, -1.000000000000000000 ) ) ;
#25488=VERTEX_POINT ( 'NONE', #8981 ) ;
#25491=ORIENTED_EDGE ( 'NONE', *, *, #6773, .T. ) ;
#25502=DIRECTION ( 'NONE',  ( 0.9868265225415260300, 0.1617819965527648174, 0.000000000000000000 ) ) ;
#25504=ORIENTED_EDGE ( 'NONE', *, *, #5822, .T. ) ;
#25505=CARTESIAN_POINT ( 'NONE',  ( 0.000000000000000000, 3.214697847761802057E-14, -87.50000000000000000 ) ) ;
#25508=LINE ( 'NONE', #17877, #2888 ) ;
#25514=CARTESIAN_POINT ( 'NONE',  ( 17.27856612038528894, 33.69708579775584667, -36.68877005347592757 ) ) ;
#25518=DIRECTION ( 'NONE',  ( 0.7621620551276362399, 0.6473862847818278032, 0.000000000000000000 ) ) ;
#25523=CARTESIAN_POINT ( 'NONE',  ( -37.12776225901827587, -7.411627343331159246, 68.31122994652405112 ) ) ;
#25524=VERTEX_POINT ( 'NONE', #9513 ) ;
#25526=DIRECTION ( 'NONE',  ( -0.6876994588534234287, 0.7259954919231307313, 1.333632083068605180E-16 ) ) ;
#25530=DIRECTION ( 'NONE',  ( -0.8854131517428555087, 0.2458337514780908895, -0.3944734685057937895 ) ) ;
#25546=ORIENTED_EDGE ( 'NONE', *, *, #12675, .F. ) ;
#25549=CARTESIAN_POINT ( 'NONE',  ( 37.55078559520313775, -4.831299144296470338, 49.43553178847298568 ) ) ;
#25551=PLANE ( 'NONE',  #3272 ) ;
#25553=DIRECTION ( 'NONE',  ( 0.9289767198167914186, 0.3701381553399144542, -0.000000000000000000 ) ) ;
#25554=CIRCLE ( 'NONE', #12507, 32.54542015209054995 ) ;
#25557=ORIENTED_EDGE ( 'NONE', *, *, #6056, .T. ) ;
#25566=DIRECTION ( 'NONE',  ( 0.000000000000000000, 1.836970198721029441E-16, -1.000000000000000000 ) ) ;
#25575=DIRECTION ( 'NONE',  ( 0.000000000000000000, 1.000000000000000000, 0.000000000000000000 ) ) ;
#25586=ORIENTED_EDGE ( 'NONE', *, *, #32847, .T. ) ;
#25587=ORIENTED_EDGE ( 'NONE', *, *, #7985, .T. ) ;
#25591=LINE ( 'NONE', #4042, #19048 ) ;
#25593=ORIENTED_EDGE ( 'NONE', *, *, #13880, .F. ) ;
#25597=ORIENTED_EDGE ( 'NONE', *, *, #27817, .T. ) ;
#25598=LINE ( 'NONE', #22768, #23238 ) ;
#25603=EDGE_LOOP ( 'NONE', ( #33113, #27940, #3521, #11929, #14664, #29113, #30270, #33317, #28647, #26288, #11216, #10841 ) ) ;
#25606=ORIENTED_EDGE ( 'NONE', *, *, #24115, .F. ) ;
#25608=DIRECTION ( 'NONE',  ( 0.000000000000000000, -1.000000000000000000, 0.000000000000000000 ) ) ;
#25611=VECTOR ( 'NONE', #1024, 1000.000000000000000 ) ;
#25631=VECTOR ( 'NONE', #29673, 1000.000000000000114 ) ;
#25633=EDGE_LOOP ( 'NONE', ( #29435, #15839, #17958, #8492, #1978, #23959 ) ) ;
#25643=CARTESIAN_POINT ( 'NONE',  ( 0.000000000000000000, 3.524919873834583163E-15, 68.31122994652405112 ) ) ;
#25645=AXIS2_PLACEMENT_3D ( 'NONE', #23721, #31886, #26038 ) ;
#25646=CARTESIAN_POINT ( 'NONE',  ( 0.000000000000000000, 3.524919873834583163E-15, 68.31122994652405112 ) ) ;
#25649=VECTOR ( 'NONE', #34394, 1000.000000000000000 ) ;
#25651=LINE ( 'NONE', #1452, #1426 ) ;
#25659=EDGE_CURVE ( 'NONE', #15297, #750, #7164, .T. ) ;
#25670=ORIENTED_EDGE ( 'NONE', *, *, #3225, .F. ) ;
#25671=ORIENTED_EDGE ( 'NONE', *, *, #20389, .T. ) ;
#25677=ORIENTED_EDGE ( 'NONE', *, *, #8948, .T. ) ;
#25679=ADVANCED_FACE ( 'NONE', ( #15919 ), #30294, .F. ) ;
#25681=CARTESIAN_POINT ( 'NONE',  ( -30.91434716440808117, 10.17386417614053684, 68.31122994652405112 ) ) ;
#25687=AXIS2_PLACEMENT_3D ( 'NONE', #2113, #32000, #18513 ) ;
#25694=VECTOR ( 'NONE', #13192, 1000.000000000000000 ) ;
#25697=CARTESIAN_POINT ( 'NONE',  ( -26.18205399241665177, -19.33143609808336549, 68.31122994652405112 ) ) ;
#25699=LINE ( 'NONE', #29060, #5932 ) ;
#25714=VECTOR ( 'NONE', #21185, 1000.000000000000114 ) ;
#25720=ORIENTED_EDGE ( 'NONE', *, *, #1121, .T. ) ;
#25721=ORIENTED_EDGE ( 'NONE', *, *, #12239, .T. ) ;
#25726=ORIENTED_EDGE ( 'NONE', *, *, #22881, .T. ) ;
#25730=LINE ( 'NONE', #1356, #19225 ) ;
#25731=LINE ( 'NONE', #1357, #1081 ) ;
#25740=FACE_OUTER_BOUND ( 'NONE', #26622, .T. ) ;
#25741=ORIENTED_EDGE ( 'NONE', *, *, #30697, .F. ) ;
#25745=EDGE_LOOP ( 'NONE', ( #29818, #6175, #19778, #3634 ) ) ;
#25746=LINE ( 'NONE', #26095, #25041 ) ;
#25747=DIRECTION ( 'NONE',  ( -0.5155538571770220679, -0.8568571761675890519, 0.000000000000000000 ) ) ;
#25750=ADVANCED_FACE ( 'NONE', ( #13582 ), #2709, .T. ) ;
#25752=CARTESIAN_POINT ( 'NONE',  ( 10.17231796313411429, 17.63622956525712482, -87.50000000000000000 ) ) ;
#25765=EDGE_LOOP ( 'NONE', ( #23582, #11439, #11592, #26858 ) ) ;
#25766=VERTEX_POINT ( 'NONE', #44 ) ;
#25781=CARTESIAN_POINT ( 'NONE',  ( 3.235562306570555532E-30, 28.08988295778447508, -87.50000000000000000 ) ) ;
#25782=VERTEX_POINT ( 'NONE', #32782 ) ;
#25789=VECTOR ( 'NONE', #31054, 1000.000000000000000 ) ;
#25790=VECTOR ( 'NONE', #22778, 1000.000000000000000 ) ;
#25796=ORIENTED_EDGE ( 'NONE', *, *, #12163, .F. ) ;
#25802=DIRECTION ( 'NONE',  ( 1.000000000000000000, 0.000000000000000000, 0.000000000000000000 ) ) ;
#25808=FACE_OUTER_BOUND ( 'NONE', #23907, .T. ) ;
#25809=EDGE_LOOP ( 'NONE', ( #17042, #29482, #9961, #19304 ) ) ;
#25810=CARTESIAN_POINT ( 'NONE',  ( 32.05156013847309993, -20.15193397489277771, 68.31122994652405112 ) ) ;
#25814=ORIENTED_EDGE ( 'NONE', *, *, #6672, .T. ) ;
#25819=LINE ( 'NONE', #17832, #34734 ) ;
#25825=EDGE_CURVE ( 'NONE', #3836, #20902, #33490, .T. ) ;
#25828=DIRECTION ( 'NONE',  ( -1.000000000000000000, 0.000000000000000000, 0.000000000000000000 ) ) ;
#25830=DIRECTION ( 'NONE',  ( 0.9941379571543595972, 0.1081190184239419622, 1.986114147597513362E-17 ) ) ;
#25832=ORIENTED_EDGE ( 'NONE', *, *, #1754, .F. ) ;
#25837=EDGE_CURVE ( 'NONE', #4182, #3468, #28155, .T. ) ;
#25840=ORIENTED_EDGE ( 'NONE', *, *, #14604, .F. ) ;
#25842=EDGE_CURVE ( 'NONE', #34696, #22911, #33321, .T. ) ;
#25848=FACE_OUTER_BOUND ( 'NONE', #136, .T. ) ;
#25849=VERTEX_POINT ( 'NONE', #33136 ) ;
#25850=ORIENTED_EDGE ( 'NONE', *, *, #23244, .F. ) ;
#25863=AXIS2_PLACEMENT_3D ( 'NONE', #27740, #3353, #4224 ) ;
#25867=ORIENTED_EDGE ( 'NONE', *, *, #23641, .T. ) ;
#25872=EDGE_CURVE ( 'NONE', #16741, #11336, #22290, .T. ) ;
#25878=FACE_OUTER_BOUND ( 'NONE', #29900, .T. ) ;
#25882=CARTESIAN_POINT ( 'NONE',  ( -20.02113311122509032, -13.65249191622732461, -87.50000000000000000 ) ) ;
#25889=ORIENTED_EDGE ( 'NONE', *, *, #25131, .T. ) ;
#25890=ADVANCED_FACE ( 'NONE', ( #8935 ), #16974, .F. ) ;
#25893=DIRECTION ( 'NONE',  ( 1.000000000000000000, 0.000000000000000000, 0.000000000000000000 ) ) ;
#25896=ORIENTED_EDGE ( 'NONE', *, *, #14773, .F. ) ;
#25902=CARTESIAN_POINT ( 'NONE',  ( 32.54460952423469422, 0.2297037030477300235, 49.43553178847298568 ) ) ;
#25910=ADVANCED_FACE ( 'NONE', ( #11802 ), #22652, .F. ) ;
#25913=VERTEX_POINT ( 'NONE', #30480 ) ;
#25922=EDGE_CURVE ( 'NONE', #28173, #22010, #22992, .T. ) ;
#25925=ORIENTED_EDGE ( 'NONE', *, *, #23529, .F. ) ;
#25926=FACE_OUTER_BOUND ( 'NONE', #34431, .T. ) ;
#25927=EDGE_LOOP ( 'NONE', ( #16022, #25557, #3467, #14658 ) ) ;
#25931=VECTOR ( 'NONE', #4895, 1000.000000000000000 ) ;
#25942=LINE ( 'NONE', #34118, #20158 ) ;
#25943=CARTESIAN_POINT ( 'NONE',  ( -10.84269519964070305, -36.27449394610879096, 68.31122994652405112 ) ) ;
#25944=DIRECTION ( 'NONE',  ( -0.8568571761675893850, -0.5155538571770214018, 0.000000000000000000 ) ) ;
#25945=CARTESIAN_POINT ( 'NONE',  ( -23.93921925319781963, 29.33115633223345142, 68.31122994652405112 ) ) ;
#25947=ORIENTED_EDGE ( 'NONE', *, *, #19614, .F. ) ;
#25955=CARTESIAN_POINT ( 'NONE',  ( 20.62763069236413926, -31.74750072459299588, 49.43553178847298568 ) ) ;
#25974=ORIENTED_EDGE ( 'NONE', *, *, #6250, .T. ) ;
#25976=CARTESIAN_POINT ( 'NONE',  ( -21.41424479178918361, -24.50784553716280101, 68.31122994652405112 ) ) ;
#25977=VECTOR ( 'NONE', #9106, 1000.000000000000000 ) ;
#25978=LINE ( 'NONE', #1083, #31275 ) ;
#25981=DIRECTION ( 'NONE',  ( 0.000000000000000000, -1.000000000000000000, -1.836970198721029934E-16 ) ) ;
#25982=DIRECTION ( 'NONE',  ( -1.000000000000000000, 0.000000000000000000, 0.000000000000000000 ) ) ;
#25987=CARTESIAN_POINT ( 'NONE',  ( -37.69926482250235722, 3.578808500140865156, 68.31122994652405112 ) ) ;
#25993=CARTESIAN_POINT ( 'NONE',  ( -5.021133111224989953, -1.691831803474591833, -67.50000000000000000 ) ) ;
#26000=ORIENTED_EDGE ( 'NONE', *, *, #29805, .F. ) ;
#26001=LINE ( 'NONE', #3762, #25977 ) ;
#26011=CARTESIAN_POINT ( 'NONE',  ( 2.658817013151218312E-15, -10.87635688602997597, 87.50000000000000000 ) ) ;
#26013=AXIS2_PLACEMENT_3D ( 'NONE', #30509, #6104, #3089 ) ;
#26014=VERTEX_POINT ( 'NONE', #7122 ) ;
#26016=EDGE_LOOP ( 'NONE', ( #12633, #32085, #29170, #30018 ) ) ;
#26020=ORIENTED_EDGE ( 'NONE', *, *, #15107, .T. ) ;
#26021=VERTEX_POINT ( 'NONE', #1620 ) ;
#26023=ADVANCED_FACE ( 'NONE', ( #28505 ), #28676, .F. ) ;
#26025=VECTOR ( 'NONE', #32361, 1000.000000000000000 ) ;
#26026=VECTOR ( 'NONE', #19003, 1000.000000000000000 ) ;
#26029=CARTESIAN_POINT ( 'NONE',  ( -35.00000000000000000, 45.00000000000000711, -36.68877005347592757 ) ) ;
#26035=EDGE_CURVE ( 'NONE', #7776, #15307, #34189, .T. ) ;
#26038=DIRECTION ( 'NONE',  ( 0.9289767198167915296, 0.3701381553399144542, 0.000000000000000000 ) ) ;
#26039=ORIENTED_EDGE ( 'NONE', *, *, #10922, .T. ) ;
#26050=CARTESIAN_POINT ( 'NONE',  ( 5.021133111224162171, -25.61315202898006049, -67.50000000000000000 ) ) ;
#26054=CARTESIAN_POINT ( 'NONE',  ( 28.11866956577617316, 16.38733641342590985, 68.31122994652405112 ) ) ;
#26068=ORIENTED_EDGE ( 'NONE', *, *, #22257, .T. ) ;
#26072=CARTESIAN_POINT ( 'NONE',  ( 23.31255882915078814, -22.70966696615089830, 68.31122994652405112 ) ) ;
#26074=ORIENTED_EDGE ( 'NONE', *, *, #20590, .F. ) ;
#26079=EDGE_CURVE ( 'NONE', #31010, #19356, #9983, .T. ) ;
#26082=EDGE_LOOP ( 'NONE', ( #31096, #21758, #25037, #15252 ) ) ;
#26083=VECTOR ( 'NONE', #11907, 1000.000000000000000 ) ;
#26093=DIRECTION ( 'NONE',  ( 3.697785493223492838E-32, 1.934419779023891545E-16, -1.000000000000000000 ) ) ;
#26095=CARTESIAN_POINT ( 'NONE',  ( -34.04247984038124031, 16.56841925338182619, -36.68877005347593467 ) ) ;
#26099=AXIS2_PLACEMENT_3D ( 'NONE', #33166, #13788, #24438 ) ;
#26102=DIRECTION ( 'NONE',  ( 0.000000000000000000, 1.836970198721029441E-16, -1.000000000000000000 ) ) ;
#26113=VECTOR ( 'NONE', #787, 1000.000000000000000 ) ;
#26118=VERTEX_POINT ( 'NONE', #5 ) ;
#26121=CARTESIAN_POINT ( 'NONE',  ( -5.021133111224782120, 16.12922284503173742, -67.50000000000000000 ) ) ;
#26131=VERTEX_POINT ( 'NONE', #35081 ) ;
#26136=AXIS2_PLACEMENT_3D ( 'NONE', #16500, #2247, #30009 ) ;
#26138=DIRECTION ( 'NONE',  ( 1.000000000000000000, 0.000000000000000000, 0.000000000000000000 ) ) ;
#26147=DIRECTION ( 'NONE',  ( 0.000000000000000000, 1.000000000000000000, 1.836970198721029688E-16 ) ) ;
#26153=DIRECTION ( 'NONE',  ( 0.000000000000000000, 1.836970198721029441E-16, -1.000000000000000000 ) ) ;
#26155=VERTEX_POINT ( 'NONE', #13539 ) ;
#26158=VERTEX_POINT ( 'NONE', #10866 ) ;
#26160=DIRECTION ( 'NONE',  ( -1.000000000000000000, 6.792721752314501023E-48, -3.697785493223492838E-32 ) ) ;
#26164=ORIENTED_EDGE ( 'NONE', *, *, #14527, .F. ) ;
#26167=DIRECTION ( 'NONE',  ( -0.000000000000000000, -1.836970198721029688E-16, 1.000000000000000000 ) ) ;
#26172=CARTESIAN_POINT ( 'NONE',  ( 1.991296462759137853, -32.48444414290483451, 68.31122994652405112 ) ) ;
#26176=ADVANCED_FACE ( 'NONE', ( #13892 ), #19241, .T. ) ;
#26181=EDGE_LOOP ( 'NONE', ( #31234, #13339, #2375, #27844, #12905 ) ) ;
#26185=VECTOR ( 'NONE', #2237, 1000.000000000000000 ) ;
#26189=ORIENTED_EDGE ( 'NONE', *, *, #26740, .F. ) ;
#26190=PLANE ( 'NONE',  #1993 ) ;
#26193=FACE_OUTER_BOUND ( 'NONE', #33475, .T. ) ;
#26194=LINE ( 'NONE', #26029, #25649 ) ;
#26195=ORIENTED_EDGE ( 'NONE', *, *, #34982, .T. ) ;
#26206=DIRECTION ( 'NONE',  ( 0.000000000000000000, 0.000000000000000000, 1.000000000000000000 ) ) ;
#26209=VERTEX_POINT ( 'NONE', #29383 ) ;
#26210=FACE_OUTER_BOUND ( 'NONE', #7491, .T. ) ;
#26213=CARTESIAN_POINT ( 'NONE',  ( -18.07349068442141515, -27.06572199953720315, -36.68877005347593467 ) ) ;
#26215=AXIS2_PLACEMENT_3D ( 'NONE', #6939, #4089, #28144 ) ;
#26218=CARTESIAN_POINT ( 'NONE',  ( -30.76765767668601725, -10.60922306139169891, -36.68877005347593467 ) ) ;
#26228=ADVANCED_FACE ( 'NONE', ( #16044 ), #16402, .T. ) ;
#26229=ORIENTED_EDGE ( 'NONE', *, *, #21764, .T. ) ;
#26232=CARTESIAN_POINT ( 'NONE',  ( -37.85301660235036536, 0.7430237821112765095, -36.68877005347593467 ) ) ;
#26233=ORIENTED_EDGE ( 'NONE', *, *, #7221, .T. ) ;
#26245=CARTESIAN_POINT ( 'NONE',  ( 3.235562306570555532E-30, 8.235406450278430768, -87.50000000000000000 ) ) ;
#26249=FACE_OUTER_BOUND ( 'NONE', #15990, .T. ) ;
#26250=FACE_OUTER_BOUND ( 'NONE', #9048, .T. ) ;
#26260=EDGE_LOOP ( 'NONE', ( #1506, #34268, #11700, #9172 ) ) ;
#26265=DIRECTION ( 'NONE',  ( -0.9476531711828023452, 0.3193015301359802827, 0.000000000000000000 ) ) ;
#26270=ORIENTED_EDGE ( 'NONE', *, *, #18854, .T. ) ;
#26271=AXIS2_PLACEMENT_3D ( 'NONE', #19161, #11676, #804 ) ;
#26287=ORIENTED_EDGE ( 'NONE', *, *, #15040, .F. ) ;
#26288=ORIENTED_EDGE ( 'NONE', *, *, #24314, .T. ) ;
#26294=VECTOR ( 'NONE', #10576, 1000.000000000000000 ) ;
#26297=CIRCLE ( 'NONE', #20072, 2.036051781435510577 ) ;
#26301=CARTESIAN_POINT ( 'NONE',  ( -35.00000000000000000, 42.49491490430484220, 36.69637551990492597 ) ) ;
#26306=ORIENTED_EDGE ( 'NONE', *, *, #10436, .F. ) ;
#26309=CARTESIAN_POINT ( 'NONE',  ( 0.000000000000000000, 1.974842713994612024E-15, 76.74945698428001606 ) ) ;
#26312=CARTESIAN_POINT ( 'NONE',  ( 27.99209646187090783, 25.49206711720158225, 49.43553178847298568 ) ) ;
#26313=DIRECTION ( 'NONE',  ( 0.000000000000000000, 1.836970198721029688E-16, -1.000000000000000000 ) ) ;
#26314=DIRECTION ( 'NONE',  ( -0.3193015301359797831, 0.9476531711828025673, 0.000000000000000000 ) ) ;
#26320=EDGE_CURVE ( 'NONE', #11743, #2097, #22429, .T. ) ;
#26333=FACE_OUTER_BOUND ( 'NONE', #23298, .T. ) ;
#26337=ORIENTED_EDGE ( 'NONE', *, *, #21165, .T. ) ;
#26343=ADVANCED_FACE ( 'NONE', ( #33093 ), #30612, .F. ) ;
#26353=CARTESIAN_POINT ( 'NONE',  ( 22.89764159710613001, 4.274639749586560455, -77.50000000000000000 ) ) ;
#26354=EDGE_CURVE ( 'NONE', #6786, #29803, #894, .T. ) ;
#26355=CARTESIAN_POINT ( 'NONE',  ( 1.991296462759137853, -32.48444414290483451, 68.31122994652405112 ) ) ;
#26357=PLANE ( 'NONE',  #18293 ) ;
#26359=DIRECTION ( 'NONE',  ( 0.2675283385292205884, 0.9635499925192231307, 1.770012621235684308E-16 ) ) ;
#26369=VERTEX_POINT ( 'NONE', #32916 ) ;
#26374=ORIENTED_EDGE ( 'NONE', *, *, #32921, .F. ) ;
#26376=DIRECTION ( 'NONE',  ( -0.000000000000000000, -0.000000000000000000, -1.000000000000000000 ) ) ;
#26383=DIRECTION ( 'NONE',  ( -1.000000000000000000, 0.000000000000000000, 0.000000000000000000 ) ) ;
#26387=LINE ( 'NONE', #29055, #35025 ) ;
#26393=CIRCLE ( 'NONE', #15758, 2.085824230283342740 ) ;
#26395=CARTESIAN_POINT ( 'NONE',  ( -30.76765767668601725, -10.60922306139171667, 68.31122994652405112 ) ) ;
#26397=VECTOR ( 'NONE', #33491, 1000.000000000000000 ) ;
#26412=LINE ( 'NONE', #12912, #29262 ) ;
#26415=AXIS2_PLACEMENT_3D ( 'NONE', #13844, #32223, #34541 ) ;
#26419=ORIENTED_EDGE ( 'NONE', *, *, #3205, .F. ) ;
#26423=ADVANCED_FACE ( 'NONE', ( #1752 ), #6910, .F. ) ;
#26428=LINE ( 'NONE', #32459, #33257 ) ;
#26437=CARTESIAN_POINT ( 'NONE',  ( -9.978866888775527855, 8.235406450278427215, -67.50000000000000000 ) ) ;
#26440=AXIS2_PLACEMENT_3D ( 'NONE', #34452, #28589, #33931 ) ;
#26441=CARTESIAN_POINT ( 'NONE',  ( 27.99209646187092559, 25.49206711720156093, 49.43553178847298568 ) ) ;
#26448=VECTOR ( 'NONE', #7045, 1000.000000000000114 ) ;
#26453=ORIENTED_EDGE ( 'NONE', *, *, #11533, .F. ) ;
#26463=ORIENTED_EDGE ( 'NONE', *, *, #33298, .F. ) ;
#26464=EDGE_LOOP ( 'NONE', ( #363, #9295, #29314, #12441 ) ) ;
#26466=VECTOR ( 'NONE', #22856, 1000.000000000000114 ) ;
#26472=DIRECTION ( 'NONE',  ( 0.6051742151937651304, 0.7960930657056438653, -0.000000000000000000 ) ) ;
#26477=FACE_OUTER_BOUND ( 'NONE', #19470, .T. ) ;
#26478=EDGE_CURVE ( 'NONE', #31238, #19439, #9769, .T. ) ;
#26480=CARTESIAN_POINT ( 'NONE',  ( 10.96230482721425403, -14.55883922869198166, -87.50000000000000000 ) ) ;
#26487=CARTESIAN_POINT ( 'NONE',  ( 3.235562306570555532E-30, 24.02303923978504940, -67.50000000000000000 ) ) ;
#26489=LINE ( 'NONE', #2109, #34925 ) ;
#26500=AXIS2_PLACEMENT_3D ( 'NONE', #7746, #18633, #26265 ) ;
#26503=CARTESIAN_POINT ( 'NONE',  ( -37.58721499952019940, -4.609089608337735733, -36.68877005347593467 ) ) ;
#26504=CARTESIAN_POINT ( 'NONE',  ( 0.000000000000000000, 3.214697847761802057E-14, -87.50000000000000000 ) ) ;
#26507=DIRECTION ( 'NONE',  ( -0.9075754196709575616, 0.4198891015602634891, -0.000000000000000000 ) ) ;
#26510=DIRECTION ( 'NONE',  ( 0.000000000000000000, 1.836970198721029688E-16, -1.000000000000000000 ) ) ;
#26522=ORIENTED_EDGE ( 'NONE', *, *, #7420, .T. ) ;
#26523=VECTOR ( 'NONE', #7521, 1000.000000000000227 ) ;
#26525=CARTESIAN_POINT ( 'NONE',  ( 26.04754872656012310, -19.51229300245306320, 49.43553178847298568 ) ) ;
#26526=CARTESIAN_POINT ( 'NONE',  ( 22.89764159710611224, 17.63622956525712127, -77.50000000000000000 ) ) ;
#26539=ORIENTED_EDGE ( 'NONE', *, *, #17155, .F. ) ;
#26540=ADVANCED_FACE ( 'NONE', ( #20802 ), #31647, .F. ) ;
#26546=ORIENTED_EDGE ( 'NONE', *, *, #28719, .F. ) ;
#26549=DIRECTION ( 'NONE',  ( -0.000000000000000000, -0.000000000000000000, -1.000000000000000000 ) ) ;
#26555=DIRECTION ( 'NONE',  ( -0.000000000000000000, 1.836970198721029934E-16, -1.000000000000000000 ) ) ;
#26560=ORIENTED_EDGE ( 'NONE', *, *, #2412, .T. ) ;
#26566=DIRECTION ( 'NONE',  ( -1.000000000000000000, 0.000000000000000000, 0.000000000000000000 ) ) ;
#26570=DIRECTION ( 'NONE',  ( -0.6473862847818285804, -0.7621620551276356847, -0.000000000000000000 ) ) ;
#26577=VECTOR ( 'NONE', #8637, 1000.000000000000000 ) ;
#26578=ORIENTED_EDGE ( 'NONE', *, *, #7289, .F. ) ;
#26579=CARTESIAN_POINT ( 'NONE',  ( 0.000000000000000000, 0.000000000000000000, 0.000000000000000000 ) ) ;
#26580=ADVANCED_FACE ( 'NONE', ( #13151 ), #18509, .F. ) ;
#26595=ORIENTED_EDGE ( 'NONE', *, *, #10665, .F. ) ;
#26622=EDGE_LOOP ( 'NONE', ( #19396, #26287, #21243, #1085 ) ) ;
#26638=AXIS2_PLACEMENT_3D ( 'NONE', #9218, #19734, #16901 ) ;
#26642=ORIENTED_EDGE ( 'NONE', *, *, #27164, .T. ) ;
#26652=CARTESIAN_POINT ( 'NONE',  ( -18.07349068442144358, -27.06572199953721736, 68.31122994652405112 ) ) ;
#26662=LINE ( 'NONE', #29519, #6908 ) ;
#26665=VERTEX_POINT ( 'NONE', #16178 ) ;
#26666=EDGE_CURVE ( 'NONE', #29934, #1639, #26489, .T. ) ;
#26673=ORIENTED_EDGE ( 'NONE', *, *, #6965, .T. ) ;
#26676=ORIENTED_EDGE ( 'NONE', *, *, #5419, .T. ) ;
#26679=AXIS2_PLACEMENT_3D ( 'NONE', #24802, #436, #8784 ) ;
#26683=VERTEX_POINT ( 'NONE', #9158 ) ;
#26688=CARTESIAN_POINT ( 'NONE',  ( 15.44711578872682267, -28.64595934308655600, 68.31122994652405112 ) ) ;
#26689=DIRECTION ( 'NONE',  ( 0.000000000000000000, 1.836970198721029688E-16, -1.000000000000000000 ) ) ;
#26692=CARTESIAN_POINT ( 'NONE',  ( 27.99209646187092559, 25.49206711720156093, 68.31122994652405112 ) ) ;
#26693=ORIENTED_EDGE ( 'NONE', *, *, #32655, .F. ) ;
#26699=DIRECTION ( 'NONE',  ( 0.1617819965527614312, -0.9868265225415265851, -0.000000000000000000 ) ) ;
#26700=ORIENTED_EDGE ( 'NONE', *, *, #29558, .T. ) ;
#26701=CARTESIAN_POINT ( 'NONE',  ( -32.71222340678873053, 19.07754906224033675, 68.31122994652405112 ) ) ;
#26704=DIRECTION ( 'NONE',  ( 0.000000000000000000, -1.000000000000000000, -1.836970198721029934E-16 ) ) ;
#26709=ORIENTED_EDGE ( 'NONE', *, *, #12859, .F. ) ;
#26717=EDGE_CURVE ( 'NONE', #27275, #23058, #20142, .T. ) ;
#26722=CARTESIAN_POINT ( 'NONE',  ( 22.89764159710615132, -5.651112684911595352, -87.50000000000000000 ) ) ;
#26726=EDGE_LOOP ( 'NONE', ( #24268, #25504, #8965, #548 ) ) ;
#26729=CARTESIAN_POINT ( 'NONE',  ( 0.000000000000000000, 6.992329373473909019E-15, 49.43553178847298568 ) ) ;
#26731=PLANE ( 'NONE',  #30748 ) ;
#26738=VECTOR ( 'NONE', #25553, 1000.000000000000000 ) ;
#26740=EDGE_CURVE ( 'NONE', #26683, #29298, #13309, .T. ) ;
#26742=VECTOR ( 'NONE', #21821, 1000.000000000000000 ) ;
#26745=DIRECTION ( 'NONE',  ( 0.000000000000000000, 1.836970198721029441E-16, -1.000000000000000000 ) ) ;
#26751=CARTESIAN_POINT ( 'NONE',  ( -35.00000000000000000, 16.36947364650383818, 36.69637551990492597 ) ) ;
#26752=DIRECTION ( 'NONE',  ( 0.4684084406997908734, -0.8835120444460226041, -1.622985295858433536E-16 ) ) ;
#26756=LINE ( 'NONE', #21951, #26294 ) ;
#26757=VECTOR ( 'NONE', #34819, 1000.000000000000000 ) ;
#26758=ORIENTED_EDGE ( 'NONE', *, *, #21101, .T. ) ;
#26760=EDGE_CURVE ( 'NONE', #2924, #319, #12373, .T. ) ;
#26765=AXIS2_PLACEMENT_3D ( 'NONE', #4181, #22366, #33563 ) ;
#26768=LINE ( 'NONE', #23912, #34464 ) ;
#26774=DIRECTION ( 'NONE',  ( -0.000000000000000000, -1.836970198721029688E-16, 1.000000000000000000 ) ) ;
#26779=ORIENTED_EDGE ( 'NONE', *, *, #31805, .F. ) ;
#26781=AXIS2_PLACEMENT_3D ( 'NONE', #33320, #8752, #28334 ) ;
#26785=PLANE ( 'NONE',  #18053 ) ;
#26789=ORIENTED_EDGE ( 'NONE', *, *, #22760, .F. ) ;
#26791=CARTESIAN_POINT ( 'NONE',  ( 5.021133111224576062, 16.12922284503174097, -87.50000000000000000 ) ) ;
#26793=VECTOR ( 'NONE', #26383, 1000.000000000000000 ) ;
#26794=DIRECTION ( 'NONE',  ( 0.000000000000000000, -0.9836764282395641379, 0.1799463379062027635 ) ) ;
#26802=LINE ( 'NONE', #34647, #10884 ) ;
#26806=VECTOR ( 'NONE', #30921, 1000.000000000000227 ) ;
#26807=AXIS2_PLACEMENT_3D ( 'NONE', #32479, #5250, #13114 ) ;
#26820=FACE_OUTER_BOUND ( 'NONE', #10584, .T. ) ;
#26828=EDGE_CURVE ( 'NONE', #13032, #6490, #15744, .T. ) ;
#26836=CIRCLE ( 'NONE', #25121, 32.54542015209055705 ) ;
#26848=CARTESIAN_POINT ( 'NONE',  ( 17.88561705399011714, -27.19023860642122514, 49.43553178847298568 ) ) ;
#26858=ORIENTED_EDGE ( 'NONE', *, *, #5118, .F. ) ;
#26864=CARTESIAN_POINT ( 'NONE',  ( -35.00000000000000000, -46.95407462254104303, 36.69637551990492597 ) ) ;
#26869=CARTESIAN_POINT ( 'NONE',  ( 5.021133111224679091, 24.02303923978504940, -67.50000000000000000 ) ) ;
#26870=ORIENTED_EDGE ( 'NONE', *, *, #22135, .T. ) ;
#26872=ADVANCED_FACE ( 'NONE', ( #18934 ), #10745, .T. ) ;
#26879=CARTESIAN_POINT ( 'NONE',  ( 22.10765473302597073, -14.55883922869198344, -77.50000000000000000 ) ) ;
#26882=VECTOR ( 'NONE', #15550, 1000.000000000000000 ) ;
#26885=CARTESIAN_POINT ( 'NONE',  ( -35.00000000000000000, -38.34433698000722046, -36.69637551990492597 ) ) ;
#26890=ORIENTED_EDGE ( 'NONE', *, *, #27311, .T. ) ;
#26905=CARTESIAN_POINT ( 'NONE',  ( 0.000000000000000000, 3.524919873834583163E-15, 68.31122994652405112 ) ) ;
#26907=DIRECTION ( 'NONE',  ( 0.000000000000000000, 1.836970198721029441E-16, -1.000000000000000000 ) ) ;
#26908=CARTESIAN_POINT ( 'NONE',  ( 32.54460952423469422, 0.2297037030477265540, 68.31122994652405112 ) ) ;
#26912=DIRECTION ( 'NONE',  ( -0.000000000000000000, 0.8486862100397269959, 0.5288966977476833309 ) ) ;
#26916=CARTESIAN_POINT ( 'NONE',  ( 9.736651044630743712, -33.69708579775584667, 49.43553178847298568 ) ) ;
#26921=AXIS2_PLACEMENT_3D ( 'NONE', #19967, #5886, #27612 ) ;
#26923=ADVANCED_FACE ( 'NONE', ( #16623 ), #21594, .F. ) ;
#26927=DIRECTION ( 'NONE',  ( -0.000000000000000000, 0.8486862100397269959, 0.5288966977476833309 ) ) ;
#26937=EDGE_CURVE ( 'NONE', #5262, #33527, #11437, .T. ) ;
#26939=ORIENTED_EDGE ( 'NONE', *, *, #3485, .T. ) ;
#26942=ORIENTED_EDGE ( 'NONE', *, *, #3205, .T. ) ;
#26945=CARTESIAN_POINT ( 'NONE',  ( 8.485274312747499437, 31.41981051364775013, 68.31122994652405112 ) ) ;
#26946=DIRECTION ( 'NONE',  ( 0.5611870653623828309, 0.8276889981568903432, 1.520440023423472778E-16 ) ) ;
#26948=EDGE_LOOP ( 'NONE', ( #18305, #15160, #32435, #22395 ) ) ;
#26960=VERTEX_POINT ( 'NONE', #27457 ) ;
#26971=ORIENTED_EDGE ( 'NONE', *, *, #23435, .T. ) ;
#26974=DIRECTION ( 'NONE',  ( 0.000000000000000000, -1.000000000000000000, -1.541976423090495633E-16 ) ) ;
#26986=DIRECTION ( 'NONE',  ( 0.000000000000000000, -1.000000000000000000, -1.836970198721029688E-16 ) ) ;
#27001=ADVANCED_FACE ( 'NONE', ( #22298 ), #20334, .F. ) ;
#27009=LINE ( 'NONE', #35033, #24786 ) ;
#27016=DIRECTION ( 'NONE',  ( -0.9635499925192230197, 0.2675283385292207550, 0.000000000000000000 ) ) ;
#27027=LINE ( 'NONE', #11364, #12160 ) ;
#27033=EDGE_CURVE ( 'NONE', #10097, #9979, #27541, .T. ) ;
#27034=LINE ( 'NONE', #13349, #29227 ) ;
#27037=ORIENTED_EDGE ( 'NONE', *, *, #18854, .F. ) ;
#27041=CARTESIAN_POINT ( 'NONE',  ( 0.000000000000000000, -44.99999999999995737, -36.68877005347594888 ) ) ;
#27045=EDGE_LOOP ( 'NONE', ( #10292, #9747, #30960, #646 ) ) ;
#27046=CARTESIAN_POINT ( 'NONE',  ( 17.88561705399012780, -27.19023860642123935, 68.31122994652405112 ) ) ;
#27049=VERTEX_POINT ( 'NONE', #19642 ) ;
#27056=PLANE ( 'NONE',  #13765 ) ;
#27062=VECTOR ( 'NONE', #10612, 1000.000000000000000 ) ;
#27072=DIRECTION ( 'NONE',  ( 0.2149704402110236556, -0.9766205557100866574, -0.000000000000000000 ) ) ;
#27086=DIRECTION ( 'NONE',  ( -0.05413890858541756113, 0.9985334138511239299, 1.834276123671687812E-16 ) ) ;
#27087=DIRECTION ( 'NONE',  ( 0.000000000000000000, 0.000000000000000000, -1.000000000000000000 ) ) ;
#27090=CARTESIAN_POINT ( 'NONE',  ( 3.235562306570555532E-30, -1.691831803474591833, -67.50000000000000000 ) ) ;
#27091=LINE ( 'NONE', #24581, #20898 ) ;
#27094=VECTOR ( 'NONE', #9632, 1000.000000000000000 ) ;
#27100=ORIENTED_EDGE ( 'NONE', *, *, #29181, .F. ) ;
#27107=EDGE_LOOP ( 'NONE', ( #17401, #31210, #6067, #23255 ) ) ;
#27108=EDGE_CURVE ( 'NONE', #1533, #32452, #25311, .T. ) ;
#27111=ORIENTED_EDGE ( 'NONE', *, *, #33619, .T. ) ;
#27113=EDGE_CURVE ( 'NONE', #34772, #15054, #25125, .T. ) ;
#27118=FACE_OUTER_BOUND ( 'NONE', #5469, .T. ) ;
#27129=VECTOR ( 'NONE', #17969, 1000.000000000000000 ) ;
#27131=CARTESIAN_POINT ( 'NONE',  ( 30.69344702212033837, -10.82204614554913036, 68.31122994652405112 ) ) ;
#27141=LINE ( 'NONE', #2927, #7434 ) ;
#27143=VECTOR ( 'NONE', #13679, 1000.000000000000114 ) ;
#27145=ORIENTED_EDGE ( 'NONE', *, *, #11367, .T. ) ;
#27146=APPLICATION_CONTEXT ( 'automotive_design' ) ;
#27147=DIRECTION ( 'NONE',  ( 1.997825486195704824E-17, 0.000000000000000000, -1.000000000000000000 ) ) ;
#27151=ORIENTED_EDGE ( 'NONE', *, *, #12447, .F. ) ;
#27152=LINE ( 'NONE', #2769, #8390 ) ;
#27155=ORIENTED_EDGE ( 'NONE', *, *, #28013, .F. ) ;
#27161=CARTESIAN_POINT ( 'NONE',  ( -45.00000000000000000, -4.831299144296466785, -15.81122994652406355 ) ) ;
#27163=ORIENTED_EDGE ( 'NONE', *, *, #19869, .F. ) ;
#27164=EDGE_CURVE ( 'NONE', #16061, #25913, #4807, .T. ) ;
#27168=CARTESIAN_POINT ( 'NONE',  ( 22.89764159710611224, 13.56412600238610544, -87.50000000000000000 ) ) ;
#27172=DIRECTION ( 'NONE',  ( 0.000000000000000000, 1.836970198721029441E-16, -1.000000000000000000 ) ) ;
#27173=LINE ( 'NONE', #19008, #25631 ) ;
#27184=ORIENTED_EDGE ( 'NONE', *, *, #25091, .F. ) ;
#27189=EDGE_CURVE ( 'NONE', #23058, #20852, #2153, .T. ) ;
#27201=ORIENTED_EDGE ( 'NONE', *, *, #7415, .T. ) ;
#27216=VERTEX_POINT ( 'NONE', #4984 ) ;
#27226=DIRECTION ( 'NONE',  ( -0.4198891015602635446, -0.9075754196709575616, -1.667188999027280528E-16 ) ) ;
#27230=CARTESIAN_POINT ( 'NONE',  ( 0.000000000000000000, 0.000000000000000000, 87.50000000000000000 ) ) ;
#27232=EDGE_CURVE ( 'NONE', #8590, #4316, #29389, .T. ) ;
#27240=CARTESIAN_POINT ( 'NONE',  ( 5.021133111224473033, 6.201984591278720593, -87.50000000000000000 ) ) ;
#27242=ORIENTED_EDGE ( 'NONE', *, *, #30577, .F. ) ;
#27248=CARTESIAN_POINT ( 'NONE',  ( 36.10877985260813716, 11.38239727801118306, 49.43553178847298568 ) ) ;
#27249=CARTESIAN_POINT ( 'NONE',  ( -2.216215597024039141, -32.46987467335850397, -36.68877005347593467 ) ) ;
#27250=AXIS2_PLACEMENT_3D ( 'NONE', #23370, #1829, #15028 ) ;
#27256=DIRECTION ( 'NONE',  ( 0.000000000000000000, 1.000000000000000000, 0.000000000000000000 ) ) ;
#27263=DIRECTION ( 'NONE',  ( 0.9985334138511239299, -0.05413890858541753337, 0.000000000000000000 ) ) ;
#27264=DIRECTION ( 'NONE',  ( 0.000000000000000000, 1.836970198721029441E-16, -1.000000000000000000 ) ) ;
#27268=EDGE_CURVE ( 'NONE', #33289, #20006, #15170, .T. ) ;
#27272=CARTESIAN_POINT ( 'NONE',  ( 0.000000000000000000, -32.54542015209055705, 49.43553178847298568 ) ) ;
#27275=VERTEX_POINT ( 'NONE', #26011 ) ;
#27280=DIRECTION ( 'NONE',  ( 0.3701381553399132329, 0.9289767198167918627, -0.000000000000000000 ) ) ;
#27284=ORIENTED_EDGE ( 'NONE', *, *, #33236, .T. ) ;
#27285=ORIENTED_EDGE ( 'NONE', *, *, #19546, .T. ) ;
#27297=DIRECTION ( 'NONE',  ( 0.000000000000000000, -1.836970198721029934E-16, 1.000000000000000000 ) ) ;
#27298=CARTESIAN_POINT ( 'NONE',  ( -29.34345171400087793, 14.07715221144534823, 68.31122994652405112 ) ) ;
#27307=ADVANCED_FACE ( 'NONE', ( #32392 ), #371, .T. ) ;
#27309=CARTESIAN_POINT ( 'NONE',  ( -1.307386931792819285, 37.83772838912469894, 68.31122994652405112 ) ) ;
#27311=EDGE_CURVE ( 'NONE', #31132, #29028, #8012, .T. ) ;
#27315=ORIENTED_EDGE ( 'NONE', *, *, #2961, .T. ) ;
#27317=CARTESIAN_POINT ( 'NONE',  ( -35.00000000000000000, 0.5883377166429079042, -15.81122994652406355 ) ) ;
#27321=AXIS2_PLACEMENT_3D ( 'NONE', #5217, #26946, #7720 ) ;
#27327=ORIENTED_EDGE ( 'NONE', *, *, #32984, .F. ) ;
#27333=ORIENTED_EDGE ( 'NONE', *, *, #9872, .F. ) ;
#27337=DIRECTION ( 'NONE',  ( 1.000000000000000000, -0.000000000000000000, -0.000000000000000000 ) ) ;
#27340=DIRECTION ( 'NONE',  ( 0.9766205557100871015, 0.2149704402110223789, 0.000000000000000000 ) ) ;
#27342=FACE_OUTER_BOUND ( 'NONE', #6043, .T. ) ;
#27343=CARTESIAN_POINT ( 'NONE',  ( 0.000000000000000000, 3.524919873834583163E-15, 68.31122994652405112 ) ) ;
#27350=ORIENTED_EDGE ( 'NONE', *, *, #27232, .T. ) ;
#27358=VECTOR ( 'NONE', #10689, 1000.000000000000000 ) ;
#27360=EDGE_CURVE ( 'NONE', #22752, #28240, #8228, .T. ) ;
#27364=CIRCLE ( 'NONE', #12050, 32.54542015209055705 ) ;
#27366=DIRECTION ( 'NONE',  ( 0.9985334138511239299, 0.05413890858541774848, 0.000000000000000000 ) ) ;
#27367=ORIENTED_EDGE ( 'NONE', *, *, #29030, .F. ) ;
#27370=DIRECTION ( 'NONE',  ( -0.5155538571770218459, 0.8568571761675891629, 0.000000000000000000 ) ) ;
#27374=VECTOR ( 'NONE', #14049, 1000.000000000000000 ) ;
#27383=FACE_OUTER_BOUND ( 'NONE', #3227, .T. ) ;
#27390=ORIENTED_EDGE ( 'NONE', *, *, #19548, .T. ) ;
#27393=AXIS2_PLACEMENT_3D ( 'NONE', #21339, #29523, #5115 ) ;
#27399=ORIENTED_EDGE ( 'NONE', *, *, #31324, .F. ) ;
#27401=PLANE ( 'NONE',  #22908 ) ;
#27404=CARTESIAN_POINT ( 'NONE',  ( 10.17231796313409298, 8.346743312457579833, -77.50000000000000000 ) ) ;
#27426=EDGE_CURVE ( 'NONE', #26369, #9416, #24207, .T. ) ;
#27432=ORIENTED_EDGE ( 'NONE', *, *, #9605, .T. ) ;
#27434=DIRECTION ( 'NONE',  ( -0.5611870653623824978, -0.8276889981568904542, -1.520440023423473517E-16 ) ) ;
#27443=PLANE ( 'NONE',  #25352 ) ;
#27454=ADVANCED_FACE ( 'NONE', ( #27587 ), #22613, .T. ) ;
#27457=CARTESIAN_POINT ( 'NONE',  ( 5.021133111224162171, -21.54630831098063837, -67.50000000000000000 ) ) ;
#27460=EDGE_LOOP ( 'NONE', ( #17412, #346, #33345, #32108 ) ) ;
#27469=LINE ( 'NONE', #24963, #30970 ) ;
#27477=DIRECTION ( 'NONE',  ( 3.697785493223492838E-32, 1.934419779023891545E-16, -1.000000000000000000 ) ) ;
#27481=VERTEX_POINT ( 'NONE', #12115 ) ;
#27485=DIRECTION ( 'NONE',  ( 0.000000000000000000, 1.836970198721029441E-16, -1.000000000000000000 ) ) ;
#27487=CARTESIAN_POINT ( 'NONE',  ( -5.021133111225196011, -21.54630831098063837, -67.50000000000000000 ) ) ;
#27494=ORIENTED_EDGE ( 'NONE', *, *, #29299, .F. ) ;
#27497=ORIENTED_EDGE ( 'NONE', *, *, #28341, .T. ) ;
#27499=CYLINDRICAL_SURFACE ( 'NONE', #20543, 10.00000000000000000 ) ;
#27500=EDGE_LOOP ( 'NONE', ( #31705, #6415, #30001, #30131 ) ) ;
#27504=DIRECTION ( 'NONE',  ( 0.000000000000000000, 1.000000000000000000, 0.000000000000000000 ) ) ;
#27506=ORIENTED_EDGE ( 'NONE', *, *, #28224, .T. ) ;
#27508=LINE ( 'NONE', #815, #15027 ) ;
#27535=ORIENTED_EDGE ( 'NONE', *, *, #20451, .T. ) ;
#27540=ORIENTED_EDGE ( 'NONE', *, *, #32921, .T. ) ;
#27541=CIRCLE ( 'NONE', #3656, 32.54542015209054995 ) ;
#27546=ORIENTED_EDGE ( 'NONE', *, *, #2651, .F. ) ;
#27548=DIRECTION ( 'NONE',  ( 0.9868265225415261410, -0.1617819965527648174, 0.000000000000000000 ) ) ;
#27553=VECTOR ( 'NONE', #16421, 1000.000000000000114 ) ;
#27554=CARTESIAN_POINT ( 'NONE',  ( 5.021133111224679091, 24.02303923978505296, -87.50000000000000000 ) ) ;
#27556=ORIENTED_EDGE ( 'NONE', *, *, #15615, .T. ) ;
#27557=ORIENTED_EDGE ( 'NONE', *, *, #28844, .F. ) ;
#27560=LINE ( 'NONE', #870, #24907 ) ;
#27562=EDGE_CURVE ( 'NONE', #9321, #16675, #8720, .T. ) ;
#27567=VERTEX_POINT ( 'NONE', #30441 ) ;
#27573=CYLINDRICAL_SURFACE ( 'NONE', #2186, 2.033421858999711951 ) ;
#27574=EDGE_CURVE ( 'NONE', #15307, #11484, #3682, .T. ) ;
#27575=DIRECTION ( 'NONE',  ( -1.000000000000000000, 0.000000000000000000, 0.000000000000000000 ) ) ;
#27578=CARTESIAN_POINT ( 'NONE',  ( -20.02113311122509032, -11.61907005722761532, -67.50000000000000000 ) ) ;
#27587=FACE_OUTER_BOUND ( 'NONE', #32883, .T. ) ;
#27588=DIRECTION ( 'NONE',  ( 0.000000000000000000, 1.836970198721029441E-16, -1.000000000000000000 ) ) ;
#27589=AXIS2_PLACEMENT_3D ( 'NONE', #31425, #14900, #7028 ) ;
#27590=ORIENTED_EDGE ( 'NONE', *, *, #14279, .F. ) ;
#27591=AXIS2_PLACEMENT_3D ( 'NONE', #28072, #25217, #30398 ) ;
#27593=ORIENTED_EDGE ( 'NONE', *, *, #13570, .T. ) ;
#27596=LINE ( 'NONE', #11774, #19605 ) ;
#27597=DIRECTION ( 'NONE',  ( -0.000000000000000000, 1.836970198721029688E-16, -1.000000000000000000 ) ) ;
#27604=ORIENTED_EDGE ( 'NONE', *, *, #9970, .F. ) ;
#27606=EDGE_CURVE ( 'NONE', #22562, #2115, #20983, .T. ) ;
#27607=EDGE_CURVE ( 'NONE', #17615, #8779, #19638, .T. ) ;
#27612=DIRECTION ( 'NONE',  ( 0.000000000000000000, 1.836970198721029934E-16, -1.000000000000000000 ) ) ;
#27623=DIRECTION ( 'NONE',  ( -0.8835120444460228262, 0.4684084406997903183, 0.000000000000000000 ) ) ;
#27628=VERTEX_POINT ( 'NONE', #31999 ) ;
#27629=DIRECTION ( 'NONE',  ( 0.9766205557100864354, -0.2149704402110247659, 0.000000000000000000 ) ) ;
#27636=VECTOR ( 'NONE', #32171, 1000.000000000000000 ) ;
#27639=ORIENTED_EDGE ( 'NONE', *, *, #11403, .F. ) ;
#27652=DIRECTION ( 'NONE',  ( -0.3193015301359781177, 0.9476531711828031224, 1.740810634186287624E-16 ) ) ;
#27656=ORIENTED_EDGE ( 'NONE', *, *, #31895, .F. ) ;
#27657=VECTOR ( 'NONE', #3751, 1000.000000000000114 ) ;
#27664=CYLINDRICAL_SURFACE ( 'NONE', #10372, 10.00000000000000000 ) ;
#27666=CYLINDRICAL_SURFACE ( 'NONE', #6438, 2.033421858999711507 ) ;
#27683=ORIENTED_EDGE ( 'NONE', *, *, #12675, .T. ) ;
#27685=CARTESIAN_POINT ( 'NONE',  ( -12.91951790633627439, -3.497874208484963443, -14.98024667272714083 ) ) ;
#27691=ORIENTED_EDGE ( 'NONE', *, *, #9991, .F. ) ;
#27695=CARTESIAN_POINT ( 'NONE',  ( -23.78520691327551262, 22.21414650552148373, 68.31122994652405112 ) ) ;
#27697=LINE ( 'NONE', #3314, #8624 ) ;
#27698=LINE ( 'NONE', #19186, #20215 ) ;
#27701=DIRECTION ( 'NONE',  ( -0.000000000000000000, 1.836970198721029934E-16, -1.000000000000000000 ) ) ;
#27706=CARTESIAN_POINT ( 'NONE',  ( -20.72055270933793736, 25.09707290294328885, 68.31122994652405112 ) ) ;
#27711=EDGE_LOOP ( 'NONE', ( #6991, #27540, #2724, #28461 ) ) ;
#27713=LINE ( 'NONE', #20077, #25611 ) ;
#27714=ADVANCED_FACE ( 'NONE', ( #7435 ), #4064, .F. ) ;
#27715=AXIS2_PLACEMENT_3D ( 'NONE', #19351, #5789, #9015 ) ;
#27719=CARTESIAN_POINT ( 'NONE',  ( 5.713835024271042506, 32.03991982186466458, 68.31122994652405112 ) ) ;
#27728=PLANE ( 'NONE',  #3618 ) ;
#27731=FACE_OUTER_BOUND ( 'NONE', #17496, .T. ) ;
#27734=VERTEX_POINT ( 'NONE', #18682 ) ;
#27739=VECTOR ( 'NONE', #6273, 1000.000000000000000 ) ;
#27740=CARTESIAN_POINT ( 'NONE',  ( 22.89764159710615132, -1.579009122040562207, -77.50000000000000000 ) ) ;
#27757=CARTESIAN_POINT ( 'NONE',  ( 30.69344702212033127, -10.82204614554912325, 49.43553178847298568 ) ) ;
#27770=EDGE_CURVE ( 'NONE', #31774, #2524, #2278, .T. ) ;
#27777=DIRECTION ( 'NONE',  ( 1.000000000000000000, 0.000000000000000000, 0.000000000000000000 ) ) ;
#27782=EDGE_LOOP ( 'NONE', ( #32971, #29438, #3296, #9082 ) ) ;
#27784=FACE_OUTER_BOUND ( 'NONE', #5401, .T. ) ;
#27785=DIRECTION ( 'NONE',  ( 0.000000000000000000, 1.836970198721029441E-16, -1.000000000000000000 ) ) ;
#27789=AXIS2_PLACEMENT_3D ( 'NONE', #27343, #7954, #16166 ) ;
#27790=DIRECTION ( 'NONE',  ( -0.2675283385292216987, 0.9635499925192227977, -0.000000000000000000 ) ) ;
#27795=CARTESIAN_POINT ( 'NONE',  ( 60.00000000000000000, -33.69708579775584667, 49.43553178847298568 ) ) ;
#27796=CARTESIAN_POINT ( 'NONE',  ( 13.32059394339353986, -35.43959265050634144, 68.31122994652405112 ) ) ;
#27800=DIRECTION ( 'NONE',  ( 3.697785493223492838E-32, 1.934419779023891545E-16, -1.000000000000000000 ) ) ;
#27803=( NAMED_UNIT ( * ) SI_UNIT ( $, .STERADIAN. ) SOLID_ANGLE_UNIT ( ) );
#27805=CIRCLE ( 'NONE', #32350, 2.033421858999710619 ) ;
#27812=ORIENTED_EDGE ( 'NONE', *, *, #5390, .F. ) ;
#27817=EDGE_CURVE ( 'NONE', #9350, #8552, #10482, .T. ) ;
#27818=VECTOR ( 'NONE', #18184, 1000.000000000000000 ) ;
#27821=CARTESIAN_POINT ( 'NONE',  ( 13.32059394339353986, -35.43959265050632013, -36.68877005347593467 ) ) ;
#27831=VERTEX_POINT ( 'NONE', #10659 ) ;
#27835=CARTESIAN_POINT ( 'NONE',  ( -15.64512930492131382, -28.53829535743846435, 68.31122994652405112 ) ) ;
#27840=AXIS2_PLACEMENT_3D ( 'NONE', #3942, #7137, #19516 ) ;
#27842=DIRECTION ( 'NONE',  ( 0.9635499925192227977, -0.2675283385292215321, -4.914415851915309929E-17 ) ) ;
#27844=ORIENTED_EDGE ( 'NONE', *, *, #2027, .T. ) ;
#27845=CARTESIAN_POINT ( 'NONE',  ( 0.000000000000000000, 3.670182593897650235E-31, 87.50000000000000000 ) ) ;
#27846=CARTESIAN_POINT ( 'NONE',  ( 5.390701026406702567, -37.47456861236020131, 68.31122994652405112 ) ) ;
#27848=ORIENTED_EDGE ( 'NONE', *, *, #16583, .F. ) ;
#27856=FACE_OUTER_BOUND ( 'NONE', #631, .T. ) ;
#27859=LINE ( 'NONE', #996, #33195 ) ;
#27862=CARTESIAN_POINT ( 'NONE',  ( -35.00000000000000000, -46.95407462254104303, -36.69637551990492597 ) ) ;
#27864=EDGE_LOOP ( 'NONE', ( #5653, #28350, #15829, #12278, #10038, #10723, #26463, #917, #24692 ) ) ;
#27865=VERTEX_POINT ( 'NONE', #141 ) ;
#27867=CARTESIAN_POINT ( 'NONE',  ( 8.927936315454026328, -31.29690601358700519, 68.31122994652405112 ) ) ;
#27868=DIRECTION ( 'NONE',  ( 0.000000000000000000, 0.5288966977476834419, 0.8486862100397269959 ) ) ;
#27869=DIRECTION ( 'NONE',  ( -0.000000000000000000, -0.000000000000000000, -1.000000000000000000 ) ) ;
#27871=ADVANCED_FACE ( 'NONE', ( #10999 ), #21851, .F. ) ;
#27872=EDGE_CURVE ( 'NONE', #19171, #21431, #29305, .T. ) ;
#27881=EDGE_LOOP ( 'NONE', ( #24643, #8244, #12178, #30680 ) ) ;
#27882=EDGE_CURVE ( 'NONE', #27945, #15892, #17429, .T. ) ;
#27887=CARTESIAN_POINT ( 'NONE',  ( -35.71762877834949990, -12.58147180936567011, 68.31122994652405112 ) ) ;
#27890=DIRECTION ( 'NONE',  ( -1.000000000000000000, -0.000000000000000000, -0.000000000000000000 ) ) ;
#27894=VECTOR ( 'NONE', #23204, 1000.000000000000000 ) ;
#27896=VECTOR ( 'NONE', #25747, 1000.000000000000000 ) ;
#27911=EDGE_CURVE ( 'NONE', #28782, #7203, #28158, .T. ) ;
#27912=LINE ( 'NONE', #33431, #24514 ) ;
#27917=CARTESIAN_POINT ( 'NONE',  ( -36.04853892210773836, 11.59936550071287797, -29.04209251724896745 ) ) ;
#27921=ORIENTED_EDGE ( 'NONE', *, *, #9919, .F. ) ;
#27924=DIRECTION ( 'NONE',  ( 0.000000000000000000, 1.000000000000000000, 1.934419779023891545E-16 ) ) ;
#27931=VECTOR ( 'NONE', #25530, 1000.000000000000000 ) ;
#27936=CARTESIAN_POINT ( 'NONE',  ( 5.390701026406702567, -37.47456861236018000, -36.68877005347593467 ) ) ;
#27940=ORIENTED_EDGE ( 'NONE', *, *, #232, .T. ) ;
#27941=VECTOR ( 'NONE', #8872, 1000.000000000000114 ) ;
#27945=VERTEX_POINT ( 'NONE', #11360 ) ;
#27953=CARTESIAN_POINT ( 'NONE',  ( -5.021133111224886036, 8.235406450278427215, -67.50000000000000000 ) ) ;
#27957=EDGE_CURVE ( 'NONE', #20902, #5869, #22742, .T. ) ;
#27959=CARTESIAN_POINT ( 'NONE',  ( 31.83311414508813897, -6.771795677801486057, 68.31122994652405112 ) ) ;
#27963=EDGE_CURVE ( 'NONE', #3468, #3784, #852, .T. ) ;
#27967=ORIENTED_EDGE ( 'NONE', *, *, #34834, .T. ) ;
#27973=DIRECTION ( 'NONE',  ( -0.000000000000000000, 1.836970198721029688E-16, -1.000000000000000000 ) ) ;
#27976=CIRCLE ( 'NONE', #25687, 44.99999999999997868 ) ;
#27987=ORIENTED_EDGE ( 'NONE', *, *, #25388, .F. ) ;
#27997=CARTESIAN_POINT ( 'NONE',  ( 15.04122381213380244, 28.86114964982165887, 68.31122994652405112 ) ) ;
#27999=DIRECTION ( 'NONE',  ( 0.000000000000000000, 1.000000000000000000, 1.836970198721029688E-16 ) ) ;
#28002=ORIENTED_EDGE ( 'NONE', *, *, #4343, .T. ) ;
#28003=VECTOR ( 'NONE', #15782, 1000.000000000000000 ) ;
#28013=EDGE_CURVE ( 'NONE', #19775, #2856, #28949, .T. ) ;
#28014=EDGE_CURVE ( 'NONE', #10479, #27216, #23612, .T. ) ;
#28016=( BOUNDED_CURVE ( )  B_SPLINE_CURVE ( 3, ( #16903, #24181, #35059, #21527 ),
 .UNSPECIFIED., .F., .F. ) 
 B_SPLINE_CURVE_WITH_KNOTS ( ( 4, 4 ),
 ( 4.340081192300065283, 4.340194262747512965 ),
 .UNSPECIFIED. ) 
 CURVE ( )  GEOMETRIC_REPRESENTATION_ITEM ( )  RATIONAL_B_SPLINE_CURVE ( ( 1.000000000000000000, 0.9999999989345893514, 0.9999999989345893514, 1.000000000000000000 ) ) 
 REPRESENTATION_ITEM ( '' )  );
#28018=DIRECTION ( 'NONE',  ( -0.6051742151937663516, -0.7960930657056428661, -1.462399237109728568E-16 ) ) ;
#28021=ADVANCED_FACE ( 'NONE', ( #22916 ), #20425, .F. ) ;
#28025=VERTEX_POINT ( 'NONE', #34289 ) ;
#28027=LINE ( 'NONE', #14163, #158 ) ;
#28030=VECTOR ( 'NONE', #4193, 1000.000000000000000 ) ;
#28031=VERTEX_POINT ( 'NONE', #23101 ) ;
#28038=LINE ( 'NONE', #23752, #3713 ) ;
#28048=LINE ( 'NONE', #33211, #7116 ) ;
#28063=DIRECTION ( 'NONE',  ( -0.1081190184239420177, -0.9941379571543595972, 0.000000000000000000 ) ) ;
#28065=CARTESIAN_POINT ( 'NONE',  ( 32.81769769215652133, 18.87860345536237006, 68.31122994652405112 ) ) ;
#28069=AXIS2_PLACEMENT_3D ( 'NONE', #11193, #5644, #5299 ) ;
#28072=CARTESIAN_POINT ( 'NONE',  ( 10.17231796313409298, 6.310691531022071921, -87.50000000000000000 ) ) ;
#28082=CARTESIAN_POINT ( 'NONE',  ( -9.978866888775733912, -13.65249191622732816, -67.50000000000000000 ) ) ;
#28086=CARTESIAN_POINT ( 'NONE',  ( 31.83311414508813897, -6.771795677801482505, 49.43553178847298568 ) ) ;
#28087=CARTESIAN_POINT ( 'NONE',  ( 3.235562306570555532E-30, 1.325223266901699007E-14, -67.50000000000000000 ) ) ;
#28090=EDGE_LOOP ( 'NONE', ( #18949, #24236, #18675, #34731 ) ) ;
#28091=VERTEX_POINT ( 'NONE', #9395 ) ;
#28095=DIRECTION ( 'NONE',  ( 0.9868265225415266961, 0.1617819965527614590, 2.971887063570111902E-17 ) ) ;
#28099=DIRECTION ( 'NONE',  ( 0.000000000000000000, 1.836970198721029441E-16, -1.000000000000000000 ) ) ;
#28100=DIRECTION ( 'NONE',  ( -0.000000000000000000, 1.836970198721029934E-16, -1.000000000000000000 ) ) ;
#28108=LINE ( 'NONE', #19404, #28274 ) ;
#28111=ORIENTED_EDGE ( 'NONE', *, *, #35020, .T. ) ;
#28112=DIRECTION ( 'NONE',  ( 0.2675283385292215321, 0.9635499925192227977, 0.000000000000000000 ) ) ;
#28120=EDGE_CURVE ( 'NONE', #25488, #8590, #6702, .T. ) ;
#28139=FACE_OUTER_BOUND ( 'NONE', #13226, .T. ) ;
#28140=EDGE_LOOP ( 'NONE', ( #3608, #8320, #32136, #6262 ) ) ;
#28141=ORIENTED_EDGE ( 'NONE', *, *, #19989, .F. ) ;
#28142=LINE ( 'NONE', #14637, #11751 ) ;
#28144=DIRECTION ( 'NONE',  ( 1.000000000000000000, 0.000000000000000000, 0.000000000000000000 ) ) ;
#28145=CARTESIAN_POINT ( 'NONE',  ( -27.76765758629847269, -16.97532223688794417, 68.31122994652405112 ) ) ;
#28149=DIRECTION ( 'NONE',  ( 0.000000000000000000, 1.836970198721029688E-16, -1.000000000000000000 ) ) ;
#28155=LINE ( 'NONE', #3409, #24026 ) ;
#28156=DIRECTION ( 'NONE',  ( 0.000000000000000000, 1.836970198721029441E-16, -1.000000000000000000 ) ) ;
#28157=LINE ( 'NONE', #14820, #6580 ) ;
#28158=CIRCLE ( 'NONE', #27591, 2.036051781435508801 ) ;
#28161=AXIS2_PLACEMENT_3D ( 'NONE', #20046, #14359, #6307 ) ;
#28162=ORIENTED_EDGE ( 'NONE', *, *, #8436, .F. ) ;
#28164=CARTESIAN_POINT ( 'NONE',  ( 60.00000000000000000, 33.69708579775584667, 49.43553178847298568 ) ) ;
#28167=ADVANCED_FACE ( 'NONE', ( #20596 ), #2415, .F. ) ;
#28169=EDGE_LOOP ( 'NONE', ( #24996, #5697, #21097, #9827, #20640, #30861, #32346, #24400 ) ) ;
#28172=CIRCLE ( 'NONE', #3161, 32.54542015209054995 ) ;
#28173=VERTEX_POINT ( 'NONE', #8285 ) ;
#28180=EDGE_LOOP ( 'NONE', ( #2114, #24039, #32355, #4389, #22416, #7454, #25593, #16171 ) ) ;
#28182=PLANE ( 'NONE',  #29643 ) ;
#28183=ORIENTED_EDGE ( 'NONE', *, *, #22982, .F. ) ;
#28188=VECTOR ( 'NONE', #31519, 1000.000000000000000 ) ;
#28198=CARTESIAN_POINT ( 'NONE',  ( -37.85301660235036536, 0.7430237821112765095, -36.68877005347593467 ) ) ;
#28203=CARTESIAN_POINT ( 'NONE',  ( 5.021133111224162171, -21.54630831098063837, -67.50000000000000000 ) ) ;
#28204=VERTEX_POINT ( 'NONE', #27317 ) ;
#28205=DIRECTION ( 'NONE',  ( -0.000000000000000000, -1.836970198721029688E-16, 1.000000000000000000 ) ) ;
#28210=ORIENTED_EDGE ( 'NONE', *, *, #29134, .F. ) ;
#28215=ORIENTED_EDGE ( 'NONE', *, *, #7303, .F. ) ;
#28220=VERTEX_POINT ( 'NONE', #99 ) ;
#28224=EDGE_CURVE ( 'NONE', #1565, #4220, #26802, .T. ) ;
#28230=ORIENTED_EDGE ( 'NONE', *, *, #19838, .F. ) ;
#28240=VERTEX_POINT ( 'NONE', #21292 ) ;
#28243=CARTESIAN_POINT ( 'NONE',  ( 21.85761591200894216, 30.91355005303806180, 49.43553178847298568 ) ) ;
#28248=DIRECTION ( 'NONE',  ( 0.000000000000000000, 1.836970198721029688E-16, -1.000000000000000000 ) ) ;
#28252=ORIENTED_EDGE ( 'NONE', *, *, #5632, .F. ) ;
#28254=DIRECTION ( 'NONE',  ( 0.000000000000000000, 1.836970198721029441E-16, -1.000000000000000000 ) ) ;
#28256=EDGE_CURVE ( 'NONE', #4555, #4220, #5427, .T. ) ;
#28259=ADVANCED_FACE ( 'NONE', ( #18463 ), #29308, .T. ) ;
#28265=FACE_OUTER_BOUND ( 'NONE', #3250, .T. ) ;
#28274=VECTOR ( 'NONE', #17460, 1000.000000000000000 ) ;
#28289=ORIENTED_EDGE ( 'NONE', *, *, #12272, .T. ) ;
#28292=ADVANCED_FACE ( 'NONE', ( #3113 ), #3635, .F. ) ;
#28296=CARTESIAN_POINT ( 'NONE',  ( -36.80830595996284416, 8.862931941313773265, 68.31122994652405112 ) ) ;
#28298=DIRECTION ( 'NONE',  ( 0.000000000000000000, 1.836970198721029441E-16, -1.000000000000000000 ) ) ;
#28302=ORIENTED_EDGE ( 'NONE', *, *, #23338, .T. ) ;
#28303=VECTOR ( 'NONE', #10838, 1000.000000000000000 ) ;
#28306=EDGE_CURVE ( 'NONE', #31368, #32385, #11491, .T. ) ;
#28315=ORIENTED_EDGE ( 'NONE', *, *, #3893, .T. ) ;
#28321=ORIENTED_EDGE ( 'NONE', *, *, #15963, .T. ) ;
#28325=CARTESIAN_POINT ( 'NONE',  ( -9.978866888775527855, 8.235406450278427215, -67.50000000000000000 ) ) ;
#28330=EDGE_CURVE ( 'NONE', #23654, #13441, #6483, .T. ) ;
#28331=CARTESIAN_POINT ( 'NONE',  ( -15.64512930492131382, -28.53829535743844659, -36.68877005347593467 ) ) ;
#28334=DIRECTION ( 'NONE',  ( 1.000000000000000000, 0.000000000000000000, -0.000000000000000000 ) ) ;
#28336=DIRECTION ( 'NONE',  ( -0.8568571761675891629, -0.5155538571770218459, -9.470570714698669088E-17 ) ) ;
#28341=EDGE_CURVE ( 'NONE', #30722, #20533, #27364, .T. ) ;
#28342=LINE ( 'NONE', #9644, #2890 ) ;
#28349=ORIENTED_EDGE ( 'NONE', *, *, #10937, .T. ) ;
#28350=ORIENTED_EDGE ( 'NONE', *, *, #17593, .T. ) ;
#28361=CARTESIAN_POINT ( 'NONE',  ( 26.97014235612466493, -26.57093094961043533, 49.43553178847298568 ) ) ;
#28362=ORIENTED_EDGE ( 'NONE', *, *, #34586, .T. ) ;
#28363=ORIENTED_EDGE ( 'NONE', *, *, #494, .F. ) ;
#28364=DIRECTION ( 'NONE',  ( 0.2149704402110236556, 0.9766205557100866574, 0.000000000000000000 ) ) ;
#28365=CARTESIAN_POINT ( 'NONE',  ( -37.85301660235036536, 0.7430237821112573027, 68.31122994652405112 ) ) ;
#28366=EDGE_CURVE ( 'NONE', #3550, #33018, #11148, .T. ) ;
#28371=EDGE_CURVE ( 'NONE', #14545, #29231, #9163, .T. ) ;
#28373=ADVANCED_FACE ( 'NONE', ( #33192 ), #13809, .T. ) ;
#28375=CARTESIAN_POINT ( 'NONE',  ( -30.76765767668600660, -10.60922306139170779, -36.68877005347593467 ) ) ;
#28377=CARTESIAN_POINT ( 'NONE',  ( 0.000000000000000000, 2.296212748401288367E-15, 47.49999999999999289 ) ) ;
#28395=VERTEX_POINT ( 'NONE', #19686 ) ;
#28397=ORIENTED_EDGE ( 'NONE', *, *, #12592, .F. ) ;
#28399=CARTESIAN_POINT ( 'NONE',  ( -35.00000000000000000, -14.38258422898374533, 21.76353962326706082 ) ) ;
#28403=DIRECTION ( 'NONE',  ( -1.000000000000000000, 6.792721752314501023E-48, -3.697785493223492838E-32 ) ) ;
#28410=ADVANCED_FACE ( 'NONE', ( #33370 ), #27499, .F. ) ;
#28414=DIRECTION ( 'NONE',  ( 0.000000000000000000, 1.000000000000000000, 0.000000000000000000 ) ) ;
#28423=LINE ( 'NONE', #1022, #6419 ) ;
#28427=EDGE_CURVE ( 'NONE', #12281, #27481, #31062, .T. ) ;
#28437=DIRECTION ( 'NONE',  ( -0.9289767198167909745, 0.3701381553399156199, -0.000000000000000000 ) ) ;
#28441=ORIENTED_EDGE ( 'NONE', *, *, #19742, .T. ) ;
#28444=LINE ( 'NONE', #31287, #20883 ) ;
#28453=EDGE_CURVE ( 'NONE', #19961, #3900, #23951, .T. ) ;
#28458=ADVANCED_FACE ( 'NONE', ( #12211 ), #23056, .T. ) ;
#28459=EDGE_CURVE ( 'NONE', #8996, #24880, #5197, .T. ) ;
#28461=ORIENTED_EDGE ( 'NONE', *, *, #18413, .T. ) ;
#28471=ORIENTED_EDGE ( 'NONE', *, *, #24499, .F. ) ;
#28473=ORIENTED_EDGE ( 'NONE', *, *, #4352, .T. ) ;
#28486=CARTESIAN_POINT ( 'NONE',  ( -37.85301660235036536, 0.7430237821112573027, 15.81122994652406355 ) ) ;
#28491=LINE ( 'NONE', #17492, #21390 ) ;
#28497=LINE ( 'NONE', #20489, #22641 ) ;
#28505=FACE_OUTER_BOUND ( 'NONE', #16992, .T. ) ;
#28515=EDGE_LOOP ( 'NONE', ( #33368, #13388, #1904, #26642 ) ) ;
#28520=EDGE_CURVE ( 'NONE', #1376, #28825, #28734, .T. ) ;
#28521=ORIENTED_EDGE ( 'NONE', *, *, #28371, .T. ) ;
#28529=EDGE_CURVE ( 'NONE', #33917, #12216, #3813, .T. ) ;
#28531=ADVANCED_FACE ( 'NONE', ( #18727 ), #30262, .F. ) ;
#28534=CARTESIAN_POINT ( 'NONE',  ( 22.89764159710611224, 17.63622956525712482, -87.50000000000000000 ) ) ;
#28536=ORIENTED_EDGE ( 'NONE', *, *, #20685, .F. ) ;
#28543=CARTESIAN_POINT ( 'NONE',  ( 3.235562306570555532E-30, -1.691831803474591833, -67.50000000000000000 ) ) ;
#28544=DIRECTION ( 'NONE',  ( 0.000000000000000000, 1.836970198721029441E-16, -1.000000000000000000 ) ) ;
#28549=LINE ( 'NONE', #20712, #32128 ) ;
#28550=CARTESIAN_POINT ( 'NONE',  ( 0.000000000000000000, 33.69708579775584667, 49.43553178847298568 ) ) ;
#28551=FACE_OUTER_BOUND ( 'NONE', #30851, .T. ) ;
#28556=ORIENTED_EDGE ( 'NONE', *, *, #21132, .F. ) ;
#28559=CARTESIAN_POINT ( 'NONE',  ( 5.021133111224162171, -25.61315202898005694, -87.50000000000000000 ) ) ;
#28563=DIRECTION ( 'NONE',  ( 0.000000000000000000, 0.000000000000000000, 1.000000000000000000 ) ) ;
#28566=AXIS2_PLACEMENT_3D ( 'NONE', #26579, #2200, #13073 ) ;
#28568=AXIS2_PLACEMENT_3D ( 'NONE', #28550, #6114, #33530 ) ;
#28569=AXIS2_PLACEMENT_3D ( 'NONE', #33900, #20380, #9519 ) ;
#28574=ORIENTED_EDGE ( 'NONE', *, *, #23478, .T. ) ;
#28578=CARTESIAN_POINT ( 'NONE',  ( -23.93921925319781963, 29.33115633223345142, 68.31122994652405112 ) ) ;
#28581=PLANE ( 'NONE',  #24754 ) ;
#28589=DIRECTION ( 'NONE',  ( 0.000000000000000000, -1.000000000000000000, -1.836970198721029934E-16 ) ) ;
#28590=CARTESIAN_POINT ( 'NONE',  ( -27.76765758629847269, -16.97532223688792286, -36.68877005347593467 ) ) ;
#28594=AXIS2_PLACEMENT_3D ( 'NONE', #26309, #21330, #24158 ) ;
#28602=CARTESIAN_POINT ( 'NONE',  ( -30.76765767668600660, -10.60922306139172555, 68.31122994652405112 ) ) ;
#28603=DIRECTION ( 'NONE',  ( 0.8835120444460227151, -0.4684084406997905403, -8.604523463949019211E-17 ) ) ;
#28604=EDGE_CURVE ( 'NONE', #32360, #18325, #5696, .T. ) ;
#28610=ORIENTED_EDGE ( 'NONE', *, *, #33829, .F. ) ;
#28615=LINE ( 'NONE', #28086, #7643 ) ;
#28626=CARTESIAN_POINT ( 'NONE',  ( -25.07182831876307105, -28.36910952062234870, 68.31122994652405112 ) ) ;
#28636=AXIS2_PLACEMENT_3D ( 'NONE', #34418, #23734, #20542 ) ;
#28641=EDGE_CURVE ( 'NONE', #29194, #1101, #13674, .T. ) ;
#28642=ORIENTED_EDGE ( 'NONE', *, *, #34671, .F. ) ;
#28643=ORIENTED_EDGE ( 'NONE', *, *, #18553, .F. ) ;
#28647=ORIENTED_EDGE ( 'NONE', *, *, #29030, .T. ) ;
#28651=EDGE_CURVE ( 'NONE', #8202, #33289, #32569, .T. ) ;
#28656=DIRECTION ( 'NONE',  ( 0.7259954919231310644, -0.6876994588534230957, -1.263283411590317421E-16 ) ) ;
#28663=VECTOR ( 'NONE', #14655, 1000.000000000000000 ) ;
#28670=DIRECTION ( 'NONE',  ( 0.9868265225415260300, 0.1617819965527648174, 0.000000000000000000 ) ) ;
#28676=PLANE ( 'NONE',  #22369 ) ;
#28677=LINE ( 'NONE', #4278, #8227 ) ;
#28678=DIRECTION ( 'NONE',  ( -0.7259954919231303982, 0.6876994588534237618, 1.263283411590318407E-16 ) ) ;
#28680=CYLINDRICAL_SURFACE ( 'NONE', #12047, 2.033421858999711951 ) ;
#28689=EDGE_CURVE ( 'NONE', #23161, #30243, #8376, .T. ) ;
#28708=LINE ( 'NONE', #18055, #8001 ) ;
#28719=EDGE_CURVE ( 'NONE', #22002, #12565, #6371, .T. ) ;
#28724=ADVANCED_FACE ( 'NONE', ( #11917 ), #23124, .F. ) ;
#28726=ORIENTED_EDGE ( 'NONE', *, *, #27562, .T. ) ;
#28732=VERTEX_POINT ( 'NONE', #33966 ) ;
#28733=CIRCLE ( 'NONE', #10550, 10.00000000000000000 ) ;
#28734=LINE ( 'NONE', #34914, #27931 ) ;
#28736=VERTEX_POINT ( 'NONE', #25955 ) ;
#28746=ORIENTED_EDGE ( 'NONE', *, *, #3412, .T. ) ;
#28757=ORIENTED_EDGE ( 'NONE', *, *, #28689, .T. ) ;
#28759=DIRECTION ( 'NONE',  ( -0.7259954919231307313, 0.6876994588534234287, 0.000000000000000000 ) ) ;
#28763=EDGE_LOOP ( 'NONE', ( #7989, #15294, #20440, #10538, #7703, #17113, #25925, #31484 ) ) ;
#28764=EDGE_CURVE ( 'NONE', #17068, #25913, #14416, .T. ) ;
#28769=LINE ( 'NONE', #20761, #25931 ) ;
#28777=ORIENTED_EDGE ( 'NONE', *, *, #1003, .T. ) ;
#28778=AXIS2_PLACEMENT_3D ( 'NONE', #16427, #14098, #27256 ) ;
#28780=ORIENTED_EDGE ( 'NONE', *, *, #33927, .F. ) ;
#28782=VERTEX_POINT ( 'NONE', #9230 ) ;
#28786=DIRECTION ( 'NONE',  ( -0.000000000000000000, 1.836970198721029688E-16, -1.000000000000000000 ) ) ;
#28787=LINE ( 'NONE', #23444, #9696 ) ;
#28791=EDGE_CURVE ( 'NONE', #29040, #6216, #31290, .T. ) ;
#28798=DIRECTION ( 'NONE',  ( 0.000000000000000000, -1.000000000000000000, 0.000000000000000000 ) ) ;
#28803=DIRECTION ( 'NONE',  ( 0.000000000000000000, 0.000000000000000000, 1.000000000000000000 ) ) ;
#28814=DIRECTION ( 'NONE',  ( -0.9868265225415261410, -0.1617819965527648174, 0.000000000000000000 ) ) ;
#28820=PLANE ( 'NONE',  #22077 ) ;
#28825=VERTEX_POINT ( 'NONE', #27917 ) ;
#28827=DIRECTION ( 'NONE',  ( 0.000000000000000000, 1.000000000000000000, -0.000000000000000000 ) ) ;
#28830=DIRECTION ( 'NONE',  ( -0.000000000000000000, 1.836970198721029934E-16, -1.000000000000000000 ) ) ;
#28833=CARTESIAN_POINT ( 'NONE',  ( 4.979875012683822710, -33.69708579775584667, 49.43553178847298568 ) ) ;
#28844=EDGE_CURVE ( 'NONE', #10173, #1134, #34130, .T. ) ;
#28854=DIRECTION ( 'NONE',  ( 0.000000000000000000, 1.000000000000000000, 0.000000000000000000 ) ) ;
#28857=AXIS2_PLACEMENT_3D ( 'NONE', #20913, #4001, #4179 ) ;
#28866=VERTEX_POINT ( 'NONE', #29330 ) ;
#28867=PLANE ( 'NONE',  #32684 ) ;
#28872=DIRECTION ( 'NONE',  ( 8.498729137172956618E-17, 0.000000000000000000, 1.000000000000000000 ) ) ;
#28874=ORIENTED_EDGE ( 'NONE', *, *, #5373, .T. ) ;
#28876=DIRECTION ( 'NONE',  ( -0.000000000000000000, -1.836970198721029688E-16, 1.000000000000000000 ) ) ;
#28877=PLANE ( 'NONE',  #14133 ) ;
#28883=CARTESIAN_POINT ( 'NONE',  ( -35.00000000000000000, 8.360858262960562115, -23.84547010402785006 ) ) ;
#28886=ORIENTED_EDGE ( 'NONE', *, *, #23478, .F. ) ;
#28894=DIRECTION ( 'NONE',  ( 3.697785493223492838E-32, 1.934419779023891545E-16, -1.000000000000000000 ) ) ;
#28897=ADVANCED_FACE ( 'NONE', ( #4743 ), #31808, .F. ) ;
#28903=CIRCLE ( 'NONE', #12459, 32.54542015209056416 ) ;
#28911=PLANE ( 'NONE',  #23611 ) ;
#28916=AXIS2_PLACEMENT_3D ( 'NONE', #21533, #26689, #2656 ) ;
#28923=LINE ( 'NONE', #11070, #3251 ) ;
#28924=DIRECTION ( 'NONE',  ( -0.000000000000000000, -0.000000000000000000, -1.000000000000000000 ) ) ;
#28933=DIRECTION ( 'NONE',  ( 0.000000000000000000, 1.000000000000000000, 0.000000000000000000 ) ) ;
#28938=EDGE_CURVE ( 'NONE', #28204, #20346, #18148, .T. ) ;
#28939=EDGE_CURVE ( 'NONE', #15487, #29934, #15291, .T. ) ;
#28940=CARTESIAN_POINT ( 'NONE',  ( 0.000000000000000000, 6.992329373473909019E-15, 49.43553178847298568 ) ) ;
#28946=AXIS2_PLACEMENT_3D ( 'NONE', #17875, #20188, #25331 ) ;
#28947=ORIENTED_EDGE ( 'NONE', *, *, #9489, .F. ) ;
#28949=LINE ( 'NONE', #15435, #26448 ) ;
#28960=ADVANCED_FACE ( 'NONE', ( #2434 ), #13317, .F. ) ;
#28964=ORIENTED_EDGE ( 'NONE', *, *, #17905, .F. ) ;
#28968=DIRECTION ( 'NONE',  ( 0.000000000000000000, 1.000000000000000000, 0.000000000000000000 ) ) ;
#28969=CARTESIAN_POINT ( 'NONE',  ( 3.235562306570555532E-30, 1.325223266901699007E-14, -67.50000000000000000 ) ) ;
#28984=FACE_OUTER_BOUND ( 'NONE', #25603, .T. ) ;
#28987=DIRECTION ( 'NONE',  ( -0.000000000000000000, 1.836970198721029934E-16, -1.000000000000000000 ) ) ;
#28991=VERTEX_POINT ( 'NONE', #30856 ) ;
#28993=ORIENTED_EDGE ( 'NONE', *, *, #17549, .T. ) ;
#28996=DIRECTION ( 'NONE',  ( -0.3193015301359796165, 0.9476531711828025673, 0.000000000000000000 ) ) ;
#28998=CARTESIAN_POINT ( 'NONE',  ( -12.25939112814508825, 30.14816249862101927, 68.31122994652405112 ) ) ;
#29000=ORIENTED_EDGE ( 'NONE', *, *, #22135, .F. ) ;
#29009=CARTESIAN_POINT ( 'NONE',  ( 0.000000000000000000, 3.524919873834583163E-15, 68.31122994652405112 ) ) ;
#29018=PLANE ( 'NONE',  #11092 ) ;
#29021=CARTESIAN_POINT ( 'NONE',  ( 0.000000000000000000, 33.69708579775584667, 49.43553178847298568 ) ) ;
#29027=ORIENTED_EDGE ( 'NONE', *, *, #858, .T. ) ;
#29028=VERTEX_POINT ( 'NONE', #22503 ) ;
#29030=EDGE_CURVE ( 'NONE', #5316, #21613, #27173, .T. ) ;
#29036=VERTEX_POINT ( 'NONE', #11837 ) ;
#29039=CARTESIAN_POINT ( 'NONE',  ( 26.97014235612466493, -26.57093094961043889, 68.31122994652405112 ) ) ;
#29040=VERTEX_POINT ( 'NONE', #9136 ) ;
#29055=CARTESIAN_POINT ( 'NONE',  ( 29.83064097883987742, 23.32756518004832813, 68.31122994652405112 ) ) ;
#29060=CARTESIAN_POINT ( 'NONE',  ( -29.68486519896224962, 23.49918569563710946, 68.31122994652405112 ) ) ;
#29062=AXIS2_PLACEMENT_3D ( 'NONE', #28325, #14807, #18014 ) ;
#29064=LINE ( 'NONE', #4324, #1925 ) ;
#29085=DIRECTION ( 'NONE',  ( 1.000000000000000000, 0.000000000000000000, 0.000000000000000000 ) ) ;
#29086=VECTOR ( 'NONE', #27575, 1000.000000000000000 ) ;
#29087=DIRECTION ( 'NONE',  ( 0.7960930657056433102, 0.6051742151937656855, 0.000000000000000000 ) ) ;
#29090=EDGE_CURVE ( 'NONE', #16627, #29871, #28708, .T. ) ;
#29093=DIRECTION ( 'NONE',  ( -0.000000000000000000, 1.836970198721029934E-16, -1.000000000000000000 ) ) ;
#29096=FACE_OUTER_BOUND ( 'NONE', #20212, .T. ) ;
#29097=EDGE_CURVE ( 'NONE', #8552, #17675, #31376, .T. ) ;
#29098=DIRECTION ( 'NONE',  ( 0.3701381553399132329, 0.9289767198167918627, -0.000000000000000000 ) ) ;
#29109=ORIENTED_EDGE ( 'NONE', *, *, #27770, .F. ) ;
#29111=ORIENTED_EDGE ( 'NONE', *, *, #4717, .T. ) ;
#29113=ORIENTED_EDGE ( 'NONE', *, *, #22413, .T. ) ;
#29115=CARTESIAN_POINT ( 'NONE',  ( 0.000000000000000000, 2.281310696040539424E-14, -36.68877005347592757 ) ) ;
#29120=ORIENTED_EDGE ( 'NONE', *, *, #11534, .T. ) ;
#29124=ORIENTED_EDGE ( 'NONE', *, *, #11981, .F. ) ;
#29126=EDGE_LOOP ( 'NONE', ( #18775, #772, #30204, #18087 ) ) ;
#29134=EDGE_CURVE ( 'NONE', #20735, #17606, #25508, .T. ) ;
#29150=ORIENTED_EDGE ( 'NONE', *, *, #19374, .F. ) ;
#29159=LINE ( 'NONE', #26487, #25096 ) ;
#29166=CARTESIAN_POINT ( 'NONE',  ( -9.978866888775733912, -11.61907005722761177, -87.50000000000000000 ) ) ;
#29170=ORIENTED_EDGE ( 'NONE', *, *, #21886, .T. ) ;
#29176=ORIENTED_EDGE ( 'NONE', *, *, #3849, .T. ) ;
#29178=DIRECTION ( 'NONE',  ( -0.000000000000000000, 1.836970198721029934E-16, -1.000000000000000000 ) ) ;
#29179=FACE_OUTER_BOUND ( 'NONE', #1526, .T. ) ;
#29181=EDGE_CURVE ( 'NONE', #13343, #4555, #3960, .T. ) ;
#29184=CARTESIAN_POINT ( 'NONE',  ( 5.021133111224162171, -25.61315202898005694, -87.50000000000000000 ) ) ;
#29185=AXIS2_PLACEMENT_3D ( 'NONE', #33481, #24932, #399 ) ;
#29187=CARTESIAN_POINT ( 'NONE',  ( 22.10765473302597073, -14.55883922869198344, -77.50000000000000000 ) ) ;
#29190=CARTESIAN_POINT ( 'NONE',  ( 5.713835024271039842, 32.03991982186465748, 68.31122994652405112 ) ) ;
#29192=CARTESIAN_POINT ( 'NONE',  ( 10.17231796313411429, 13.56412600238610189, -77.50000000000000000 ) ) ;
#29194=VERTEX_POINT ( 'NONE', #34047 ) ;
#29201=EDGE_LOOP ( 'NONE', ( #23712, #5528, #8884, #18244 ) ) ;
#29203=LINE ( 'NONE', #26701, #18060 ) ;
#29211=DIRECTION ( 'NONE',  ( 1.000000000000000000, 0.000000000000000000, 0.000000000000000000 ) ) ;
#29217=ORIENTED_EDGE ( 'NONE', *, *, #23244, .T. ) ;
#29225=DIRECTION ( 'NONE',  ( 1.000000000000000000, 0.000000000000000000, -0.000000000000000000 ) ) ;
#29227=VECTOR ( 'NONE', #29178, 1000.000000000000000 ) ;
#29230=VERTEX_POINT ( 'NONE', #23539 ) ;
#29231=VERTEX_POINT ( 'NONE', #15371 ) ;
#29237=LINE ( 'NONE', #1485, #26793 ) ;
#29239=CARTESIAN_POINT ( 'NONE',  ( -45.00000000000000000, 42.49491490430484220, -36.69637551990492597 ) ) ;
#29242=VECTOR ( 'NONE', #26153, 1000.000000000000000 ) ;
#29251=ADVANCED_FACE ( 'NONE', ( #31719 ), #7326, .T. ) ;
#29259=ORIENTED_EDGE ( 'NONE', *, *, #31, .F. ) ;
#29262=VECTOR ( 'NONE', #32101, 1000.000000000000000 ) ;
#29263=ORIENTED_EDGE ( 'NONE', *, *, #24735, .F. ) ;
#29269=AXIS2_PLACEMENT_3D ( 'NONE', #28969, #20615, #12273 ) ;
#29272=DIRECTION ( 'NONE',  ( -0.000000000000000000, -0.000000000000000000, -1.000000000000000000 ) ) ;
#29274=VERTEX_POINT ( 'NONE', #12882 ) ;
#29280=CIRCLE ( 'NONE', #13944, 2.033421858999710619 ) ;
#29281=FACE_OUTER_BOUND ( 'NONE', #10189, .T. ) ;
#29288=CARTESIAN_POINT ( 'NONE',  ( 22.10765473302597073, -12.47301499840864025, -77.50000000000000000 ) ) ;
#29289=DIRECTION ( 'NONE',  ( -0.000000000000000000, -1.836970198721029688E-16, 1.000000000000000000 ) ) ;
#29297=CARTESIAN_POINT ( 'NONE',  ( -35.00000000000000000, 16.36947364650383818, 36.69637551990492597 ) ) ;
#29298=VERTEX_POINT ( 'NONE', #7504 ) ;
#29299=EDGE_CURVE ( 'NONE', #11793, #19626, #23882, .T. ) ;
#29301=VECTOR ( 'NONE', #8834, 1000.000000000000114 ) ;
#29305=CIRCLE ( 'NONE', #1455, 32.54542015209055705 ) ;
#29308=PLANE ( 'NONE',  #5751 ) ;
#29314=ORIENTED_EDGE ( 'NONE', *, *, #3412, .F. ) ;
#29327=VECTOR ( 'NONE', #26912, 1000.000000000000000 ) ;
#29328=LINE ( 'NONE', #31977, #33060 ) ;
#29330=CARTESIAN_POINT ( 'NONE',  ( -35.00000000000000000, 8.360858262960560339, 23.84547010402786427 ) ) ;
#29339=CARTESIAN_POINT ( 'NONE',  ( 25.76952721012209224, 19.87802405277948736, 49.43553178847298568 ) ) ;
#29346=ADVANCED_FACE ( 'NONE', ( #32068 ), #26731, .F. ) ;
#29347=EDGE_CURVE ( 'NONE', #5081, #11199, #13224, .T. ) ;
#29367=CARTESIAN_POINT ( 'NONE',  ( -5.021133111224679091, 28.08988295778447508, -67.50000000000000000 ) ) ;
#29368=FACE_OUTER_BOUND ( 'NONE', #20286, .T. ) ;
#29370=VERTEX_POINT ( 'NONE', #10194 ) ;
#29372=DIRECTION ( 'NONE',  ( -0.000000000000000000, -1.836970198721029688E-16, 1.000000000000000000 ) ) ;
#29373=ORIENTED_EDGE ( 'NONE', *, *, #10170, .T. ) ;
#29375=DIRECTION ( 'NONE',  ( 0.000000000000000000, 0.000000000000000000, 1.000000000000000000 ) ) ;
#29383=CARTESIAN_POINT ( 'NONE',  ( 5.021133111224265200, -15.68591377522703390, -87.50000000000000000 ) ) ;
#29389=LINE ( 'NONE', #12677, #5933 ) ;
#29399=CARTESIAN_POINT ( 'NONE',  ( -31.87924797510909869, -6.551177101682124970, 68.31122994652405112 ) ) ;
#29401=ORIENTED_EDGE ( 'NONE', *, *, #21472, .T. ) ;
#29402=VERTEX_POINT ( 'NONE', #24575 ) ;
#29403=DIRECTION ( 'NONE',  ( 0.000000000000000000, 1.836970198721029441E-16, -1.000000000000000000 ) ) ;
#29410=CARTESIAN_POINT ( 'NONE',  ( 23.93847777447631131, 22.04889236939138542, 49.43553178847298568 ) ) ;
#29412=EDGE_CURVE ( 'NONE', #30243, #32960, #24472, .T. ) ;
#29415=CARTESIAN_POINT ( 'NONE',  ( 11.62236370382047745, -30.39942490923500884, 68.31122994652405112 ) ) ;
#29416=EDGE_LOOP ( 'NONE', ( #7408, #17557, #11745, #34529 ) ) ;
#29423=FACE_OUTER_BOUND ( 'NONE', #33005, .T. ) ;
#29424=DIRECTION ( 'NONE',  ( 0.000000000000000000, 0.000000000000000000, -1.000000000000000000 ) ) ;
#29430=VERTEX_POINT ( 'NONE', #24763 ) ;
#29435=ORIENTED_EDGE ( 'NONE', *, *, #3654, .T. ) ;
#29438=ORIENTED_EDGE ( 'NONE', *, *, #522, .F. ) ;
#29439=AXIS2_PLACEMENT_3D ( 'NONE', #34941, #23723, #10557 ) ;
#29443=FACE_BOUND ( 'NONE', #17280, .T. ) ;
#29449=EDGE_CURVE ( 'NONE', #29973, #2835, #29941, .T. ) ;
#29450=ADVANCED_FACE ( 'NONE', ( #21927 ), #19273, .F. ) ;
#29456=CARTESIAN_POINT ( 'NONE',  ( -32.71222340678873053, 19.07754906224035807, -36.68877005347593467 ) ) ;
#29461=LINE ( 'NONE', #23592, #8810 ) ;
#29462=AXIS2_PLACEMENT_3D ( 'NONE', #34214, #20696, #18743 ) ;
#29469=PLANE ( 'NONE',  #1308 ) ;
#29471=VECTOR ( 'NONE', #15488, 1000.000000000000000 ) ;
#29476=DIRECTION ( 'NONE',  ( 0.000000000000000000, 0.000000000000000000, 1.000000000000000000 ) ) ;
#29477=LINE ( 'NONE', #16313, #26757 ) ;
#29482=ORIENTED_EDGE ( 'NONE', *, *, #9151, .F. ) ;
#29486=EDGE_CURVE ( 'NONE', #20346, #11447, #25289, .T. ) ;
#29496=DIRECTION ( 'NONE',  ( -0.000000000000000000, -1.836970198721029688E-16, 1.000000000000000000 ) ) ;
#29504=CARTESIAN_POINT ( 'NONE',  ( -45.42888529050880209, 14.20380584968301640, 33.22126893951599413 ) ) ;
#29508=LINE ( 'NONE', #13318, #7189 ) ;
#29509=CARTESIAN_POINT ( 'NONE',  ( -36.80830595996284416, 8.862931941313791029, -36.68877005347593467 ) ) ;
#29516=VECTOR ( 'NONE', #28830, 1000.000000000000000 ) ;
#29519=CARTESIAN_POINT ( 'NONE',  ( -30.91434716440808117, 10.17386417614055638, -36.68877005347593467 ) ) ;
#29523=DIRECTION ( 'NONE',  ( -0.1617819965527647619, -0.9868265225415261410, -1.812770913216290044E-16 ) ) ;
#29529=PLANE ( 'NONE',  #12733 ) ;
#29538=ADVANCED_FACE ( 'NONE', ( #20485 ), #3920, .F. ) ;
#29540=EDGE_CURVE ( 'NONE', #10055, #18879, #30992, .T. ) ;
#29544=ORIENTED_EDGE ( 'NONE', *, *, #24168, .T. ) ;
#29548=EDGE_LOOP ( 'NONE', ( #59, #23722, #1998, #12871 ) ) ;
#29549=DIRECTION ( 'NONE',  ( 1.000000000000000000, 0.000000000000000000, -0.000000000000000000 ) ) ;
#29551=ORIENTED_EDGE ( 'NONE', *, *, #24735, .T. ) ;
#29558=EDGE_CURVE ( 'NONE', #27628, #28173, #1775, .T. ) ;
#29566=ADVANCED_FACE ( 'NONE', ( #12138 ), #34178, .T. ) ;
#29567=DIRECTION ( 'NONE',  ( 0.000000000000000000, 1.000000000000000000, 0.000000000000000000 ) ) ;
#29573=LINE ( 'NONE', #29399, #34111 ) ;
#29576=DIRECTION ( 'NONE',  ( 0.000000000000000000, 0.000000000000000000, 1.000000000000000000 ) ) ;
#29578=CARTESIAN_POINT ( 'NONE',  ( 0.000000000000000000, 33.69708579775584667, -36.68877005347592757 ) ) ;
#29579=VERTEX_POINT ( 'NONE', #4269 ) ;
#29586=DIRECTION ( 'NONE',  ( -0.000000000000000000, 1.836970198721029934E-16, -1.000000000000000000 ) ) ;
#29597=CARTESIAN_POINT ( 'NONE',  ( 32.05156013847309993, -20.15193397489277771, 49.43553178847298568 ) ) ;
#29598=CARTESIAN_POINT ( 'NONE',  ( -35.00000000000000000, 16.36473396058513075, -36.68877005347592757 ) ) ;
#29604=EDGE_CURVE ( 'NONE', #6574, #17675, #25819, .T. ) ;
#29605=EDGE_CURVE ( 'NONE', #13484, #2324, #23164, .T. ) ;
#29613=PLANE ( 'NONE',  #24104 ) ;
#29615=VERTEX_POINT ( 'NONE', #19966 ) ;
#29622=ORIENTED_EDGE ( 'NONE', *, *, #5118, .T. ) ;
#29624=DIRECTION ( 'NONE',  ( -0.000000000000000000, 1.836970198721029934E-16, -1.000000000000000000 ) ) ;
#29630=EDGE_LOOP ( 'NONE', ( #15264, #12032 ) ) ;
#29631=AXIS2_PLACEMENT_3D ( 'NONE', #34072, #10534, #24031 ) ;
#29637=FACE_OUTER_BOUND ( 'NONE', #8208, .T. ) ;
#29639=DIRECTION ( 'NONE',  ( -0.000000000000000000, 1.836970198721029934E-16, -1.000000000000000000 ) ) ;
#29642=CARTESIAN_POINT ( 'NONE',  ( 0.000000000000000000, 2.281310696040539424E-14, -36.68877005347594178 ) ) ;
#29643=AXIS2_PLACEMENT_3D ( 'NONE', #22679, #11830, #30504 ) ;
#29654=VECTOR ( 'NONE', #327, 1000.000000000000000 ) ;
#29659=ORIENTED_EDGE ( 'NONE', *, *, #32145, .T. ) ;
#29660=CIRCLE ( 'NONE', #33083, 32.54542015209057126 ) ;
#29664=FACE_OUTER_BOUND ( 'NONE', #14237, .T. ) ;
#29666=ORIENTED_EDGE ( 'NONE', *, *, #27232, .F. ) ;
#29673=DIRECTION ( 'NONE',  ( -0.02866416272524431944, -0.5286793732840951998, 0.8483374835754913246 ) ) ;
#29679=VECTOR ( 'NONE', #27588, 1000.000000000000000 ) ;
#29682=VECTOR ( 'NONE', #15779, 1000.000000000000114 ) ;
#29683=VECTOR ( 'NONE', #8284, 1000.000000000000227 ) ;
#29685=ORIENTED_EDGE ( 'NONE', *, *, #26740, .T. ) ;
#29695=VERTEX_POINT ( 'NONE', #15689 ) ;
#29700=DIRECTION ( 'NONE',  ( 0.000000000000000000, -1.000000000000000000, -1.836970198721029934E-16 ) ) ;
#29713=DIRECTION ( 'NONE',  ( -0.2675283385292215321, -0.9635499925192227977, -0.000000000000000000 ) ) ;
#29715=EDGE_LOOP ( 'NONE', ( #31654, #33593, #26578, #9969, #19580, #13737, #4925, #7490, #21521, #13865 ) ) ;
#29717=ORIENTED_EDGE ( 'NONE', *, *, #21132, .T. ) ;
#29719=CARTESIAN_POINT ( 'NONE',  ( 32.81769769215652133, 18.87860345536237006, 68.31122994652405112 ) ) ;
#29720=VERTEX_POINT ( 'NONE', #32211 ) ;
#29724=ORIENTED_EDGE ( 'NONE', *, *, #14068, .F. ) ;
#29732=AXIS2_PLACEMENT_3D ( 'NONE', #3549, #8371, #16934 ) ;
#29742=ORIENTED_EDGE ( 'NONE', *, *, #20389, .F. ) ;
#29743=ORIENTED_EDGE ( 'NONE', *, *, #18799, .T. ) ;
#29752=CARTESIAN_POINT ( 'NONE',  ( -49.20661276131353645, 21.27332514515927286, 0.4570320086110524205 ) ) ;
#29755=ORIENTED_EDGE ( 'NONE', *, *, #28014, .F. ) ;
#29757=DIRECTION ( 'NONE',  ( -1.000000000000000000, 6.792721752314501023E-48, -3.697785493223492838E-32 ) ) ;
#29769=LINE ( 'NONE', #409, #31037 ) ;
#29781=EDGE_CURVE ( 'NONE', #3900, #10873, #20833, .T. ) ;
#29782=AXIS2_PLACEMENT_3D ( 'NONE', #5467, #34866, #10476 ) ;
#29787=CARTESIAN_POINT ( 'NONE',  ( 23.31255882915078814, -22.70966696615089830, 68.31122994652405112 ) ) ;
#29795=ORIENTED_EDGE ( 'NONE', *, *, #27108, .T. ) ;
#29802=CARTESIAN_POINT ( 'NONE',  ( 22.89764159710613001, 8.346743312457581609, -87.50000000000000000 ) ) ;
#29803=VERTEX_POINT ( 'NONE', #7997 ) ;
#29805=EDGE_CURVE ( 'NONE', #28395, #17606, #1961, .T. ) ;
#29806=CARTESIAN_POINT ( 'NONE',  ( -23.48826533576967179, -5.175545323022858746, -16.02576232019386993 ) ) ;
#29807=VECTOR ( 'NONE', #18928, 999.9999999999998863 ) ;
#29808=DIRECTION ( 'NONE',  ( 0.000000000000000000, 1.000000000000000000, 0.000000000000000000 ) ) ;
#29813=LINE ( 'NONE', #18965, #18894 ) ;
#29816=VERTEX_POINT ( 'NONE', #29719 ) ;
#29818=ORIENTED_EDGE ( 'NONE', *, *, #21690, .T. ) ;
#29825=EDGE_CURVE ( 'NONE', #13030, #2206, #16035, .T. ) ;
#29828=AXIS2_PLACEMENT_3D ( 'NONE', #33792, #20274, #23968 ) ;
#29829=ORIENTED_EDGE ( 'NONE', *, *, #10528, .T. ) ;
#29834=DIRECTION ( 'NONE',  ( -0.000000000000000000, 1.836970198721029934E-16, -1.000000000000000000 ) ) ;
#29841=LINE ( 'NONE', #13644, #13116 ) ;
#29843=ORIENTED_EDGE ( 'NONE', *, *, #18852, .F. ) ;
#29845=CARTESIAN_POINT ( 'NONE',  ( 18.63894936814906345, 26.67946662374789213, 68.31122994652405112 ) ) ;
#29847=FACE_OUTER_BOUND ( 'NONE', #32531, .T. ) ;
#29849=EDGE_CURVE ( 'NONE', #11336, #26209, #13152, .T. ) ;
#29855=DIRECTION ( 'NONE',  ( 0.000000000000000000, 1.836970198721029441E-16, -1.000000000000000000 ) ) ;
#29858=VECTOR ( 'NONE', #5618, 1000.000000000000000 ) ;
#29863=ORIENTED_EDGE ( 'NONE', *, *, #33727, .F. ) ;
#29864=VECTOR ( 'NONE', #26102, 1000.000000000000000 ) ;
#29867=VERTEX_POINT ( 'NONE', #19758 ) ;
#29871=VERTEX_POINT ( 'NONE', #11030 ) ;
#29877=ORIENTED_EDGE ( 'NONE', *, *, #29805, .T. ) ;
#29889=CARTESIAN_POINT ( 'NONE',  ( 1.991296462759135633, -32.48444414290481319, 49.43553178847298568 ) ) ;
#29891=ADVANCED_FACE ( 'NONE', ( #25063 ), #5843, .T. ) ;
#29892=DIRECTION ( 'NONE',  ( 1.000000000000000000, 0.000000000000000000, -0.000000000000000000 ) ) ;
#29894=VECTOR ( 'NONE', #34972, 1000.000000000000114 ) ;
#29900=EDGE_LOOP ( 'NONE', ( #28726, #14240, #4265, #27556 ) ) ;
#29905=VECTOR ( 'NONE', #3432, 1000.000000000000227 ) ;
#29909=VECTOR ( 'NONE', #27264, 1000.000000000000000 ) ;
#29934=VERTEX_POINT ( 'NONE', #17091 ) ;
#29935=ORIENTED_EDGE ( 'NONE', *, *, #11395, .T. ) ;
#29940=CARTESIAN_POINT ( 'NONE',  ( 9.630725478591894984, 36.62364762272929397, 68.31122994652405112 ) ) ;
#29941=LINE ( 'NONE', #2867, #12017 ) ;
#29962=ORIENTED_EDGE ( 'NONE', *, *, #4112, .T. ) ;
#29963=CARTESIAN_POINT ( 'NONE',  ( 0.000000000000000000, 3.214697847761802057E-14, -87.50000000000000000 ) ) ;
#29964=ORIENTED_EDGE ( 'NONE', *, *, #24646, .T. ) ;
#29973=VERTEX_POINT ( 'NONE', #21707 ) ;
#29974=DIRECTION ( 'NONE',  ( 1.000000000000000000, 0.000000000000000000, 0.000000000000000000 ) ) ;
#29976=EDGE_CURVE ( 'NONE', #16944, #20519, #14242, .T. ) ;
#29979=LINE ( 'NONE', #77, #34725 ) ;
#29981=AXIS2_PLACEMENT_3D ( 'NONE', #19183, #10635, #13132 ) ;
#29982=DIRECTION ( 'NONE',  ( 0.000000000000000000, -1.000000000000000000, 0.000000000000000000 ) ) ;
#29986=ORIENTED_EDGE ( 'NONE', *, *, #9076, .T. ) ;
#29987=LINE ( 'NONE', #30333, #1445 ) ;
#29989=DIRECTION ( 'NONE',  ( -1.000000000000000000, -0.000000000000000000, -0.000000000000000000 ) ) ;
#29994=ORIENTED_EDGE ( 'NONE', *, *, #5718, .T. ) ;
#30001=ORIENTED_EDGE ( 'NONE', *, *, #5368, .F. ) ;
#30002=CARTESIAN_POINT ( 'NONE',  ( 0.000000000000000000, -33.69708579775584667, -49.43553178847298568 ) ) ;
#30008=DIRECTION ( 'NONE',  ( 0.000000000000000000, 1.836970198721029688E-16, -1.000000000000000000 ) ) ;
#30009=DIRECTION ( 'NONE',  ( 1.000000000000000000, 0.000000000000000000, -0.000000000000000000 ) ) ;
#30010=ORIENTED_EDGE ( 'NONE', *, *, #12806, .F. ) ;
#30011=ORIENTED_EDGE ( 'NONE', *, *, #9720, .F. ) ;
#30016=CARTESIAN_POINT ( 'NONE',  ( 3.235562306570555532E-30, 1.325223266901699007E-14, -67.50000000000000000 ) ) ;
#30018=ORIENTED_EDGE ( 'NONE', *, *, #28938, .T. ) ;
#30019=LINE ( 'NONE', #7767, #31571 ) ;
#30021=DIRECTION ( 'NONE',  ( 0.9289767198167909745, -0.3701381553399156199, 0.000000000000000000 ) ) ;
#30024=DIRECTION ( 'NONE',  ( 0.000000000000000000, 1.836970198721029441E-16, -1.000000000000000000 ) ) ;
#30025=EDGE_CURVE ( 'NONE', #5728, #11221, #33614, .T. ) ;
#30027=CARTESIAN_POINT ( 'NONE',  ( 5.713835024271038954, 32.03991982186465748, 49.43553178847298568 ) ) ;
#30028=DIRECTION ( 'NONE',  ( 1.000000000000000000, 0.000000000000000000, 0.000000000000000000 ) ) ;
#30029=CIRCLE ( 'NONE', #7782, 32.54542015209057126 ) ;
#30035=CARTESIAN_POINT ( 'NONE',  ( 0.000000000000000000, -33.69708579775584667, 49.43553178847298568 ) ) ;
#30039=FACE_OUTER_BOUND ( 'NONE', #5251, .T. ) ;
#30041=VECTOR ( 'NONE', #11244, 1000.000000000000114 ) ;
#30071=ORIENTED_EDGE ( 'NONE', *, *, #34271, .T. ) ;
#30084=DIRECTION ( 'NONE',  ( 1.000000000000000000, 0.000000000000000000, -0.000000000000000000 ) ) ;
#30087=DIRECTION ( 'NONE',  ( 0.000000000000000000, 1.836970198721029934E-16, -1.000000000000000000 ) ) ;
#30088=CARTESIAN_POINT ( 'NONE',  ( 0.000000000000000000, 3.524919873834583163E-15, 68.31122994652405112 ) ) ;
#30100=DIRECTION ( 'NONE',  ( 0.000000000000000000, 1.836970198721029441E-16, -1.000000000000000000 ) ) ;
#30106=DIRECTION ( 'NONE',  ( 0.000000000000000000, 1.000000000000000000, 0.000000000000000000 ) ) ;
#30107=CARTESIAN_POINT ( 'NONE',  ( 5.021133111224473033, 8.235406450278427215, -67.50000000000000000 ) ) ;
#30119=PLANE ( 'NONE',  #31527 ) ;
#30120=DIRECTION ( 'NONE',  ( 0.5611870653623822758, 0.8276889981568905652, -0.000000000000000000 ) ) ;
#30126=EDGE_CURVE ( 'NONE', #18315, #8996, #34673, .T. ) ;
#30129=VERTEX_POINT ( 'NONE', #21499 ) ;
#30131=ORIENTED_EDGE ( 'NONE', *, *, #32251, .F. ) ;
#30136=DIRECTION ( 'NONE',  ( 0.000000000000000000, 1.836970198721029441E-16, -1.000000000000000000 ) ) ;
#30140=ORIENTED_EDGE ( 'NONE', *, *, #6200, .F. ) ;
#30145=LINE ( 'NONE', #5407, #5156 ) ;
#30152=CARTESIAN_POINT ( 'NONE',  ( -15.64512930492132448, -28.53829535743847856, 68.31122994652405112 ) ) ;
#30161=CARTESIAN_POINT ( 'NONE',  ( 14.70109753509668948, 34.88954974633765005, 68.31122994652405112 ) ) ;
#30168=ADVANCED_FACE ( 'NONE', ( #24152 ), #13142, .T. ) ;
#30175=CARTESIAN_POINT ( 'NONE',  ( 5.021133111224265200, -15.68591377522703745, -67.50000000000000000 ) ) ;
#30179=CARTESIAN_POINT ( 'NONE',  ( -20.02113311122488781, 8.235406450278427215, -67.50000000000000000 ) ) ;
#30182=DIRECTION ( 'NONE',  ( 1.000000000000000000, 0.000000000000000000, 0.000000000000000000 ) ) ;
#30185=ORIENTED_EDGE ( 'NONE', *, *, #34922, .T. ) ;
#30187=CIRCLE ( 'NONE', #3479, 32.54542015209056416 ) ;
#30191=FACE_OUTER_BOUND ( 'NONE', #32298, .T. ) ;
#30193=CARTESIAN_POINT ( 'NONE',  ( -25.07182831876307105, -28.36910952062234870, 68.31122994652405112 ) ) ;
#30196=ORIENTED_EDGE ( 'NONE', *, *, #13033, .F. ) ;
#30203=DIRECTION ( 'NONE',  ( -0.05413890858541543089, -0.9985334138511240409, 0.000000000000000000 ) ) ;
#30204=ORIENTED_EDGE ( 'NONE', *, *, #19340, .F. ) ;
#30213=AXIS2_PLACEMENT_3D ( 'NONE', #30478, #25474, #33488 ) ;
#30216=EDGE_CURVE ( 'NONE', #12565, #10302, #21834, .T. ) ;
#30222=CARTESIAN_POINT ( 'NONE',  ( -37.12776225901827587, -7.411627343331148587, 17.41927665145494686 ) ) ;
#30227=EDGE_LOOP ( 'NONE', ( #30277, #34861, #7380, #5141 ) ) ;
#30229=EDGE_CURVE ( 'NONE', #30758, #10803, #5279, .T. ) ;
#30233=VECTOR ( 'NONE', #2102, 1000.000000000000114 ) ;
#30235=ORIENTED_EDGE ( 'NONE', *, *, #25004, .F. ) ;
#30237=VECTOR ( 'NONE', #5767, 1000.000000000000000 ) ;
#30238=ORIENTED_EDGE ( 'NONE', *, *, #18264, .T. ) ;
#30243=VERTEX_POINT ( 'NONE', #16169 ) ;
#30250=CARTESIAN_POINT ( 'NONE',  ( -45.00000000000000000, -4.831299144296466785, 15.81122994652406355 ) ) ;
#30254=CARTESIAN_POINT ( 'NONE',  ( 3.235562306570555532E-30, 14.09580098603202458, -67.50000000000000000 ) ) ;
#30262=CYLINDRICAL_SURFACE ( 'NONE', #6321, 2.036051781435508801 ) ;
#30268=LINE ( 'NONE', #5867, #19341 ) ;
#30270=ORIENTED_EDGE ( 'NONE', *, *, #6204, .F. ) ;
#30271=CARTESIAN_POINT ( 'NONE',  ( 10.17231796313407344, -5.651112684911596240, -87.50000000000000000 ) ) ;
#30277=ORIENTED_EDGE ( 'NONE', *, *, #11587, .T. ) ;
#30278=CARTESIAN_POINT ( 'NONE',  ( -15.64512930492131382, -28.53829535743846435, 68.31122994652405112 ) ) ;
#30279=LINE ( 'NONE', #29940, #31782 ) ;
#30281=PLANE ( 'NONE',  #26921 ) ;
#30291=ORIENTED_EDGE ( 'NONE', *, *, #21122, .T. ) ;
#30294=CYLINDRICAL_SURFACE ( 'NONE', #10423, 2.033421858999710619 ) ;
#30298=ORIENTED_EDGE ( 'NONE', *, *, #20040, .T. ) ;
#30300=CARTESIAN_POINT ( 'NONE',  ( 0.000000000000000000, 6.992329373473909019E-15, 49.43553178847298568 ) ) ;
#30309=ORIENTED_EDGE ( 'NONE', *, *, #9565, .T. ) ;
#30310=VERTEX_POINT ( 'NONE', #2619 ) ;
#30311=ADVANCED_FACE ( 'NONE', ( #11349 ), #19537, .F. ) ;
#30312=CARTESIAN_POINT ( 'NONE',  ( 22.89764159710613001, 4.274639749586562232, -87.50000000000000000 ) ) ;
#30314=ORIENTED_EDGE ( 'NONE', *, *, #19989, .T. ) ;
#30323=DIRECTION ( 'NONE',  ( -0.1617819965527614312, 0.9868265225415265851, 0.000000000000000000 ) ) ;
#30325=ORIENTED_EDGE ( 'NONE', *, *, #23258, .T. ) ;
#30333=CARTESIAN_POINT ( 'NONE',  ( 11.62236370382047745, -30.39942490923498752, -36.68877005347593467 ) ) ;
#30334=LINE ( 'NONE', #13795, #14939 ) ;
#30344=ORIENTED_EDGE ( 'NONE', *, *, #6070, .T. ) ;
#30345=LINE ( 'NONE', #8461, #10935 ) ;
#30348=ORIENTED_EDGE ( 'NONE', *, *, #28013, .T. ) ;
#30360=AXIS2_PLACEMENT_3D ( 'NONE', #26355, #25830, #1973 ) ;
#30362=DIRECTION ( 'NONE',  ( 0.9052067871510963704, 0.3606673485459945261, -0.2247659586956879396 ) ) ;
#30365=AXIS2_PLACEMENT_3D ( 'NONE', #6827, #3455, #34066 ) ;
#30368=CARTESIAN_POINT ( 'NONE',  ( 0.000000000000000000, 3.524919873834583163E-15, 68.31122994652405112 ) ) ;
#30372=DIRECTION ( 'NONE',  ( -0.000000000000000000, -1.836970198721029688E-16, 1.000000000000000000 ) ) ;
#30376=CARTESIAN_POINT ( 'NONE',  ( -20.82057426567703473, -31.63141042832694083, 68.31122994652405112 ) ) ;
#30377=CARTESIAN_POINT ( 'NONE',  ( 4.815661544189686616, -32.18716788982706589, 68.31122994652405112 ) ) ;
#30383=ORIENTED_EDGE ( 'NONE', *, *, #10617, .F. ) ;
#30391=EDGE_CURVE ( 'NONE', #17657, #23884, #33932, .T. ) ;
#30395=ORIENTED_EDGE ( 'NONE', *, *, #5280, .T. ) ;
#30398=DIRECTION ( 'NONE',  ( 0.000000000000000000, 1.000000000000000000, 0.000000000000000000 ) ) ;
#30404=DIRECTION ( 'NONE',  ( 1.000000000000000000, 0.000000000000000000, -0.000000000000000000 ) ) ;
#30406=AXIS2_PLACEMENT_3D ( 'NONE', #6760, #25981, #14631 ) ;
#30407=PLANE ( 'NONE',  #20169 ) ;
#30413=VECTOR ( 'NONE', #18310, 1000.000000000000000 ) ;
#30414=CARTESIAN_POINT ( 'NONE',  ( 2.567399184519788768, -37.78162119159486565, 68.31122994652405112 ) ) ;
#30416=PLANE ( 'NONE',  #25863 ) ;
#30417=VECTOR ( 'NONE', #33406, 1000.000000000000000 ) ;
#30422=ORIENTED_EDGE ( 'NONE', *, *, #12367, .T. ) ;
#30425=EDGE_CURVE ( 'NONE', #19968, #13940, #6156, .T. ) ;
#30427=EDGE_LOOP ( 'NONE', ( #22592, #21406, #32056, #12212 ) ) ;
#30428=EDGE_LOOP ( 'NONE', ( #29401, #17681, #25429, #24696 ) ) ;
#30430=EDGE_CURVE ( 'NONE', #11323, #29274, #15076, .T. ) ;
#30438=AXIS2_PLACEMENT_3D ( 'NONE', #19349, #14368, #8649 ) ;
#30441=CARTESIAN_POINT ( 'NONE',  ( -5.491809612354312975, 32.07872192057775607, -36.68877005347593467 ) ) ;
#30450=ORIENTED_EDGE ( 'NONE', *, *, #5438, .F. ) ;
#30456=VERTEX_POINT ( 'NONE', #30564 ) ;
#30460=AXIS2_PLACEMENT_3D ( 'NONE', #10228, #13607, #8081 ) ;
#30464=ORIENTED_EDGE ( 'NONE', *, *, #8484, .F. ) ;
#30465=DIRECTION ( 'NONE',  ( 0.1617819965527614312, -0.9868265225415265851, 0.000000000000000000 ) ) ;
#30478=CARTESIAN_POINT ( 'NONE',  ( 0.000000000000000000, 3.524919873834583163E-15, 68.31122994652405112 ) ) ;
#30480=CARTESIAN_POINT ( 'NONE',  ( -20.02113311122509032, -15.68591377522703390, -87.50000000000000000 ) ) ;
#30491=VECTOR ( 'NONE', #14378, 1000.000000000000000 ) ;
#30496=FACE_OUTER_BOUND ( 'NONE', #4876, .T. ) ;
#30504=DIRECTION ( 'NONE',  ( 0.9985334138511239299, -0.05413890858541763051, 0.000000000000000000 ) ) ;
#30509=CARTESIAN_POINT ( 'NONE',  ( 0.000000000000000000, 10.87635688602997597, 87.50000000000000000 ) ) ;
#30510=VECTOR ( 'NONE', #8927, 1000.000000000000000 ) ;
#30518=SHAPE_REPRESENTATION ( 'motor', ( #28566 ), #18940 ) ;
#30520=DIRECTION ( 'NONE',  ( -0.000000000000000000, -0.000000000000000000, 1.000000000000000000 ) ) ;
#30521=PLANE ( 'NONE',  #28568 ) ;
#30537=ADVANCED_FACE ( 'NONE', ( #9892 ), #10243, .T. ) ;
#30543=VERTEX_POINT ( 'NONE', #7736 ) ;
#30544=ORIENTED_EDGE ( 'NONE', *, *, #24749, .T. ) ;
#30545=DIRECTION ( 'NONE',  ( -1.000000000000000000, -0.000000000000000000, -0.000000000000000000 ) ) ;
#30549=DIRECTION ( 'NONE',  ( -0.000000000000000000, -0.000000000000000000, -1.000000000000000000 ) ) ;
#30564=CARTESIAN_POINT ( 'NONE',  ( -18.38714294329533416, -33.09555747561019245, -36.68877005347593467 ) ) ;
#30568=CIRCLE ( 'NONE', #3843, 2.033421858999711507 ) ;
#30569=LINE ( 'NONE', #8495, #7561 ) ;
#30577=EDGE_CURVE ( 'NONE', #3029, #18315, #7555, .T. ) ;
#30583=EDGE_CURVE ( 'NONE', #6917, #12135, #4654, .T. ) ;
#30586=CIRCLE ( 'NONE', #34543, 2.033421858999711951 ) ;
#30587=CIRCLE ( 'NONE', #13513, 32.54542015209055705 ) ;
#30590=ORIENTED_EDGE ( 'NONE', *, *, #6534, .T. ) ;
#30596=AXIS2_PLACEMENT_3D ( 'NONE', #26729, #24402, #2342 ) ;
#30612=PLANE ( 'NONE',  #24631 ) ;
#30613=DIRECTION ( 'NONE',  ( -6.189473249308364160E-17, 0.000000000000000000, 1.000000000000000000 ) ) ;
#30625=ORIENTED_EDGE ( 'NONE', *, *, #30391, .F. ) ;
#30630=EDGE_CURVE ( 'NONE', #29298, #24529, #29813, .T. ) ;
#30639=DIRECTION ( 'NONE',  ( -0.000000000000000000, 0.8486862100397269959, 0.5288966977476833309 ) ) ;
#30640=ORIENTED_EDGE ( 'NONE', *, *, #565, .T. ) ;
#30642=CARTESIAN_POINT ( 'NONE',  ( -37.12776225901827587, -7.411627343331159246, -15.81122994652406355 ) ) ;
#30643=DIRECTION ( 'NONE',  ( 0.9985334138511240409, -0.05413890858541543089, -9.945156166269024927E-18 ) ) ;
#30648=AXIS2_PLACEMENT_3D ( 'NONE', #26301, #28798, #1741 ) ;
#30649=CARTESIAN_POINT ( 'NONE',  ( -32.54223829851967764, 0.4550817492056254410, -15.81122994652406355 ) ) ;
#30657=CARTESIAN_POINT ( 'NONE',  ( 60.00000000000000000, -33.69708579775584667, 49.43553178847298568 ) ) ;
#30666=ORIENTED_EDGE ( 'NONE', *, *, #10922, .F. ) ;
#30677=CARTESIAN_POINT ( 'NONE',  ( -37.85301660235036536, 0.7430237821112573027, 68.31122994652405112 ) ) ;
#30680=ORIENTED_EDGE ( 'NONE', *, *, #9237, .T. ) ;
#30695=LINE ( 'NONE', #34058, #9851 ) ;
#30696=VECTOR ( 'NONE', #12191, 1000.000000000000114 ) ;
#30697=EDGE_CURVE ( 'NONE', #750, #14972, #24625, .T. ) ;
#30700=EDGE_CURVE ( 'NONE', #28220, #14210, #30334, .T. ) ;
#30702=ORIENTED_EDGE ( 'NONE', *, *, #20074, .F. ) ;
#30704=CARTESIAN_POINT ( 'NONE',  ( -20.02113311122509032, -11.61907005722761177, -87.50000000000000000 ) ) ;
#30709=DIRECTION ( 'NONE',  ( -1.000000000000000000, 0.000000000000000000, 0.000000000000000000 ) ) ;
#30712=VERTEX_POINT ( 'NONE', #16477 ) ;
#30720=CARTESIAN_POINT ( 'NONE',  ( 1.991296462759137853, -32.48444414290483451, 68.31122994652405112 ) ) ;
#30722=VERTEX_POINT ( 'NONE', #30152 ) ;
#30725=DIRECTION ( 'NONE',  ( -1.000000000000000000, 6.792721752314501023E-48, -3.697785493223492838E-32 ) ) ;
#30736=ADVANCED_FACE ( 'NONE', ( #790 ), #17014, .F. ) ;
#30743=ORIENTED_EDGE ( 'NONE', *, *, #7938, .T. ) ;
#30745=DIRECTION ( 'NONE',  ( -0.3193015301359797276, 0.9476531711828024562, -0.000000000000000000 ) ) ;
#30748=AXIS2_PLACEMENT_3D ( 'NONE', #26908, #27086, #21044 ) ;
#30751=CARTESIAN_POINT ( 'NONE',  ( -29.72561944762171393, -13.25111019240557475, -36.68877005347593467 ) ) ;
#30752=ORIENTED_EDGE ( 'NONE', *, *, #3088, .F. ) ;
#30758=VERTEX_POINT ( 'NONE', #11479 ) ;
#30759=ORIENTED_EDGE ( 'NONE', *, *, #30697, .T. ) ;
#30778=VECTOR ( 'NONE', #12315, 1000.000000000000000 ) ;
#30786=CARTESIAN_POINT ( 'NONE',  ( -9.410814080250917257, 36.67205378194066867, -36.68877005347593467 ) ) ;
#30791=ORIENTED_EDGE ( 'NONE', *, *, #1926, .F. ) ;
#30797=ORIENTED_EDGE ( 'NONE', *, *, #29449, .T. ) ;
#30798=AXIS2_PLACEMENT_3D ( 'NONE', #32880, #142, #27366 ) ;
#30800=VECTOR ( 'NONE', #14379, 1000.000000000000000 ) ;
#30805=VECTOR ( 'NONE', #7416, 1000.000000000000227 ) ;
#30807=CARTESIAN_POINT ( 'NONE',  ( 0.000000000000000000, 3.524919873834583163E-15, 68.31122994652405112 ) ) ;
#30813=LINE ( 'NONE', #31168, #31618 ) ;
#30826=DIRECTION ( 'NONE',  ( -0.9289767198167914186, 0.3701381553399144542, 0.000000000000000000 ) ) ;
#30830=EDGE_CURVE ( 'NONE', #28173, #10186, #31048, .T. ) ;
#30840=EDGE_LOOP ( 'NONE', ( #27593, #29964, #7567, #13395, #9312, #17345 ) ) ;
#30847=DIRECTION ( 'NONE',  ( 0.4198891015602640997, 0.9075754196709572286, 0.000000000000000000 ) ) ;
#30848=VECTOR ( 'NONE', #22423, 1000.000000000000000 ) ;
#30851=EDGE_LOOP ( 'NONE', ( #16724, #27285, #29109, #23527 ) ) ;
#30856=CARTESIAN_POINT ( 'NONE',  ( 0.000000000000000000, -32.54542015209057126, 76.74945698428001606 ) ) ;
#30858=ORIENTED_EDGE ( 'NONE', *, *, #20017, .T. ) ;
#30861=ORIENTED_EDGE ( 'NONE', *, *, #30932, .F. ) ;
#30863=DIRECTION ( 'NONE',  ( 0.000000000000000000, 1.836970198721029441E-16, -1.000000000000000000 ) ) ;
#30864=DIRECTION ( 'NONE',  ( 0.8276889981568904542, 0.5611870653623824978, -0.000000000000000000 ) ) ;
#30867=PLANE ( 'NONE',  #5960 ) ;
#30877=ORIENTED_EDGE ( 'NONE', *, *, #12870, .F. ) ;
#30878=VECTOR ( 'NONE', #14660, 1000.000000000000114 ) ;
#30880=CARTESIAN_POINT ( 'NONE',  ( -45.00000000000000000, 3.353962854566122864, -15.81122994652406355 ) ) ;
#30883=EDGE_CURVE ( 'NONE', #28025, #30456, #11662, .T. ) ;
#30884=EDGE_LOOP ( 'NONE', ( #1994, #19759, #12888, #14630 ) ) ;
#30887=ORIENTED_EDGE ( 'NONE', *, *, #18175, .T. ) ;
#30889=ADVANCED_FACE ( 'NONE', ( #6645 ), #30521, .T. ) ;
#30890=FACE_OUTER_BOUND ( 'NONE', #29416, .T. ) ;
#30907=VECTOR ( 'NONE', #28298, 1000.000000000000000 ) ;
#30913=EDGE_CURVE ( 'NONE', #9416, #32148, #15872, .T. ) ;
#30921=DIRECTION ( 'NONE',  ( 0.9635499925192230197, -0.2675283385292204774, -0.000000000000000000 ) ) ;
#30924=VERTEX_POINT ( 'NONE', #12365 ) ;
#30932=EDGE_CURVE ( 'NONE', #33546, #12281, #31953, .T. ) ;
#30947=DIRECTION ( 'NONE',  ( -0.6051742151937650194, 0.7960930657056437543, 0.000000000000000000 ) ) ;
#30950=EDGE_CURVE ( 'NONE', #11706, #24474, #10329, .T. ) ;
#30958=VECTOR ( 'NONE', #11046, 1000.000000000000000 ) ;
#30960=ORIENTED_EDGE ( 'NONE', *, *, #7938, .F. ) ;
#30967=ADVANCED_FACE ( 'NONE', ( #25878 ), #23213, .F. ) ;
#30970=VECTOR ( 'NONE', #30136, 1000.000000000000000 ) ;
#30977=EDGE_CURVE ( 'NONE', #594, #9940, #26836, .T. ) ;
#30978=LINE ( 'NONE', #3209, #24317 ) ;
#30981=DIRECTION ( 'NONE',  ( -1.000000000000000000, 6.792721752314501023E-48, -3.697785493223492838E-32 ) ) ;
#30983=ORIENTED_EDGE ( 'NONE', *, *, #29097, .F. ) ;
#30992=LINE ( 'NONE', #34005, #30778 ) ;
#30995=AXIS2_PLACEMENT_3D ( 'NONE', #1126, #11992, #23017 ) ;
#30998=VERTEX_POINT ( 'NONE', #13188 ) ;
#31000=FACE_OUTER_BOUND ( 'NONE', #31034, .T. ) ;
#31001=PLANE ( 'NONE',  #30213 ) ;
#31002=DIRECTION ( 'NONE',  ( -0.000000000000000000, 1.836970198721029934E-16, -1.000000000000000000 ) ) ;
#31003=DIRECTION ( 'NONE',  ( -0.000000000000000000, -1.836970198721029688E-16, 1.000000000000000000 ) ) ;
#31010=VERTEX_POINT ( 'NONE', #6993 ) ;
#31016=EDGE_CURVE ( 'NONE', #29402, #22892, #20617, .T. ) ;
#31024=ORIENTED_EDGE ( 'NONE', *, *, #13147, .F. ) ;
#31028=VECTOR ( 'NONE', #4313, 1000.000000000000000 ) ;
#31033=VERTEX_POINT ( 'NONE', #19065 ) ;
#31034=EDGE_LOOP ( 'NONE', ( #10914, #8691, #15579, #34255 ) ) ;
#31037=VECTOR ( 'NONE', #7699, 1000.000000000000114 ) ;
#31038=ADVANCED_FACE ( 'NONE', ( #3540 ), #27401, .F. ) ;
#31039=CARTESIAN_POINT ( 'NONE',  ( -12.25939112814508825, 30.14816249862102637, 68.31122994652405112 ) ) ;
#31041=CARTESIAN_POINT ( 'NONE',  ( -23.93921925319781963, 29.33115633223347274, -36.68877005347593467 ) ) ;
#31044=LINE ( 'NONE', #14506, #24761 ) ;
#31048=LINE ( 'NONE', #33358, #32512 ) ;
#31049=DIRECTION ( 'NONE',  ( 0.000000000000000000, 1.000000000000000000, 1.836970198721029688E-16 ) ) ;
#31054=DIRECTION ( 'NONE',  ( -0.000000000000000000, 1.836970198721029934E-16, -1.000000000000000000 ) ) ;
#31057=DIRECTION ( 'NONE',  ( 0.6051742151937647973, 0.7960930657056438653, 0.000000000000000000 ) ) ;
#31060=ORIENTED_EDGE ( 'NONE', *, *, #18809, .T. ) ;
#31062=LINE ( 'NONE', #9346, #14896 ) ;
#31065=EDGE_CURVE ( 'NONE', #17606, #4766, #16925, .T. ) ;
#31068=ORIENTED_EDGE ( 'NONE', *, *, #34307, .F. ) ;
#31084=DIRECTION ( 'NONE',  ( 0.000000000000000000, 1.836970198721029688E-16, -1.000000000000000000 ) ) ;
#31086=CARTESIAN_POINT ( 'NONE',  ( -27.84632068199329780, 25.66368763279034226, 68.31122994652405112 ) ) ;
#31088=DIRECTION ( 'NONE',  ( 0.000000000000000000, 1.836970198721029688E-16, -1.000000000000000000 ) ) ;
#31089=CARTESIAN_POINT ( 'NONE',  ( 10.62930655775863364, -36.34639295086970634, -36.68877005347593467 ) ) ;
#31096=ORIENTED_EDGE ( 'NONE', *, *, #23547, .T. ) ;
#31101=ADVANCED_FACE ( 'NONE', ( #180 ), #19762, .F. ) ;
#31114=CARTESIAN_POINT ( 'NONE',  ( 30.69344702212033127, -10.82204614554912681, 68.31122994652405112 ) ) ;
#31119=EDGE_CURVE ( 'NONE', #16921, #21448, #5848, .T. ) ;
#31122=ORIENTED_EDGE ( 'NONE', *, *, #3805, .F. ) ;
#31123=ORIENTED_EDGE ( 'NONE', *, *, #6772, .T. ) ;
#31126=VECTOR ( 'NONE', #19533, 1000.000000000000227 ) ;
#31130=CARTESIAN_POINT ( 'NONE',  ( -20.02113311122478123, 16.12922284503173742, -67.50000000000000000 ) ) ;
#31131=FACE_OUTER_BOUND ( 'NONE', #23989, .T. ) ;
#31132=VERTEX_POINT ( 'NONE', #13705 ) ;
#31137=LINE ( 'NONE', #25781, #6395 ) ;
#31153=EDGE_CURVE ( 'NONE', #319, #9821, #16571, .T. ) ;
#31154=ORIENTED_EDGE ( 'NONE', *, *, #12068, .F. ) ;
#31158=CARTESIAN_POINT ( 'NONE',  ( -31.68358972719163091, 7.440061483287550459, -36.68877005347593467 ) ) ;
#31163=LINE ( 'NONE', #9966, #11629 ) ;
#31165=VECTOR ( 'NONE', #30847, 1000.000000000000227 ) ;
#31168=CARTESIAN_POINT ( 'NONE',  ( 15.44711578872682445, -28.64595934308655600, 49.43553178847298568 ) ) ;
#31189=VECTOR ( 'NONE', #3002, 1000.000000000000114 ) ;
#31209=LINE ( 'NONE', #7327, #9164 ) ;
#31210=ORIENTED_EDGE ( 'NONE', *, *, #28224, .F. ) ;
#31222=CARTESIAN_POINT ( 'NONE',  ( -29.34345171400087793, 14.07715221144534823, 68.31122994652405112 ) ) ;
#31224=EDGE_CURVE ( 'NONE', #19647, #23009, #31137, .T. ) ;
#31233=CARTESIAN_POINT ( 'NONE',  ( 0.000000000000000000, -33.69708579775584667, 49.43553178847298568 ) ) ;
#31234=ORIENTED_EDGE ( 'NONE', *, *, #3073, .T. ) ;
#31235=VECTOR ( 'NONE', #29098, 1000.000000000000000 ) ;
#31238=VERTEX_POINT ( 'NONE', #17628 ) ;
#31241=CYLINDRICAL_SURFACE ( 'NONE', #8788, 2.033421858999710619 ) ;
#31244=EDGE_LOOP ( 'NONE', ( #6293, #1954, #24894, #24638 ) ) ;
#31245=ORIENTED_EDGE ( 'NONE', *, *, #24364, .F. ) ;
#31248=FACE_OUTER_BOUND ( 'NONE', #12517, .T. ) ;
#31265=CARTESIAN_POINT ( 'NONE',  ( 31.73435513276359643, 7.220462394039750542, 68.31122994652405112 ) ) ;
#31268=ORIENTED_EDGE ( 'NONE', *, *, #32090, .F. ) ;
#31275=VECTOR ( 'NONE', #14969, 999.9999999999998863 ) ;
#31282=CARTESIAN_POINT ( 'NONE',  ( -35.00000000000000000, -4.184937238521373004, 15.81122994652407776 ) ) ;
#31286=ORIENTED_EDGE ( 'NONE', *, *, #33626, .F. ) ;
#31287=CARTESIAN_POINT ( 'NONE',  ( -18.38714294329533416, -33.09555747561021377, 68.31122994652405112 ) ) ;
#31289=PLANE ( 'NONE',  #29269 ) ;
#31290=LINE ( 'NONE', #4225, #10913 ) ;
#31292=ORIENTED_EDGE ( 'NONE', *, *, #19869, .T. ) ;
#31309=ORIENTED_EDGE ( 'NONE', *, *, #13147, .T. ) ;
#31321=DIRECTION ( 'NONE',  ( 3.970546015203020284E-16, 0.000000000000000000, -1.000000000000000000 ) ) ;
#31324=EDGE_CURVE ( 'NONE', #5728, #29028, #12625, .T. ) ;
#31327=AXIS2_PLACEMENT_3D ( 'NONE', #13881, #8882, #27924 ) ;
#31330=LINE ( 'NONE', #14458, #7755 ) ;
#31333=EDGE_CURVE ( 'NONE', #33608, #24529, #26297, .T. ) ;
#31345=FACE_OUTER_BOUND ( 'NONE', #22030, .T. ) ;
#31354=SHAPE_REPRESENTATION_RELATIONSHIP ( 'NONE' , 'NONE' ,  #30518, #7549 ) ;
#31359=ORIENTED_EDGE ( 'NONE', *, *, #17553, .T. ) ;
#31363=ORIENTED_EDGE ( 'NONE', *, *, #1972, .F. ) ;
#31364=LINE ( 'NONE', #9310, #12816 ) ;
#31368=VERTEX_POINT ( 'NONE', #23818 ) ;
#31369=DIRECTION ( 'NONE',  ( 0.000000000000000000, 1.836970198721029441E-16, -1.000000000000000000 ) ) ;
#31371=ORIENTED_EDGE ( 'NONE', *, *, #23900, .T. ) ;
#31375=DIRECTION ( 'NONE',  ( -0.9075754196709567845, -0.4198891015602652099, -7.713237663339549565E-17 ) ) ;
#31376=LINE ( 'NONE', #4136, #27894 ) ;
#31381=CARTESIAN_POINT ( 'NONE',  ( -32.37866696771086339, 3.290334066652078171, 68.31122994652405112 ) ) ;
#31388=FACE_OUTER_BOUND ( 'NONE', #10496, .T. ) ;
#31390=CARTESIAN_POINT ( 'NONE',  ( -0.01189939958579078194, -1.353540050145433327, -8.257405511687798239 ) ) ;
#31394=DIRECTION ( 'NONE',  ( -0.8835120444460224931, -0.4684084406997908179, -0.000000000000000000 ) ) ;
#31406=VECTOR ( 'NONE', #9556, 1000.000000000000000 ) ;
#31410=VERTEX_POINT ( 'NONE', #29339 ) ;
#31413=ADVANCED_FACE ( 'NONE', ( #20799 ), #24024, .T. ) ;
#31414=EDGE_CURVE ( 'NONE', #19961, #736, #10651, .T. ) ;
#31422=LINE ( 'NONE', #31086, #22121 ) ;
#31423=LINE ( 'NONE', #23921, #11428 ) ;
#31425=CARTESIAN_POINT ( 'NONE',  ( -29.68486519896224962, 23.49918569563710946, 68.31122994652405112 ) ) ;
#31427=ORIENTED_EDGE ( 'NONE', *, *, #12859, .T. ) ;
#31429=CARTESIAN_POINT ( 'NONE',  ( 0.000000000000000000, 2.281310696040539424E-14, -36.68877005347592757 ) ) ;
#31430=LINE ( 'NONE', #17935, #28003 ) ;
#31432=VECTOR ( 'NONE', #23779, 1000.000000000000114 ) ;
#31435=ORIENTED_EDGE ( 'NONE', *, *, #11212, .F. ) ;
#31454=CARTESIAN_POINT ( 'NONE',  ( 15.04122381213380066, 28.86114964982165887, 49.43553178847298568 ) ) ;
#31457=ORIENTED_EDGE ( 'NONE', *, *, #9824, .F. ) ;
#31460=ORIENTED_EDGE ( 'NONE', *, *, #18031, .T. ) ;
#31466=LINE ( 'NONE', #5100, #14627 ) ;
#31476=PLANE ( 'NONE',  #2384 ) ;
#31480=VECTOR ( 'NONE', #34502, 1000.000000000000000 ) ;
#31481=CARTESIAN_POINT ( 'NONE',  ( 0.000000000000000000, 2.281310696040539424E-14, -36.68877005347592757 ) ) ;
#31484=ORIENTED_EDGE ( 'NONE', *, *, #21902, .F. ) ;
#31489=DIRECTION ( 'NONE',  ( 3.697785493223492838E-32, 1.934419779023891545E-16, -1.000000000000000000 ) ) ;
#31501=ORIENTED_EDGE ( 'NONE', *, *, #21535, .F. ) ;
#31502=ORIENTED_EDGE ( 'NONE', *, *, #29605, .T. ) ;
#31507=ORIENTED_EDGE ( 'NONE', *, *, #1881, .T. ) ;
#31511=ORIENTED_EDGE ( 'NONE', *, *, #8679, .T. ) ;
#31512=DIRECTION ( 'NONE',  ( -1.000000000000000000, 0.000000000000000000, 0.000000000000000000 ) ) ;
#31514=CARTESIAN_POINT ( 'NONE',  ( 0.000000000000000000, 3.524919873834583163E-15, 68.31122994652405112 ) ) ;
#31515=LINE ( 'NONE', #23333, #7460 ) ;
#31516=EDGE_CURVE ( 'NONE', #14788, #17615, #19718, .T. ) ;
#31519=DIRECTION ( 'NONE',  ( -0.000000000000000000, 1.836970198721029934E-16, -1.000000000000000000 ) ) ;
#31524=VECTOR ( 'NONE', #18531, 1000.000000000000000 ) ;
#31527=AXIS2_PLACEMENT_3D ( 'NONE', #24944, #578, #6072 ) ;
#31542=VERTEX_POINT ( 'NONE', #22029 ) ;
#31548=CARTESIAN_POINT ( 'NONE',  ( 1.532562817202168137, 33.69708579775584667, 49.43553178847298568 ) ) ;
#31552=ORIENTED_EDGE ( 'NONE', *, *, #4993, .F. ) ;
#31560=CARTESIAN_POINT ( 'NONE',  ( -35.00000000000000000, 3.353962854566122864, 15.81122994652406355 ) ) ;
#31562=LINE ( 'NONE', #26213, #9908 ) ;
#31565=ORIENTED_EDGE ( 'NONE', *, *, #23235, .T. ) ;
#31567=DIRECTION ( 'NONE',  ( 0.000000000000000000, 1.836970198721029688E-16, -1.000000000000000000 ) ) ;
#31570=EDGE_CURVE ( 'NONE', #21613, #7363, #30569, .T. ) ;
#31571=VECTOR ( 'NONE', #21652, 1000.000000000000000 ) ;
#31584=VECTOR ( 'NONE', #19812, 1000.000000000000000 ) ;
#31596=CIRCLE ( 'NONE', #16273, 2.033421858999711951 ) ;
#31605=LINE ( 'NONE', #26441, #31432 ) ;
#31609=CARTESIAN_POINT ( 'NONE',  ( -18.07349068442141515, -27.06572199953722446, 68.31122994652405112 ) ) ;
#31610=AXIS2_PLACEMENT_3D ( 'NONE', #29115, #18279, #10251 ) ;
#31613=EDGE_CURVE ( 'NONE', #18651, #7619, #12064, .T. ) ;
#31618=VECTOR ( 'NONE', #11962, 999.9999999999998863 ) ;
#31644=ORIENTED_EDGE ( 'NONE', *, *, #1015, .T. ) ;
#31645=DIRECTION ( 'NONE',  ( 0.000000000000000000, 1.836970198721029934E-16, -1.000000000000000000 ) ) ;
#31647=PLANE ( 'NONE',  #11036 ) ;
#31650=VECTOR ( 'NONE', #30182, 1000.000000000000000 ) ;
#31651=CARTESIAN_POINT ( 'NONE',  ( -32.32899628990712415, -3.747048406849347035, -36.68877005347593467 ) ) ;
#31652=PLANE ( 'NONE',  #9781 ) ;
#31653=ADVANCED_FACE ( 'NONE', ( #25926 ), #6861, .F. ) ;
#31654=ORIENTED_EDGE ( 'NONE', *, *, #21108, .T. ) ;
#31658=EDGE_CURVE ( 'NONE', #24529, #15307, #28423, .T. ) ;
#31659=CARTESIAN_POINT ( 'NONE',  ( 8.927936315454026328, -31.29690601358700519, 68.31122994652405112 ) ) ;
#31662=LINE ( 'NONE', #33334, #9916 ) ;
#31666=VECTOR ( 'NONE', #21488, 1000.000000000000114 ) ;
#31668=DIRECTION ( 'NONE',  ( -0.000000000000000000, 0.000000000000000000, 1.000000000000000000 ) ) ;
#31671=LINE ( 'NONE', #15685, #1547 ) ;
#31684=FACE_OUTER_BOUND ( 'NONE', #7200, .T. ) ;
#31687=VECTOR ( 'NONE', #27337, 1000.000000000000000 ) ;
#31689=CARTESIAN_POINT ( 'NONE',  ( -5.021133111224782120, 14.09580098603202813, -87.50000000000000000 ) ) ;
#31694=AXIS2_PLACEMENT_3D ( 'NONE', #13437, #2046, #10230 ) ;
#31701=AXIS2_PLACEMENT_3D ( 'NONE', #26945, #70, #24265 ) ;
#31704=VERTEX_POINT ( 'NONE', #23262 ) ;
#31705=ORIENTED_EDGE ( 'NONE', *, *, #12622, .T. ) ;
#31710=ORIENTED_EDGE ( 'NONE', *, *, #872, .F. ) ;
#31719=FACE_OUTER_BOUND ( 'NONE', #22043, .T. ) ;
#31721=ORIENTED_EDGE ( 'NONE', *, *, #20488, .F. ) ;
#31722=VECTOR ( 'NONE', #28100, 1000.000000000000000 ) ;
#31725=ORIENTED_EDGE ( 'NONE', *, *, #13986, .F. ) ;
#31745=CARTESIAN_POINT ( 'NONE',  ( 12.46788440507149964, 30.06253867087536946, 68.31122994652405112 ) ) ;
#31751=VECTOR ( 'NONE', #29713, 1000.000000000000114 ) ;
#31752=CARTESIAN_POINT ( 'NONE',  ( 10.96230482721425403, -12.47301499840863848, -87.50000000000000000 ) ) ;
#31758=CARTESIAN_POINT ( 'NONE',  ( 4.815661544189684840, -32.18716788982705168, 68.31122994652405112 ) ) ;
#31762=EDGE_LOOP ( 'NONE', ( #4962, #18514, #26306, #23445 ) ) ;
#31763=EDGE_CURVE ( 'NONE', #19439, #29430, #12142, .T. ) ;
#31774=VERTEX_POINT ( 'NONE', #15257 ) ;
#31776=DIRECTION ( 'NONE',  ( -0.000000000000000000, -1.836970198721029688E-16, 1.000000000000000000 ) ) ;
#31778=DIRECTION ( 'NONE',  ( -1.000000000000000000, -0.000000000000000000, -0.000000000000000000 ) ) ;
#31781=CARTESIAN_POINT ( 'NONE',  ( 0.000000000000000000, 3.524919873834583163E-15, 68.31122994652405112 ) ) ;
#31782=VECTOR ( 'NONE', #26907, 1000.000000000000000 ) ;
#31783=EDGE_LOOP ( 'NONE', ( #3341, #17310, #11024, #2622 ) ) ;
#31791=EDGE_LOOP ( 'NONE', ( #34302, #21731 ) ) ;
#31800=ORIENTED_EDGE ( 'NONE', *, *, #18264, .F. ) ;
#31803=CARTESIAN_POINT ( 'NONE',  ( -9.978866888775426602, 16.12922284503173742, -67.50000000000000000 ) ) ;
#31804=EDGE_CURVE ( 'NONE', #3430, #31033, #4531, .T. ) ;
#31805=EDGE_CURVE ( 'NONE', #1194, #19968, #34814, .T. ) ;
#31807=AXIS2_PLACEMENT_3D ( 'NONE', #3048, #13920, #24762 ) ;
#31808=PLANE ( 'NONE',  #9764 ) ;
#31811=DIRECTION ( 'NONE',  ( 0.000000000000000000, 1.000000000000000000, 0.000000000000000000 ) ) ;
#31815=DIRECTION ( 'NONE',  ( 0.000000000000000000, 1.000000000000000000, 0.000000000000000000 ) ) ;
#31819=CONICAL_SURFACE ( 'NONE', #5667, 32.54542015209054995, 1.389864428407444175 ) ;
#31823=DIRECTION ( 'NONE',  ( 1.000000000000000000, 0.000000000000000000, -0.000000000000000000 ) ) ;
#31824=ORIENTED_EDGE ( 'NONE', *, *, #17870, .F. ) ;
#31827=ORIENTED_EDGE ( 'NONE', *, *, #12660, .F. ) ;
#31828=CARTESIAN_POINT ( 'NONE',  ( 1.991296462759137853, -32.48444414290483451, 68.31122994652405112 ) ) ;
#31834=EDGE_CURVE ( 'NONE', #23118, #28220, #7924, .T. ) ;
#31835=EDGE_CURVE ( 'NONE', #8890, #24034, #31605, .T. ) ;
#31840=CARTESIAN_POINT ( 'NONE',  ( -21.41424479178918361, -24.50784553716277969, -36.68877005347593467 ) ) ;
#31849=VERTEX_POINT ( 'NONE', #10248 ) ;
#31856=CARTESIAN_POINT ( 'NONE',  ( 5.390701026406702567, -37.47456861236020131, 68.31122994652405112 ) ) ;
#31873=PLANE ( 'NONE',  #5945 ) ;
#31881=VECTOR ( 'NONE', #6637, 1000.000000000000000 ) ;
#31882=LINE ( 'NONE', #13048, #14711 ) ;
#31886=DIRECTION ( 'NONE',  ( 0.3701381553399144542, -0.9289767198167915296, -1.706502549609061741E-16 ) ) ;
#31890=DIRECTION ( 'NONE',  ( 3.697785493223492838E-32, 1.934419779023891545E-16, -1.000000000000000000 ) ) ;
#31895=EDGE_CURVE ( 'NONE', #640, #31947, #7742, .T. ) ;
#31900=VECTOR ( 'NONE', #27890, 1000.000000000000000 ) ;
#31905=AXIS2_PLACEMENT_3D ( 'NONE', #7468, #26167, #1788 ) ;
#31907=CARTESIAN_POINT ( 'NONE',  ( -30.58418286738120884, -22.31615353445080174, 68.31122994652405112 ) ) ;
#31910=ORIENTED_EDGE ( 'NONE', *, *, #16538, .T. ) ;
#31911=CIRCLE ( 'NONE', #17677, 2.033421858999711951 ) ;
#31913=EDGE_LOOP ( 'NONE', ( #33678, #6382, #25491, #25132 ) ) ;
#31926=DIRECTION ( 'NONE',  ( 0.000000000000000000, 1.000000000000000000, 0.000000000000000000 ) ) ;
#31930=EDGE_CURVE ( 'NONE', #6016, #15632, #33183, .T. ) ;
#31934=ORIENTED_EDGE ( 'NONE', *, *, #27562, .F. ) ;
#31942=DIRECTION ( 'NONE',  ( 0.9941379571543595972, -0.1081190184239417262, -1.986114147597509048E-17 ) ) ;
#31947=VERTEX_POINT ( 'NONE', #10782 ) ;
#31952=AXIS2_PLACEMENT_3D ( 'NONE', #25218, #8675, #5816 ) ;
#31953=CIRCLE ( 'NONE', #5802, 44.99999999999997868 ) ;
#31954=EDGE_LOOP ( 'NONE', ( #20699, #11990, #28947, #5035 ) ) ;
#31955=( GEOMETRIC_REPRESENTATION_CONTEXT ( 3 ) GLOBAL_UNCERTAINTY_ASSIGNED_CONTEXT ( ( #33809 ) ) GLOBAL_UNIT_ASSIGNED_CONTEXT ( ( #16805, #14118, #27803 ) ) REPRESENTATION_CONTEXT ( 'NONE', 'WORKASPACE' ) );
#31956=VECTOR ( 'NONE', #17030, 1000.000000000000114 ) ;
#31960=ORIENTED_EDGE ( 'NONE', *, *, #31895, .T. ) ;
#31962=ADVANCED_FACE ( 'NONE', ( #271 ), #5587, .T. ) ;
#31977=CARTESIAN_POINT ( 'NONE',  ( -37.58721499952019940, -4.609089608337754385, 68.31122994652405112 ) ) ;
#31983=EDGE_CURVE ( 'NONE', #4316, #2764, #24453, .T. ) ;
#31999=CARTESIAN_POINT ( 'NONE',  ( -29.34345171400088859, 14.07715221144535533, 68.31122994652405112 ) ) ;
#32000=DIRECTION ( 'NONE',  ( 0.000000000000000000, 0.000000000000000000, -1.000000000000000000 ) ) ;
#32002=ADVANCED_FACE ( 'NONE', ( #22332 ), #8094, .F. ) ;
#32010=EDGE_CURVE ( 'NONE', #29274, #736, #32826, .T. ) ;
#32016=ADVANCED_FACE ( 'NONE', ( #452 ), #27666, .F. ) ;
#32017=DIRECTION ( 'NONE',  ( 0.000000000000000000, 0.000000000000000000, 1.000000000000000000 ) ) ;
#32023=CARTESIAN_POINT ( 'NONE',  ( 5.021133111224473033, 8.235406450278427215, -67.50000000000000000 ) ) ;
#32025=LINE ( 'NONE', #21366, #1678 ) ;
#32030=VECTOR ( 'NONE', #18974, 1000.000000000000114 ) ;
#32032=DIRECTION ( 'NONE',  ( -0.3193015301359797276, -0.9476531711828024562, 0.000000000000000000 ) ) ;
#32035=PLANE ( 'NONE',  #456 ) ;
#32049=ORIENTED_EDGE ( 'NONE', *, *, #8693, .F. ) ;
#32056=ORIENTED_EDGE ( 'NONE', *, *, #34557, .F. ) ;
#32057=DIRECTION ( 'NONE',  ( 0.000000000000000000, 0.000000000000000000, 1.000000000000000000 ) ) ;
#32064=EDGE_LOOP ( 'NONE', ( #9124, #444, #19332, #33514 ) ) ;
#32066=CARTESIAN_POINT ( 'NONE',  ( 3.235562306570555532E-30, -1.691831803474591833, -67.50000000000000000 ) ) ;
#32068=FACE_OUTER_BOUND ( 'NONE', #34947, .T. ) ;
#32079=CARTESIAN_POINT ( 'NONE',  ( -45.00000000000000000, -38.34433698000722046, 36.69637551990492597 ) ) ;
#32085=ORIENTED_EDGE ( 'NONE', *, *, #33580, .T. ) ;
#32090=EDGE_CURVE ( 'NONE', #13032, #27734, #34898, .T. ) ;
#32094=EDGE_CURVE ( 'NONE', #19171, #19439, #6291, .T. ) ;
#32098=FACE_BOUND ( 'NONE', #17361, .T. ) ;
#32099=ORIENTED_EDGE ( 'NONE', *, *, #27606, .F. ) ;
#32101=DIRECTION ( 'NONE',  ( -0.1081190184239421009, 0.9941379571543595972, 0.000000000000000000 ) ) ;
#32104=CARTESIAN_POINT ( 'NONE',  ( -37.69926482250235722, 3.578808500140884252, -36.68877005347593467 ) ) ;
#32106=DIRECTION ( 'NONE',  ( 0.000000000000000000, 1.000000000000000000, 0.000000000000000000 ) ) ;
#32108=ORIENTED_EDGE ( 'NONE', *, *, #16323, .T. ) ;
#32125=CARTESIAN_POINT ( 'NONE',  ( 0.000000000000000000, 2.281310696040539424E-14, -36.68877005347592757 ) ) ;
#32128=VECTOR ( 'NONE', #1661, 1000.000000000000000 ) ;
#32136=ORIENTED_EDGE ( 'NONE', *, *, #9403, .F. ) ;
#32142=VECTOR ( 'NONE', #30120, 1000.000000000000000 ) ;
#32145=EDGE_CURVE ( 'NONE', #26960, #32615, #4150, .T. ) ;
#32148=VERTEX_POINT ( 'NONE', #25523 ) ;
#32149=DIRECTION ( 'NONE',  ( -0.000000000000000000, -1.836970198721029688E-16, 1.000000000000000000 ) ) ;
#32151=CARTESIAN_POINT ( 'NONE',  ( -20.02113311122488781, 6.201984591278717041, -67.50000000000000000 ) ) ;
#32158=ORIENTED_EDGE ( 'NONE', *, *, #31804, .F. ) ;
#32165=CARTESIAN_POINT ( 'NONE',  ( -35.00000000000000000, 0.5883377166428923610, 68.31122994652405112 ) ) ;
#32167=DIRECTION ( 'NONE',  ( -0.000000000000000000, -0.000000000000000000, -1.000000000000000000 ) ) ;
#32171=DIRECTION ( 'NONE',  ( 0.000000000000000000, 1.836970198721029441E-16, -1.000000000000000000 ) ) ;
#32172=CARTESIAN_POINT ( 'NONE',  ( 0.000000000000000000, 3.524919873834583163E-15, 68.31122994652405112 ) ) ;
#32185=CARTESIAN_POINT ( 'NONE',  ( -28.00450684652666311, 16.58167570419055892, -36.68877005347593467 ) ) ;
#32194=ORIENTED_EDGE ( 'NONE', *, *, #25842, .F. ) ;
#32202=VECTOR ( 'NONE', #28364, 1000.000000000000227 ) ;
#32207=CARTESIAN_POINT ( 'NONE',  ( -23.46927268871044348, -22.54767421130283012, -36.68877005347593467 ) ) ;
#32208=ORIENTED_EDGE ( 'NONE', *, *, #26760, .F. ) ;
#32209=ADVANCED_FACE ( 'NONE', ( #23893 ), #20720, .F. ) ;
#32211=CARTESIAN_POINT ( 'NONE',  ( -36.80830595996284416, 8.862931941313782147, 24.65111515542800547 ) ) ;
#32212=EDGE_LOOP ( 'NONE', ( #30544, #17214, #25587, #22246 ) ) ;
#32218=EDGE_LOOP ( 'NONE', ( #16231, #8119, #33272, #25726 ) ) ;
#32223=DIRECTION ( 'NONE',  ( 0.000000000000000000, -1.000000000000000000, 0.000000000000000000 ) ) ;
#32224=CARTESIAN_POINT ( 'NONE',  ( -27.13361903382165963, -26.41607761506757868, 68.31122994652405112 ) ) ;
#32226=DIRECTION ( 'NONE',  ( -0.000000000000000000, 1.836970198721029688E-16, -1.000000000000000000 ) ) ;
#32241=CARTESIAN_POINT ( 'NONE',  ( -23.46927268871045058, -22.54767421130284077, 68.31122994652405112 ) ) ;
#32244=ORIENTED_EDGE ( 'NONE', *, *, #4751, .T. ) ;
#32251=EDGE_CURVE ( 'NONE', #29816, #27865, #2019, .T. ) ;
#32254=AXIS2_PLACEMENT_3D ( 'NONE', #16437, #25115, #19280 ) ;
#32255=DIRECTION ( 'NONE',  ( 0.8835120444460227151, -0.4684084406997903183, 0.000000000000000000 ) ) ;
#32263=DIRECTION ( 'NONE',  ( -0.000000000000000000, 1.836970198721029934E-16, -1.000000000000000000 ) ) ;
#32266=CARTESIAN_POINT ( 'NONE',  ( -5.021133111224989953, -3.725253662474300231, -87.50000000000000000 ) ) ;
#32267=CARTESIAN_POINT ( 'NONE',  ( -45.00000000000000000, 0.000000000000000000, 0.000000000000000000 ) ) ;
#32269=VERTEX_POINT ( 'NONE', #26218 ) ;
#32272=CIRCLE ( 'NONE', #29439, 2.033421858999711951 ) ;
#32277=VERTEX_POINT ( 'NONE', #21059 ) ;
#32279=CARTESIAN_POINT ( 'NONE',  ( -9.978866888775733912, -11.61907005722761532, -67.50000000000000000 ) ) ;
#32297=LINE ( 'NONE', #17627, #10078 ) ;
#32298=EDGE_LOOP ( 'NONE', ( #22764, #27100, #12924, #8016 ) ) ;
#32303=DIRECTION ( 'NONE',  ( 0.000000000000000000, 0.000000000000000000, 1.000000000000000000 ) ) ;
#32304=ORIENTED_EDGE ( 'NONE', *, *, #232, .F. ) ;
#32306=FACE_OUTER_BOUND ( 'NONE', #13684, .T. ) ;
#32331=CIRCLE ( 'NONE', #7296, 32.54542015209056416 ) ;
#32337=EDGE_CURVE ( 'NONE', #17138, #4500, #29064, .T. ) ;
#32341=DIRECTION ( 'NONE',  ( 0.000000000000000000, 1.000000000000000000, 0.000000000000000000 ) ) ;
#32343=VECTOR ( 'NONE', #11251, 1000.000000000000000 ) ;
#32346=ORIENTED_EDGE ( 'NONE', *, *, #11704, .F. ) ;
#32350=AXIS2_PLACEMENT_3D ( 'NONE', #24041, #13215, #3823 ) ;
#32351=ORIENTED_EDGE ( 'NONE', *, *, #31804, .T. ) ;
#32353=CARTESIAN_POINT ( 'NONE',  ( 3.235562306570555532E-30, -5.758675521474015291, -67.50000000000000000 ) ) ;
#32355=ORIENTED_EDGE ( 'NONE', *, *, #7180, .F. ) ;
#32359=CARTESIAN_POINT ( 'NONE',  ( 31.83311414508813897, -6.771795677801486057, 68.31122994652405112 ) ) ;
#32360=VERTEX_POINT ( 'NONE', #4494 ) ;
#32361=DIRECTION ( 'NONE',  ( -0.000000000000000000, 1.836970198721029934E-16, -1.000000000000000000 ) ) ;
#32372=ORIENTED_EDGE ( 'NONE', *, *, #8282, .T. ) ;
#32375=LINE ( 'NONE', #18706, #31189 ) ;
#32381=DIRECTION ( 'NONE',  ( -0.000000000000000000, -0.000000000000000000, -1.000000000000000000 ) ) ;
#32385=VERTEX_POINT ( 'NONE', #13587 ) ;
#32392=FACE_OUTER_BOUND ( 'NONE', #6920, .T. ) ;
#32394=EDGE_CURVE ( 'NONE', #20123, #5102, #10912, .T. ) ;
#32395=ORIENTED_EDGE ( 'NONE', *, *, #32145, .F. ) ;
#32399=VERTEX_POINT ( 'NONE', #16268 ) ;
#32411=DIRECTION ( 'NONE',  ( 0.000000000000000000, 1.000000000000000000, 0.000000000000000000 ) ) ;
#32413=VERTEX_POINT ( 'NONE', #29598 ) ;
#32415=CARTESIAN_POINT ( 'NONE',  ( -12.25939112814508825, 30.14816249862104769, -36.68877005347593467 ) ) ;
#32419=CARTESIAN_POINT ( 'NONE',  ( -9.978866888775733912, -13.65249191622732461, -87.50000000000000000 ) ) ;
#32422=PLANE ( 'NONE',  #15152 ) ;
#32424=ADVANCED_FACE ( 'NONE', ( #5196 ), #16443, .F. ) ;
#32430=CARTESIAN_POINT ( 'NONE',  ( 26.04754872656010178, -19.51229300245306320, 68.31122994652405112 ) ) ;
#32432=ORIENTED_EDGE ( 'NONE', *, *, #3450, .F. ) ;
#32435=ORIENTED_EDGE ( 'NONE', *, *, #31658, .F. ) ;
#32442=EDGE_LOOP ( 'NONE', ( #6596, #26758, #22261, #24228 ) ) ;
#32443=PLANE ( 'NONE',  #16186 ) ;
#32452=VERTEX_POINT ( 'NONE', #19116 ) ;
#32457=LINE ( 'NONE', #24094, #2875 ) ;
#32459=CARTESIAN_POINT ( 'NONE',  ( -35.00000000000000000, 3.353962854566122864, 15.81122994652406355 ) ) ;
#32461=DIRECTION ( 'NONE',  ( 0.000000000000000000, 1.836970198721029688E-16, -1.000000000000000000 ) ) ;
#32478=CARTESIAN_POINT ( 'NONE',  ( -34.04247984038124031, 16.56841925338180488, 68.31122994652405112 ) ) ;
#32479=CARTESIAN_POINT ( 'NONE',  ( 3.235562306570555532E-30, -5.758675521474015291, -67.50000000000000000 ) ) ;
#32481=ORIENTED_EDGE ( 'NONE', *, *, #18677, .F. ) ;
#32483=VECTOR ( 'NONE', #21943, 1000.000000000000000 ) ;
#32485=VECTOR ( 'NONE', #22083, 1000.000000000000114 ) ;
#32486=ORIENTED_EDGE ( 'NONE', *, *, #13949, .F. ) ;
#32488=CARTESIAN_POINT ( 'NONE',  ( -18.45373714011839539, 26.80790850550480542, 68.31122994652405112 ) ) ;
#32505=DIRECTION ( 'NONE',  ( 1.000000000000000000, 0.000000000000000000, 0.000000000000000000 ) ) ;
#32512=VECTOR ( 'NONE', #30863, 1000.000000000000000 ) ;
#32513=CIRCLE ( 'NONE', #26271, 2.033421858999711951 ) ;
#32525=EDGE_CURVE ( 'NONE', #33041, #18637, #23522, .T. ) ;
#32531=EDGE_LOOP ( 'NONE', ( #30238, #3562, #21649, #32372 ) ) ;
#32534=VECTOR ( 'NONE', #5500, 1000.000000000000000 ) ;
#32539=ORIENTED_EDGE ( 'NONE', *, *, #27113, .F. ) ;
#32543=EDGE_CURVE ( 'NONE', #32705, #33757, #11625, .T. ) ;
#32550=DIRECTION ( 'NONE',  ( -0.000000000000000000, 1.836970198721029934E-16, -1.000000000000000000 ) ) ;
#32556=ORIENTED_EDGE ( 'NONE', *, *, #29558, .F. ) ;
#32558=DIRECTION ( 'NONE',  ( 0.000000000000000000, -1.836970198721030181E-16, 1.000000000000000000 ) ) ;
#32561=LINE ( 'NONE', #24205, #14588 ) ;
#32568=ORIENTED_EDGE ( 'NONE', *, *, #28641, .T. ) ;
#32569=LINE ( 'NONE', #19422, #17185 ) ;
#32575=AXIS2_PLACEMENT_3D ( 'NONE', #19851, #976, #33531 ) ;
#32580=ORIENTED_EDGE ( 'NONE', *, *, #34974, .F. ) ;
#32590=DIRECTION ( 'NONE',  ( -0.6051742151937647973, 0.7960930657056438653, 0.000000000000000000 ) ) ;
#32594=DIRECTION ( 'NONE',  ( -1.000000000000000000, 0.000000000000000000, -0.000000000000000000 ) ) ;
#32597=FACE_OUTER_BOUND ( 'NONE', #8818, .T. ) ;
#32608=CARTESIAN_POINT ( 'NONE',  ( 5.021133111224162171, -23.57973016998034765, -67.50000000000000000 ) ) ;
#32610=CARTESIAN_POINT ( 'NONE',  ( 3.235562306570555532E-30, 1.325223266901699007E-14, -67.50000000000000000 ) ) ;
#32615=VERTEX_POINT ( 'NONE', #33669 ) ;
#32623=CARTESIAN_POINT ( 'NONE',  ( 20.89386240318430055, 24.95297350523386015, 68.31122994652405112 ) ) ;
#32638=VECTOR ( 'NONE', #7515, 1000.000000000000114 ) ;
#32639=AXIS2_PLACEMENT_3D ( 'NONE', #30088, #32920, #21555 ) ;
#32643=CARTESIAN_POINT ( 'NONE',  ( 15.04122381213380244, 28.86114964982166597, 68.31122994652405112 ) ) ;
#32647=DIRECTION ( 'NONE',  ( -0.000000000000000000, -0.000000000000000000, 1.000000000000000000 ) ) ;
#32650=DIRECTION ( 'NONE',  ( 0.000000000000000000, -0.000000000000000000, 1.000000000000000000 ) ) ;
#32655=EDGE_CURVE ( 'NONE', #30998, #22969, #9643, .T. ) ;
#32659=LINE ( 'NONE', #32478, #29683 ) ;
#32667=AXIS2_PLACEMENT_3D ( 'NONE', #24028, #16228, #19246 ) ;
#32669=PLANE ( 'NONE',  #1012 ) ;
#32677=PLANE ( 'NONE',  #23889 ) ;
#32679=ORIENTED_EDGE ( 'NONE', *, *, #7892, .F. ) ;
#32681=CARTESIAN_POINT ( 'NONE',  ( -20.02113311122478123, 16.12922284503174097, -87.50000000000000000 ) ) ;
#32684=AXIS2_PLACEMENT_3D ( 'NONE', #4466, #32057, #29225 ) ;
#32691=DIRECTION ( 'NONE',  ( -1.000000000000000000, 6.792721752314501023E-48, -3.697785493223492838E-32 ) ) ;
#32705=VERTEX_POINT ( 'NONE', #12674 ) ;
#32710=VECTOR ( 'NONE', #25013, 1000.000000000000000 ) ;
#32718=LINE ( 'NONE', #16378, #34956 ) ;
#32722=VERTEX_POINT ( 'NONE', #20497 ) ;
#32729=ORIENTED_EDGE ( 'NONE', *, *, #14235, .T. ) ;
#32737=AXIS2_PLACEMENT_3D ( 'NONE', #16290, #23551, #31926 ) ;
#32739=ADVANCED_FACE ( 'NONE', ( #23512 ), #6954, .F. ) ;
#32747=PLANE ( 'NONE',  #1779 ) ;
#32754=ORIENTED_EDGE ( 'NONE', *, *, #19794, .T. ) ;
#32761=AXIS2_PLACEMENT_3D ( 'NONE', #32818, #28018, #8447 ) ;
#32762=CARTESIAN_POINT ( 'NONE',  ( 37.71145559917817280, 3.353962854566119756, 49.43553178847298568 ) ) ;
#32765=VERTEX_POINT ( 'NONE', #32925 ) ;
#32772=CARTESIAN_POINT ( 'NONE',  ( -32.54223829851967764, 0.4550817492056196678, 15.81122994652406355 ) ) ;
#32773=CARTESIAN_POINT ( 'NONE',  ( -35.00000000000000000, -46.95407462254104303, 36.69637551990492597 ) ) ;
#32774=VERTEX_POINT ( 'NONE', #17547 ) ;
#32782=CARTESIAN_POINT ( 'NONE',  ( 22.89764159710611224, 13.56412600238610366, -77.50000000000000000 ) ) ;
#32794=ORIENTED_EDGE ( 'NONE', *, *, #13187, .F. ) ;
#32804=AXIS2_PLACEMENT_3D ( 'NONE', #20879, #34760, #21050 ) ;
#32812=CARTESIAN_POINT ( 'NONE',  ( 0.000000000000000000, 0.000000000000000000, 87.50000000000000000 ) ) ;
#32818=CARTESIAN_POINT ( 'NONE',  ( 21.85761591200894216, 30.91355005303805825, 68.31122994652405112 ) ) ;
#32822=EDGE_LOOP ( 'NONE', ( #9706, #22662, #21308, #21660 ) ) ;
#32823=AXIS2_PLACEMENT_3D ( 'NONE', #24999, #2594, #27504 ) ;
#32826=LINE ( 'NONE', #24818, #32030 ) ;
#32833=CARTESIAN_POINT ( 'NONE',  ( 36.10877985260814427, 11.38239727801116352, 49.43553178847298568 ) ) ;
#32834=DIRECTION ( 'NONE',  ( 0.9289767198167914186, 0.3701381553399144542, -0.000000000000000000 ) ) ;
#32838=ORIENTED_EDGE ( 'NONE', *, *, #20336, .F. ) ;
#32846=CARTESIAN_POINT ( 'NONE',  ( 0.000000000000000000, 2.281310696040539424E-14, -36.68877005347592757 ) ) ;
#32847=EDGE_CURVE ( 'NONE', #25253, #31542, #33711, .T. ) ;
#32855=DIRECTION ( 'NONE',  ( 0.8276889981568912313, 0.5611870653623813876, 1.030883914978405312E-16 ) ) ;
#32858=VECTOR ( 'NONE', #17816, 1000.000000000000114 ) ;
#32863=VECTOR ( 'NONE', #34167, 1000.000000000000000 ) ;
#32864=EDGE_LOOP ( 'NONE', ( #4783, #18565, #1090, #7825 ) ) ;
#32878=CARTESIAN_POINT ( 'NONE',  ( 5.021133111224369117, -1.691831803474591833, -67.50000000000000000 ) ) ;
#32880=CARTESIAN_POINT ( 'NONE',  ( 32.40067729534749219, 3.066020821660472517, 68.31122994652405112 ) ) ;
#32883=EDGE_LOOP ( 'NONE', ( #7573, #8005, #6317, #26700 ) ) ;
#32891=EDGE_CURVE ( 'NONE', #10877, #28025, #31562, .T. ) ;
#32897=EDGE_LOOP ( 'NONE', ( #27037, #16713, #24137, #20776 ) ) ;
#32899=CARTESIAN_POINT ( 'NONE',  ( 29.63313772848249883, -13.45665341906702572, 68.31122994652405112 ) ) ;
#32905=ORIENTED_EDGE ( 'NONE', *, *, #32010, .F. ) ;
#32906=DIRECTION ( 'NONE',  ( 0.000000000000000000, 0.000000000000000000, 1.000000000000000000 ) ) ;
#32915=CARTESIAN_POINT ( 'NONE',  ( 3.235562306570555532E-30, -11.61907005722761532, -67.50000000000000000 ) ) ;
#32916=CARTESIAN_POINT ( 'NONE',  ( -32.32899628990713126, -3.747048406849353697, 68.31122994652405112 ) ) ;
#32920=DIRECTION ( 'NONE',  ( 0.000000000000000000, 0.000000000000000000, 1.000000000000000000 ) ) ;
#32921=EDGE_CURVE ( 'NONE', #3404, #22677, #25699, .T. ) ;
#32925=CARTESIAN_POINT ( 'NONE',  ( -20.82057426567703473, -31.63141042832694083, 68.31122994652405112 ) ) ;
#32928=ORIENTED_EDGE ( 'NONE', *, *, #29412, .F. ) ;
#32929=EDGE_CURVE ( 'NONE', #22259, #32269, #5375, .T. ) ;
#32930=EDGE_CURVE ( 'NONE', #17595, #5551, #10909, .T. ) ;
#32936=CARTESIAN_POINT ( 'NONE',  ( -31.68358972719163091, 7.440061483287530919, 68.31122994652405112 ) ) ;
#32940=VERTEX_POINT ( 'NONE', #2016 ) ;
#32941=DIRECTION ( 'NONE',  ( 0.000000000000000000, 0.000000000000000000, 1.000000000000000000 ) ) ;
#32943=DIRECTION ( 'NONE',  ( -0.000000000000000000, 1.836970198721029688E-16, -1.000000000000000000 ) ) ;
#32960=VERTEX_POINT ( 'NONE', #13584 ) ;
#32961=EDGE_CURVE ( 'NONE', #15892, #28736, #10203, .T. ) ;
#32966=VERTEX_POINT ( 'NONE', #32079 ) ;
#32971=ORIENTED_EDGE ( 'NONE', *, *, #6212, .T. ) ;
#32973=CARTESIAN_POINT ( 'NONE',  ( -5.021133111224886036, 6.201984591278720593, -87.50000000000000000 ) ) ;
#32984=EDGE_CURVE ( 'NONE', #1890, #12135, #10741, .T. ) ;
#32985=DIRECTION ( 'NONE',  ( 0.9818488882034280829, 0.1609659548241204607, 0.1003131203843820457 ) ) ;
#32987=ORIENTED_EDGE ( 'NONE', *, *, #24153, .T. ) ;
#32990=DIRECTION ( 'NONE',  ( -0.000000000000000000, -1.836970198721029688E-16, 1.000000000000000000 ) ) ;
#32993=VECTOR ( 'NONE', #12353, 1000.000000000000000 ) ;
#32996=ORIENTED_EDGE ( 'NONE', *, *, #7340, .F. ) ;
#33005=EDGE_LOOP ( 'NONE', ( #28874, #12527, #2298, #20140 ) ) ;
#33007=FACE_OUTER_BOUND ( 'NONE', #21172, .T. ) ;
#33016=DIRECTION ( 'NONE',  ( 0.000000000000000000, 1.836970198721029441E-16, -1.000000000000000000 ) ) ;
#33018=VERTEX_POINT ( 'NONE', #34590 ) ;
#33024=AXIS2_PLACEMENT_3D ( 'NONE', #11672, #25526, #5763 ) ;
#33026=CARTESIAN_POINT ( 'NONE',  ( -35.00000000000000000, 16.36947364650383818, 36.69637551990492597 ) ) ;
#33034=PLANE ( 'NONE',  #34476 ) ;
#33036=ADVANCED_FACE ( 'NONE', ( #2355 ), #24065, .F. ) ;
#33038=LINE ( 'NONE', #30035, #9234 ) ;
#33041=VERTEX_POINT ( 'NONE', #24244 ) ;
#33042=CARTESIAN_POINT ( 'NONE',  ( -35.00000000000000000, 28.28427124746189136, -36.69637551990492597 ) ) ;
#33051=AXIS2_PLACEMENT_3D ( 'NONE', #31233, #28563, #4333 ) ;
#33058=ORIENTED_EDGE ( 'NONE', *, *, #31153, .T. ) ;
#33060=VECTOR ( 'NONE', #7240, 1000.000000000000000 ) ;
#33077=AXIS2_PLACEMENT_3D ( 'NONE', #9672, #20535, #32032 ) ;
#33081=CIRCLE ( 'NONE', #25122, 32.54542015209054284 ) ;
#33083=AXIS2_PLACEMENT_3D ( 'NONE', #25074, #3889, #25608 ) ;
#33084=DIRECTION ( 'NONE',  ( 0.000000000000000000, 1.836970198721029441E-16, -1.000000000000000000 ) ) ;
#33089=DIRECTION ( 'NONE',  ( 0.9075754196709575616, -0.4198891015602635446, 0.000000000000000000 ) ) ;
#33090=ORIENTED_EDGE ( 'NONE', *, *, #11807, .T. ) ;
#33093=FACE_OUTER_BOUND ( 'NONE', #4992, .T. ) ;
#33094=ADVANCED_FACE ( 'NONE', ( #19112 ), #19282, .F. ) ;
#33106=VECTOR ( 'NONE', #3146, 1000.000000000000000 ) ;
#33110=ORIENTED_EDGE ( 'NONE', *, *, #15657, .T. ) ;
#33113=ORIENTED_EDGE ( 'NONE', *, *, #14231, .T. ) ;
#33122=ADVANCED_FACE ( 'NONE', ( #25303 ), #30119, .T. ) ;
#33128=CARTESIAN_POINT ( 'NONE',  ( 0.000000000000000000, 3.524919873834583163E-15, 68.31122994652405112 ) ) ;
#33129=FACE_OUTER_BOUND ( 'NONE', #24464, .T. ) ;
#33130=VECTOR ( 'NONE', #15649, 1000.000000000000000 ) ;
#33133=CARTESIAN_POINT ( 'NONE',  ( 15.44711578872682267, -28.64595934308657377, 49.43553178847298568 ) ) ;
#33136=CARTESIAN_POINT ( 'NONE',  ( 35.63428259149705468, -12.79065496477506869, 49.43553178847298568 ) ) ;
#33137=EDGE_CURVE ( 'NONE', #11027, #28736, #3410, .T. ) ;
#33143=ORIENTED_EDGE ( 'NONE', *, *, #30883, .F. ) ;
#33152=VECTOR ( 'NONE', #27623, 1000.000000000000114 ) ;
#33165=DIRECTION ( 'NONE',  ( -0.000000000000000000, 1.836970198721029934E-16, -1.000000000000000000 ) ) ;
#33166=CARTESIAN_POINT ( 'NONE',  ( 0.000000000000000000, 3.524919873834583163E-15, 68.31122994652405112 ) ) ;
#33170=CARTESIAN_POINT ( 'NONE',  ( -5.021133111224989953, -5.758675521474015291, -67.50000000000000000 ) ) ;
#33173=ORIENTED_EDGE ( 'NONE', *, *, #20451, .F. ) ;
#33174=EDGE_CURVE ( 'NONE', #18486, #18999, #6243, .T. ) ;
#33183=CIRCLE ( 'NONE', #18972, 2.033421858999711951 ) ;
#33185=CARTESIAN_POINT ( 'NONE',  ( -9.978866888775527855, 6.201984591278717041, -67.50000000000000000 ) ) ;
#33190=ORIENTED_EDGE ( 'NONE', *, *, #10859, .F. ) ;
#33191=CARTESIAN_POINT ( 'NONE',  ( -32.37866696771086339, 3.290334066652079947, 68.31122994652405112 ) ) ;
#33192=FACE_OUTER_BOUND ( 'NONE', #9745, .T. ) ;
#33195=VECTOR ( 'NONE', #641, 1000.000000000000000 ) ;
#33210=VECTOR ( 'NONE', #10337, 1000.000000000000000 ) ;
#33211=CARTESIAN_POINT ( 'NONE',  ( 60.00000000000000000, -33.69708579775584667, 49.43553178847298568 ) ) ;
#33212=DIRECTION ( 'NONE',  ( 1.000000000000000000, 0.000000000000000000, 0.000000000000000000 ) ) ;
#33213=FACE_OUTER_BOUND ( 'NONE', #13566, .T. ) ;
#33219=ORIENTED_EDGE ( 'NONE', *, *, #15040, .T. ) ;
#33227=ORIENTED_EDGE ( 'NONE', *, *, #12870, .T. ) ;
#33229=CARTESIAN_POINT ( 'NONE',  ( -35.00000000000000000, 3.432458613951613557, 15.93718699791191185 ) ) ;
#33236=EDGE_CURVE ( 'NONE', #30543, #23102, #25651, .T. ) ;
#33240=CARTESIAN_POINT ( 'NONE',  ( 0.000000000000000000, 3.524919873834583163E-15, 68.31122994652405112 ) ) ;
#33242=AXIS2_PLACEMENT_3D ( 'NONE', #340, #865, #8515 ) ;
#33250=AXIS2_PLACEMENT_3D ( 'NONE', #22796, #28656, #19955 ) ;
#33257=VECTOR ( 'NONE', #10239, 1000.000000000000000 ) ;
#33264=VERTEX_POINT ( 'NONE', #9290 ) ;
#33265=VECTOR ( 'NONE', #33534, 1000.000000000000000 ) ;
#33272=ORIENTED_EDGE ( 'NONE', *, *, #28791, .T. ) ;
#33274=CARTESIAN_POINT ( 'NONE',  ( 34.58310883014599568, -15.42890216704096851, 49.43553178847298568 ) ) ;
#33278=EDGE_CURVE ( 'NONE', #319, #28991, #15166, .T. ) ;
#33284=VECTOR ( 'NONE', #4140, 1000.000000000000000 ) ;
#33285=ORIENTED_EDGE ( 'NONE', *, *, #2637, .T. ) ;
#33289=VERTEX_POINT ( 'NONE', #20495 ) ;
#33294=DIRECTION ( 'NONE',  ( 0.000000000000000000, 1.836970198721029441E-16, -1.000000000000000000 ) ) ;
#33298=EDGE_CURVE ( 'NONE', #32277, #14545, #28677, .T. ) ;
#33302=CIRCLE ( 'NONE', #22517, 32.54542015209054995 ) ;
#33307=DIRECTION ( 'NONE',  ( 0.8276889981568904542, -0.5611870653623824978, 0.000000000000000000 ) ) ;
#33309=EDGE_CURVE ( 'NONE', #22892, #7203, #13024, .T. ) ;
#33310=DIRECTION ( 'NONE',  ( 0.05413890858541543089, 0.9985334138511240409, 0.000000000000000000 ) ) ;
#33317=ORIENTED_EDGE ( 'NONE', *, *, #1589, .T. ) ;
#33320=CARTESIAN_POINT ( 'NONE',  ( 0.000000000000000000, 2.296212748401288367E-15, 47.49999999999999289 ) ) ;
#33321=LINE ( 'NONE', #17503, #7562 ) ;
#33326=CARTESIAN_POINT ( 'NONE',  ( -31.87924797510909869, -6.551177101682124970, 68.31122994652405112 ) ) ;
#33334=CARTESIAN_POINT ( 'NONE',  ( -45.00000000000000000, -4.831299144296466785, 15.81122994652406355 ) ) ;
#33345=ORIENTED_EDGE ( 'NONE', *, *, #13300, .F. ) ;
#33354=LINE ( 'NONE', #29806, #12292 ) ;
#33358=CARTESIAN_POINT ( 'NONE',  ( -28.00450684652667022, 16.58167570419054471, 68.31122994652405112 ) ) ;
#33362=VECTOR ( 'NONE', #10801, 1000.000000000000000 ) ;
#33368=ORIENTED_EDGE ( 'NONE', *, *, #150, .T. ) ;
#33370=FACE_OUTER_BOUND ( 'NONE', #11396, .T. ) ;
#33371=VECTOR ( 'NONE', #10244, 1000.000000000000000 ) ;
#33389=DIRECTION ( 'NONE',  ( -0.000000000000000000, -1.836970198721029688E-16, 1.000000000000000000 ) ) ;
#33391=CARTESIAN_POINT ( 'NONE',  ( -30.58418286738120884, -22.31615353445080174, 68.31122994652405112 ) ) ;
#33403=VECTOR ( 'NONE', #5969, 1000.000000000000000 ) ;
#33406=DIRECTION ( 'NONE',  ( 0.000000000000000000, 1.836970198721030181E-16, -1.000000000000000000 ) ) ;
#33409=VERTEX_POINT ( 'NONE', #19364 ) ;
#33414=VECTOR ( 'NONE', #11644, 1000.000000000000000 ) ;
#33416=DIRECTION ( 'NONE',  ( 0.000000000000000000, 1.000000000000000000, 0.000000000000000000 ) ) ;
#33427=EDGE_LOOP ( 'NONE', ( #244, #8040, #1880, #11966 ) ) ;
#33428=EDGE_LOOP ( 'NONE', ( #25597, #19558, #7670, #34710 ) ) ;
#33431=CARTESIAN_POINT ( 'NONE',  ( -10.84269519964070305, -36.27449394610879096, 68.31122994652405112 ) ) ;
#33434=ORIENTED_EDGE ( 'NONE', *, *, #16125, .T. ) ;
#33436=ADVANCED_FACE ( 'NONE', ( #11181 ), #20840, .T. ) ;
#33441=EDGE_CURVE ( 'NONE', #18325, #18475, #21017, .T. ) ;
#33442=CARTESIAN_POINT ( 'NONE',  ( 26.97014235612466493, -26.57093094961043889, 68.31122994652405112 ) ) ;
#33448=DIRECTION ( 'NONE',  ( 0.7621620551276360178, -0.6473862847818281363, 0.000000000000000000 ) ) ;
#33470=ADVANCED_FACE ( 'NONE', ( #31684 ), #15881, .F. ) ;
#33475=EDGE_LOOP ( 'NONE', ( #9746, #23960, #26546, #23597 ) ) ;
#33477=ADVANCED_FACE ( 'NONE', ( #30039 ), #29018, .F. ) ;
#33478=CARTESIAN_POINT ( 'NONE',  ( 1.991296462759137853, -32.48444414290481319, -36.68877005347593467 ) ) ;
#33481=CARTESIAN_POINT ( 'NONE',  ( 3.235562306570555532E-30, 14.09580098603202458, -67.50000000000000000 ) ) ;
#33482=ORIENTED_EDGE ( 'NONE', *, *, #19817, .F. ) ;
#33483=VECTOR ( 'NONE', #17182, 1000.000000000000000 ) ;
#33484=FACE_OUTER_BOUND ( 'NONE', #4012, .T. ) ;
#33486=ORIENTED_EDGE ( 'NONE', *, *, #22626, .T. ) ;
#33487=PLANE ( 'NONE',  #12940 ) ;
#33488=DIRECTION ( 'NONE',  ( 1.000000000000000000, 0.000000000000000000, -0.000000000000000000 ) ) ;
#33490=LINE ( 'NONE', #27796, #2437 ) ;
#33491=DIRECTION ( 'NONE',  ( 0.000000000000000000, 1.836970198721029441E-16, -1.000000000000000000 ) ) ;
#33496=ORIENTED_EDGE ( 'NONE', *, *, #28341, .F. ) ;
#33500=VECTOR ( 'NONE', #19435, 1000.000000000000114 ) ;
#33505=ORIENTED_EDGE ( 'NONE', *, *, #27606, .T. ) ;
#33506=DIRECTION ( 'NONE',  ( -0.1617819965527614312, 0.9868265225415265851, 0.000000000000000000 ) ) ;
#33512=LINE ( 'NONE', #27997, #31165 ) ;
#33514=ORIENTED_EDGE ( 'NONE', *, *, #4683, .T. ) ;
#33523=CARTESIAN_POINT ( 'NONE',  ( -21.41424479178918361, -24.50784553716277969, -36.68877005347593467 ) ) ;
#33525=LINE ( 'NONE', #9507, #31028 ) ;
#33527=VERTEX_POINT ( 'NONE', #33229 ) ;
#33530=DIRECTION ( 'NONE',  ( 0.000000000000000000, -0.000000000000000000, 1.000000000000000000 ) ) ;
#33531=DIRECTION ( 'NONE',  ( 0.000000000000000000, 1.836970198721029934E-16, -1.000000000000000000 ) ) ;
#33534=DIRECTION ( 'NONE',  ( 0.000000000000000000, 1.000000000000000000, 0.000000000000000000 ) ) ;
#33546=VERTEX_POINT ( 'NONE', #33042 ) ;
#33550=ORIENTED_EDGE ( 'NONE', *, *, #8544, .F. ) ;
#33553=AXIS2_PLACEMENT_3D ( 'NONE', #35017, #29496, #2948 ) ;
#33556=DIRECTION ( 'NONE',  ( -0.9985334138511239299, -0.05413890858541787338, -9.945156166269473284E-18 ) ) ;
#33560=FACE_OUTER_BOUND ( 'NONE', #23460, .T. ) ;
#33563=DIRECTION ( 'NONE',  ( 1.000000000000000000, 0.000000000000000000, 0.000000000000000000 ) ) ;
#33567=ORIENTED_EDGE ( 'NONE', *, *, #5368, .T. ) ;
#33569=LINE ( 'NONE', #488, #12313 ) ;
#33571=PLANE ( 'NONE',  #21750 ) ;
#33572=ORIENTED_EDGE ( 'NONE', *, *, #1405, .T. ) ;
#33577=LINE ( 'NONE', #14563, #1259 ) ;
#33580=EDGE_CURVE ( 'NONE', #2324, #28031, #6162, .T. ) ;
#33592=CYLINDRICAL_SURFACE ( 'NONE', #2250, 2.033421858999710619 ) ;
#33593=ORIENTED_EDGE ( 'NONE', *, *, #26937, .T. ) ;
#33594=CARTESIAN_POINT ( 'NONE',  ( -25.63124651156763179, 20.05601094782693394, 68.31122994652405112 ) ) ;
#33600=ORIENTED_EDGE ( 'NONE', *, *, #20590, .T. ) ;
#33603=CARTESIAN_POINT ( 'NONE',  ( 17.88561705399011714, -27.19023860642122514, 68.31122994652405112 ) ) ;
#33606=DIRECTION ( 'NONE',  ( 0.000000000000000000, 1.836970198721029441E-16, -1.000000000000000000 ) ) ;
#33608=VERTEX_POINT ( 'NONE', #7213 ) ;
#33614=LINE ( 'NONE', #33442, #8051 ) ;
#33619=EDGE_CURVE ( 'NONE', #8787, #22671, #11443, .T. ) ;
#33625=DIRECTION ( 'NONE',  ( 1.000000000000000000, -0.000000000000000000, 0.000000000000000000 ) ) ;
#33626=EDGE_CURVE ( 'NONE', #5671, #5820, #25746, .T. ) ;
#33631=DIRECTION ( 'NONE',  ( -0.000000000000000000, 1.836970198721029934E-16, -1.000000000000000000 ) ) ;
#33634=EDGE_LOOP ( 'NONE', ( #30625, #24570, #11005, #29373, #11605, #1442, #17458, #424 ) ) ;
#33653=CARTESIAN_POINT ( 'NONE',  ( -27.76765758629847980, -16.97532223688790864, -36.68877005347593467 ) ) ;
#33659=PRODUCT_DEFINITION_SHAPE ( 'NONE', 'NONE',  #16007 ) ;
#33664=VECTOR ( 'NONE', #4671, 1000.000000000000000 ) ;
#33669=CARTESIAN_POINT ( 'NONE',  ( 5.021133111224162171, -21.54630831098063481, -87.50000000000000000 ) ) ;
#33670=CARTESIAN_POINT ( 'NONE',  ( -34.66645501699844090, -15.21971901163153440, -36.68877005347593467 ) ) ;
#33671=EDGE_LOOP ( 'NONE', ( #16382, #3478, #15693, #28002 ) ) ;
#33672=DIRECTION ( 'NONE',  ( 0.000000000000000000, -1.000000000000000000, 0.000000000000000000 ) ) ;
#33678=ORIENTED_EDGE ( 'NONE', *, *, #6124, .T. ) ;
#33680=CARTESIAN_POINT ( 'NONE',  ( 10.96230482721425403, -16.64466345897533017, -77.50000000000000000 ) ) ;
#33684=CARTESIAN_POINT ( 'NONE',  ( 22.10765473302597073, -12.47301499840863848, -87.50000000000000000 ) ) ;
#33692=AXIS2_PLACEMENT_3D ( 'NONE', #32266, #34775, #10570 ) ;
#33696=PLANE ( 'NONE',  #1658 ) ;
#33702=DIRECTION ( 'NONE',  ( -0.000000000000000000, -1.836970198721029688E-16, 1.000000000000000000 ) ) ;
#33707=DIRECTION ( 'NONE',  ( 0.000000000000000000, 1.836970198721029441E-16, -1.000000000000000000 ) ) ;
#33709=FACE_OUTER_BOUND ( 'NONE', #21787, .T. ) ;
#33711=LINE ( 'NONE', #10027, #19027 ) ;
#33714=DIRECTION ( 'NONE',  ( 0.000000000000000000, 1.836970198721029441E-16, -1.000000000000000000 ) ) ;
#33720=VECTOR ( 'NONE', #11178, 1000.000000000000000 ) ;
#33727=EDGE_CURVE ( 'NONE', #9979, #9877, #27141, .T. ) ;
#33736=LINE ( 'NONE', #30720, #21076 ) ;
#33737=ORIENTED_EDGE ( 'NONE', *, *, #22834, .T. ) ;
#33738=ORIENTED_EDGE ( 'NONE', *, *, #26354, .T. ) ;
#33748=FACE_OUTER_BOUND ( 'NONE', #4022, .T. ) ;
#33755=CARTESIAN_POINT ( 'NONE',  ( -27.27957549904816048, -33.75938860598994040, 33.83906026525051658 ) ) ;
#33756=LINE ( 'NONE', #33933, #31406 ) ;
#33757=VERTEX_POINT ( 'NONE', #5238 ) ;
#33767=ORIENTED_EDGE ( 'NONE', *, *, #27189, .T. ) ;
#33771=ORIENTED_EDGE ( 'NONE', *, *, #21472, .F. ) ;
#33772=FACE_OUTER_BOUND ( 'NONE', #2714, .T. ) ;
#33776=DIRECTION ( 'NONE',  ( -0.000000000000000000, -0.000000000000000000, -1.000000000000000000 ) ) ;
#33781=DIRECTION ( 'NONE',  ( 0.9868265225415260300, -0.1617819965527648174, 0.000000000000000000 ) ) ;
#33792=CARTESIAN_POINT ( 'NONE',  ( 22.89764159710613001, 6.310691531022071921, -87.50000000000000000 ) ) ;
#33794=CARTESIAN_POINT ( 'NONE',  ( -18.45373714011839539, 26.80790850550482673, -36.68877005347593467 ) ) ;
#33795=DIRECTION ( 'NONE',  ( 0.1617819965527614312, -0.9868265225415265851, -0.000000000000000000 ) ) ;
#33797=VECTOR ( 'NONE', #6226, 1000.000000000000000 ) ;
#33809=UNCERTAINTY_MEASURE_WITH_UNIT (LENGTH_MEASURE( 1.000000000000000082E-05 ), #16805, 'distance_accuracy_value', 'NONE');
#33823=AXIS2_PLACEMENT_3D ( 'NONE', #18331, #23140, #4762 ) ;
#33829=EDGE_CURVE ( 'NONE', #18536, #7560, #624, .T. ) ;
#33835=ADVANCED_FACE ( 'NONE', ( #11485 ), #3810, .F. ) ;
#33851=LINE ( 'NONE', #26353, #13407 ) ;
#33853=DIRECTION ( 'NONE',  ( 0.000000000000000000, 1.000000000000000000, 0.000000000000000000 ) ) ;
#33860=VERTEX_POINT ( 'NONE', #9342 ) ;
#33864=VERTEX_POINT ( 'NONE', #30704 ) ;
#33865=ORIENTED_EDGE ( 'NONE', *, *, #17296, .T. ) ;
#33873=EDGE_LOOP ( 'NONE', ( #31511, #6980, #16249, #11734 ) ) ;
#33884=LINE ( 'NONE', #18919, #10648 ) ;
#33886=ADVANCED_FACE ( 'NONE', ( #799 ), #19503, .F. ) ;
#33896=AXIS2_PLACEMENT_3D ( 'NONE', #5403, #10936, #15580 ) ;
#33900=CARTESIAN_POINT ( 'NONE',  ( 10.17231796313407344, -3.615060903476079890, -77.50000000000000000 ) ) ;
#33901=DIRECTION ( 'NONE',  ( -0.000000000000000000, 1.836970198721029934E-16, -1.000000000000000000 ) ) ;
#33908=DIRECTION ( 'NONE',  ( 3.697785493223492838E-32, 1.934419779023891545E-16, -1.000000000000000000 ) ) ;
#33909=ORIENTED_EDGE ( 'NONE', *, *, #27108, .F. ) ;
#33915=CARTESIAN_POINT ( 'NONE',  ( 37.86520737902618805, 0.5181781365365152325, 49.43553178847298568 ) ) ;
#33917=VERTEX_POINT ( 'NONE', #27846 ) ;
#33919=DIRECTION ( 'NONE',  ( -0.05413890858541785950, 0.9985334138511238189, -0.000000000000000000 ) ) ;
#33924=DIRECTION ( 'NONE',  ( -0.000000000000000000, -1.836970198721029688E-16, 1.000000000000000000 ) ) ;
#33927=EDGE_CURVE ( 'NONE', #26960, #20418, #28027, .T. ) ;
#33931=DIRECTION ( 'NONE',  ( 0.000000000000000000, 1.836970198721029934E-16, -1.000000000000000000 ) ) ;
#33932=LINE ( 'NONE', #33755, #21696 ) ;
#33933=CARTESIAN_POINT ( 'NONE',  ( -18.38714294329533416, -33.09555747561021377, 68.31122994652405112 ) ) ;
#33941=AXIS2_PLACEMENT_3D ( 'NONE', #22933, #6010, #1045 ) ;
#33942=ORIENTED_EDGE ( 'NONE', *, *, #15224, .F. ) ;
#33953=ADVANCED_FACE ( 'NONE', ( #17898 ), #34243, .F. ) ;
#33955=AXIS2_PLACEMENT_3D ( 'NONE', #8290, #30008, #19515 ) ;
#33957=CARTESIAN_POINT ( 'NONE',  ( -29.34345171400087793, 14.07715221144536777, -36.68877005347593467 ) ) ;
#33964=CIRCLE ( 'NONE', #10649, 32.54542015209057126 ) ;
#33966=CARTESIAN_POINT ( 'NONE',  ( -17.07420202168509604, 33.79163469797341435, 68.31122994652405112 ) ) ;
#33967=ADVANCED_FACE ( 'NONE', ( #23560 ), #2022, .F. ) ;
#33971=ORIENTED_EDGE ( 'NONE', *, *, #34187, .T. ) ;
#33984=EDGE_LOOP ( 'NONE', ( #1776, #23644, #28964, #20608 ) ) ;
#33987=VECTOR ( 'NONE', #14066, 1000.000000000000000 ) ;
#33991=ORIENTED_EDGE ( 'NONE', *, *, #9581, .F. ) ;
#33992=DIRECTION ( 'NONE',  ( 0.9476531711828025673, 0.3193015301359796165, 5.865473952658193889E-17 ) ) ;
#34003=DIRECTION ( 'NONE',  ( -0.000000000000000000, -1.000000000000000000, -0.000000000000000000 ) ) ;
#34005=CARTESIAN_POINT ( 'NONE',  ( 32.54460952423469422, 0.2297037030477265540, 68.31122994652405112 ) ) ;
#34011=EDGE_LOOP ( 'NONE', ( #6436, #21460, #3712, #7920 ) ) ;
#34013=FACE_OUTER_BOUND ( 'NONE', #20047, .T. ) ;
#34020=DIRECTION ( 'NONE',  ( 0.3193015301359796165, -0.9476531711828025673, 0.000000000000000000 ) ) ;
#34026=EDGE_CURVE ( 'NONE', #750, #20418, #6952, .T. ) ;
#34028=ORIENTED_EDGE ( 'NONE', *, *, #28330, .F. ) ;
#34038=CIRCLE ( 'NONE', #27789, 32.54542015209056416 ) ;
#34045=DIRECTION ( 'NONE',  ( 1.000000000000000000, 0.000000000000000000, 0.000000000000000000 ) ) ;
#34047=CARTESIAN_POINT ( 'NONE',  ( 5.021133111224473033, 8.235406450278430768, -87.50000000000000000 ) ) ;
#34049=ORIENTED_EDGE ( 'NONE', *, *, #4793, .T. ) ;
#34051=LINE ( 'NONE', #19845, #33284 ) ;
#34054=ORIENTED_EDGE ( 'NONE', *, *, #29605, .F. ) ;
#34058=CARTESIAN_POINT ( 'NONE',  ( 10.17231796313409298, 4.274639749586561344, -77.50000000000000000 ) ) ;
#34066=DIRECTION ( 'NONE',  ( 0.000000000000000000, 1.000000000000000000, 0.000000000000000000 ) ) ;
#34072=CARTESIAN_POINT ( 'NONE',  ( 0.000000000000000000, 2.281310696040539424E-14, -36.68877005347592757 ) ) ;
#34073=ADVANCED_FACE ( 'NONE', ( #15745 ), #34954, .F. ) ;
#34076=EDGE_LOOP ( 'NONE', ( #12028, #32996, #16971, #9594, #18076, #20798, #18351, #19870 ) ) ;
#34078=EDGE_LOOP ( 'NONE', ( #1555, #19910, #19402, #14618 ) ) ;
#34079=ORIENTED_EDGE ( 'NONE', *, *, #18613, .T. ) ;
#34087=CARTESIAN_POINT ( 'NONE',  ( -30.91434716440808117, 10.17386417614053684, 68.31122994652405112 ) ) ;
#34089=CARTESIAN_POINT ( 'NONE',  ( -35.00000000000000000, 28.28427124746186649, 87.50000000000000000 ) ) ;
#34094=CARTESIAN_POINT ( 'NONE',  ( 36.86854689046325717, 8.645963718612076576, 49.43553178847298568 ) ) ;
#34111=VECTOR ( 'NONE', #4997, 1000.000000000000227 ) ;
#34117=VERTEX_POINT ( 'NONE', #13068 ) ;
#34118=CARTESIAN_POINT ( 'NONE',  ( -5.021133111224886036, 4.168562732279004202, -67.50000000000000000 ) ) ;
#34127=EDGE_CURVE ( 'NONE', #23603, #11199, #8104, .T. ) ;
#34130=LINE ( 'NONE', #1910, #30805 ) ;
#34135=EDGE_CURVE ( 'NONE', #26209, #1742, #7886, .T. ) ;
#34139=EDGE_CURVE ( 'NONE', #30924, #14545, #24593, .T. ) ;
#34148=PLANE ( 'NONE',  #1204 ) ;
#34150=CARTESIAN_POINT ( 'NONE',  ( 0.000000000000000000, 6.992329373473909019E-15, 49.43553178847298568 ) ) ;
#34162=DIRECTION ( 'NONE',  ( 0.000000000000000000, -1.000000000000000000, 0.000000000000000000 ) ) ;
#34165=LINE ( 'NONE', #5446, #21918 ) ;
#34166=MANIFOLD_SOLID_BREP ( 'Cut-Extrude3', #2404 ) ;
#34167=DIRECTION ( 'NONE',  ( -1.000000000000000000, 0.000000000000000000, 0.000000000000000000 ) ) ;
#34168=CARTESIAN_POINT ( 'NONE',  ( -13.53398258527560749, -35.36769364574539765, 68.31122994652405112 ) ) ;
#34178=PLANE ( 'NONE',  #29062 ) ;
#34186=CARTESIAN_POINT ( 'NONE',  ( -10.00000000000000000, 3.520859547548641820E-15, 47.49999999999999289 ) ) ;
#34187=EDGE_CURVE ( 'NONE', #8764, #21448, #10391, .T. ) ;
#34189=LINE ( 'NONE', #26526, #22958 ) ;
#34191=DIRECTION ( 'NONE',  ( 0.000000000000000000, 1.000000000000000000, 0.000000000000000000 ) ) ;
#34192=EDGE_CURVE ( 'NONE', #2863, #10173, #24782, .T. ) ;
#34202=VECTOR ( 'NONE', #23452, 1000.000000000000000 ) ;
#34203=VECTOR ( 'NONE', #24203, 1000.000000000000000 ) ;
#34205=ORIENTED_EDGE ( 'NONE', *, *, #26079, .F. ) ;
#34214=CARTESIAN_POINT ( 'NONE',  ( 0.000000000000000000, -33.69708579775584667, 49.43553178847298568 ) ) ;
#34217=ORIENTED_EDGE ( 'NONE', *, *, #4683, .F. ) ;
#34228=CARTESIAN_POINT ( 'NONE',  ( 6.857172176539690689, 37.23415287044795718, -36.68877005347593467 ) ) ;
#34229=CARTESIAN_POINT ( 'NONE',  ( -5.021133111224679091, 26.05646109878476580, -87.50000000000000000 ) ) ;
#34231=AXIS2_PLACEMENT_3D ( 'NONE', #18111, #34453, #15954 ) ;
#34235=DIRECTION ( 'NONE',  ( 0.9941379571543593752, -0.1081190184239433083, -0.000000000000000000 ) ) ;
#34239=CARTESIAN_POINT ( 'NONE',  ( 0.000000000000000000, 3.524919873834583163E-15, 68.31122994652405112 ) ) ;
#34242=DIRECTION ( 'NONE',  ( 0.000000000000000000, 1.836970198721029441E-16, -1.000000000000000000 ) ) ;
#34243=CYLINDRICAL_SURFACE ( 'NONE', #28569, 2.036051781435517682 ) ;
#34254=DIRECTION ( 'NONE',  ( 0.4198891015602644883, 0.9075754196709571175, 0.000000000000000000 ) ) ;
#34255=ORIENTED_EDGE ( 'NONE', *, *, #32090, .T. ) ;
#34258=LINE ( 'NONE', #21078, #10668 ) ;
#34268=ORIENTED_EDGE ( 'NONE', *, *, #11998, .F. ) ;
#34271=EDGE_CURVE ( 'NONE', #1639, #2071, #11813, .T. ) ;
#34289=CARTESIAN_POINT ( 'NONE',  ( -20.82057426567703473, -31.63141042832691952, -36.68877005347593467 ) ) ;
#34299=CARTESIAN_POINT ( 'NONE',  ( 22.10765473302597073, -16.64466345897532662, -77.50000000000000000 ) ) ;
#34302=ORIENTED_EDGE ( 'NONE', *, *, #19419, .F. ) ;
#34307=EDGE_CURVE ( 'NONE', #30129, #20922, #20641, .T. ) ;
#34322=DIRECTION ( 'NONE',  ( 0.000000000000000000, 1.836970198721029441E-16, -1.000000000000000000 ) ) ;
#34339=VECTOR ( 'NONE', #3863, 1000.000000000000114 ) ;
#34340=LINE ( 'NONE', #6090, #1386 ) ;
#34344=CARTESIAN_POINT ( 'NONE',  ( 0.000000000000000000, 6.992329373473909019E-15, 49.43553178847298568 ) ) ;
#34347=CARTESIAN_POINT ( 'NONE',  ( 17.88561705399010293, -27.19023860642120383, 49.43553178847298568 ) ) ;
#34361=ORIENTED_EDGE ( 'NONE', *, *, #361, .F. ) ;
#34369=FACE_OUTER_BOUND ( 'NONE', #19211, .T. ) ;
#34370=CARTESIAN_POINT ( 'NONE',  ( 0.000000000000000000, 32.54542015209057126, 76.74945698428001606 ) ) ;
#34386=ORIENTED_EDGE ( 'NONE', *, *, #30025, .F. ) ;
#34391=VECTOR ( 'NONE', #9265, 1000.000000000000000 ) ;
#34394=DIRECTION ( 'NONE',  ( 0.000000000000000000, 1.000000000000000000, 1.836970198721029688E-16 ) ) ;
#34398=CIRCLE ( 'NONE', #7174, 2.036051781435517682 ) ;
#34400=CONICAL_SURFACE ( 'NONE', #16819, 32.54542015209057126, 1.110254297872109275 ) ;
#34406=LINE ( 'NONE', #4653, #7119 ) ;
#34408=AXIS2_PLACEMENT_3D ( 'NONE', #18286, #28603, #12769 ) ;
#34416=DIRECTION ( 'NONE',  ( 1.000000000000000000, 0.000000000000000000, 0.000000000000000000 ) ) ;
#34418=CARTESIAN_POINT ( 'NONE',  ( 22.89764159710615132, -3.615060903476079890, -77.50000000000000000 ) ) ;
#34419=VERTEX_POINT ( 'NONE', #26885 ) ;
#34421=DIRECTION ( 'NONE',  ( 0.000000000000000000, 1.000000000000000000, 0.000000000000000000 ) ) ;
#34422=FACE_OUTER_BOUND ( 'NONE', #27500, .T. ) ;
#34426=AXIS2_PLACEMENT_3D ( 'NONE', #14857, #33702, #22689 ) ;
#34427=EDGE_LOOP ( 'NONE', ( #20995, #33572, #10764, #16324 ) ) ;
#34431=EDGE_LOOP ( 'NONE', ( #12072, #30422, #420, #25670 ) ) ;
#34432=FACE_OUTER_BOUND ( 'NONE', #13718, .T. ) ;
#34434=EDGE_LOOP ( 'NONE', ( #12902, #28556, #33482, #27390 ) ) ;
#34437=CARTESIAN_POINT ( 'NONE',  ( 5.021133111224369117, -3.725253662474300231, -87.50000000000000000 ) ) ;
#34452=CARTESIAN_POINT ( 'NONE',  ( 3.235562306570555532E-30, 18.16264470403145026, -67.50000000000000000 ) ) ;
#34453=DIRECTION ( 'NONE',  ( 0.000000000000000000, 0.000000000000000000, 1.000000000000000000 ) ) ;
#34464=VECTOR ( 'NONE', #4684, 999.9999999999998863 ) ;
#34465=DIRECTION ( 'NONE',  ( -0.000000000000000000, -1.836970198721029688E-16, 1.000000000000000000 ) ) ;
#34476=AXIS2_PLACEMENT_3D ( 'NONE', #13838, #24671, #311 ) ;
#34477=DIRECTION ( 'NONE',  ( 1.000000000000000000, 0.000000000000000000, -0.000000000000000000 ) ) ;
#34487=DIRECTION ( 'NONE',  ( 0.000000000000000000, 1.836970198721029441E-16, -1.000000000000000000 ) ) ;
#34489=LINE ( 'NONE', #17974, #23697 ) ;
#34493=CIRCLE ( 'NONE', #1037, 32.54542015209055705 ) ;
#34497=ORIENTED_EDGE ( 'NONE', *, *, #6612, .F. ) ;
#34500=ORIENTED_EDGE ( 'NONE', *, *, #21079, .F. ) ;
#34502=DIRECTION ( 'NONE',  ( -0.4198891015602644883, -0.9075754196709571175, 0.000000000000000000 ) ) ;
#34512=ADVANCED_FACE ( 'NONE', ( #21556 ), #8014, .F. ) ;
#34525=VECTOR ( 'NONE', #16513, 1000.000000000000114 ) ;
#34528=ORIENTED_EDGE ( 'NONE', *, *, #8948, .F. ) ;
#34529=ORIENTED_EDGE ( 'NONE', *, *, #27872, .T. ) ;
#34538=FACE_OUTER_BOUND ( 'NONE', #18288, .T. ) ;
#34541=DIRECTION ( 'NONE',  ( 0.000000000000000000, -0.000000000000000000, -1.000000000000000000 ) ) ;
#34543=AXIS2_PLACEMENT_3D ( 'NONE', #19447, #11613, #3228 ) ;
#34544=VECTOR ( 'NONE', #22186, 1000.000000000000114 ) ;
#34547=DIRECTION ( 'NONE',  ( -0.000000000000000000, 1.836970198721029934E-16, -1.000000000000000000 ) ) ;
#34550=VERTEX_POINT ( 'NONE', #21897 ) ;
#34554=ORIENTED_EDGE ( 'NONE', *, *, #29486, .T. ) ;
#34557=EDGE_CURVE ( 'NONE', #15156, #17702, #10982, .T. ) ;
#34564=LINE ( 'NONE', #20861, #24730 ) ;
#34567=VECTOR ( 'NONE', #12298, 1000.000000000000000 ) ;
#34582=DIRECTION ( 'NONE',  ( -1.000000000000000000, 0.000000000000000000, 0.000000000000000000 ) ) ;
#34585=CARTESIAN_POINT ( 'NONE',  ( 23.31255882915076683, -22.70966696615087699, 49.43553178847298568 ) ) ;
#34586=EDGE_CURVE ( 'NONE', #24110, #31132, #5861, .T. ) ;
#34590=CARTESIAN_POINT ( 'NONE',  ( -27.13361903382165963, -26.41607761506757868, 68.31122994652405112 ) ) ;
#34591=DIRECTION ( 'NONE',  ( -0.000000000000000000, -0.000000000000000000, -1.000000000000000000 ) ) ;
#34597=CARTESIAN_POINT ( 'NONE',  ( 30.69344702212033127, -10.82204614554912681, 68.31122994652405112 ) ) ;
#34604=ORIENTED_EDGE ( 'NONE', *, *, #23079, .T. ) ;
#34609=DIRECTION ( 'NONE',  ( -0.9947866662129278836, 0.05393576583119111950, -0.08654722346309884351 ) ) ;
#34622=CARTESIAN_POINT ( 'NONE',  ( 2.123179190381538906, -33.69708579775584667, -36.68877005347592757 ) ) ;
#34625=CARTESIAN_POINT ( 'NONE',  ( 8.485274312747499437, 31.41981051364775013, 49.43553178847298568 ) ) ;
#34627=ORIENTED_EDGE ( 'NONE', *, *, #19174, .F. ) ;
#34630=CARTESIAN_POINT ( 'NONE',  ( 36.10877985260814427, 11.38239727801116352, 68.31122994652405112 ) ) ;
#34633=EDGE_CURVE ( 'NONE', #30712, #22911, #9950, .T. ) ;
#34638=ORIENTED_EDGE ( 'NONE', *, *, #8484, .T. ) ;
#34640=LINE ( 'NONE', #35000, #18558 ) ;
#34647=CARTESIAN_POINT ( 'NONE',  ( -26.18205399241665177, -19.33143609808336549, 68.31122994652405112 ) ) ;
#34648=ORIENTED_EDGE ( 'NONE', *, *, #30583, .T. ) ;
#34649=VECTOR ( 'NONE', #31321, 1000.000000000000000 ) ;
#34662=ORIENTED_EDGE ( 'NONE', *, *, #21415, .F. ) ;
#34670=ORIENTED_EDGE ( 'NONE', *, *, #9826, .F. ) ;
#34671=EDGE_CURVE ( 'NONE', #17023, #17068, #20121, .T. ) ;
#34673=LINE ( 'NONE', #12800, #30233 ) ;
#34680=LINE ( 'NONE', #17631, #110 ) ;
#34683=DIRECTION ( 'NONE',  ( 0.000000000000000000, 0.000000000000000000, 1.000000000000000000 ) ) ;
#34696=VERTEX_POINT ( 'NONE', #12291 ) ;
#34701=DIRECTION ( 'NONE',  ( -0.9075754196709572286, 0.4198891015602640997, 7.713237663339529843E-17 ) ) ;
#34710=ORIENTED_EDGE ( 'NONE', *, *, #19817, .T. ) ;
#34718=DIRECTION ( 'NONE',  ( 0.000000000000000000, -1.000000000000000000, -1.836970198721029688E-16 ) ) ;
#34725=VECTOR ( 'NONE', #2564, 1000.000000000000000 ) ;
#34731=ORIENTED_EDGE ( 'NONE', *, *, #28014, .T. ) ;
#34734=VECTOR ( 'NONE', #26160, 1000.000000000000000 ) ;
#34735=CARTESIAN_POINT ( 'NONE',  ( -9.978866888775527855, 4.168562732279008642, -87.50000000000000000 ) ) ;
#34741=CARTESIAN_POINT ( 'NONE',  ( -17.07420202168509604, 33.79163469797343566, -36.68877005347593467 ) ) ;
#34742=CARTESIAN_POINT ( 'NONE',  ( 0.000000000000000000, 3.524919873834583163E-15, 68.31122994652405112 ) ) ;
#34744=CARTESIAN_POINT ( 'NONE',  ( -11.83261234297099662, -30.31820670846268229, 68.31122994652405112 ) ) ;
#34747=ORIENTED_EDGE ( 'NONE', *, *, #951, .F. ) ;
#34750=DIRECTION ( 'NONE',  ( 1.000000000000000000, 0.000000000000000000, 0.000000000000000000 ) ) ;
#34754=PLANE ( 'NONE',  #25645 ) ;
#34755=ORIENTED_EDGE ( 'NONE', *, *, #19511, .F. ) ;
#34756=VECTOR ( 'NONE', #21133, 1000.000000000000000 ) ;
#34757=CARTESIAN_POINT ( 'NONE',  ( 22.89764159710615132, -5.651112684911597128, -77.50000000000000000 ) ) ;
#34760=DIRECTION ( 'NONE',  ( -0.8276889981568906762, 0.5611870653623823868, 1.030883914978406668E-16 ) ) ;
#34767=EDGE_CURVE ( 'NONE', #10186, #5671, #2453, .T. ) ;
#34768=EDGE_CURVE ( 'NONE', #29934, #19057, #27976, .T. ) ;
#34772=VERTEX_POINT ( 'NONE', #10124 ) ;
#34775=DIRECTION ( 'NONE',  ( 3.697785493223492838E-32, 1.934419779023891545E-16, -1.000000000000000000 ) ) ;
#34780=ADVANCED_FACE ( 'NONE', ( #18683 ), #31652, .T. ) ;
#34781=CIRCLE ( 'NONE', #4067, 44.99999999999998579 ) ;
#34783=FACE_BOUND ( 'NONE', #34078, .T. ) ;
#34787=VECTOR ( 'NONE', #17639, 1000.000000000000000 ) ;
#34797=CARTESIAN_POINT ( 'NONE',  ( 24.90835164106607280, -28.52396285516520891, 68.31122994652405112 ) ) ;
#34800=LINE ( 'NONE', #10406, #31235 ) ;
#34802=ORIENTED_EDGE ( 'NONE', *, *, #4112, .F. ) ;
#34814=LINE ( 'NONE', #20759, #21216 ) ;
#34816=ORIENTED_EDGE ( 'NONE', *, *, #31983, .F. ) ;
#34818=LINE ( 'NONE', #10076, #8313 ) ;
#34819=DIRECTION ( 'NONE',  ( 1.000000000000000000, -0.000000000000000000, -0.000000000000000000 ) ) ;
#34820=CIRCLE ( 'NONE', #31952, 2.033421858999711507 ) ;
#34826=DIRECTION ( 'NONE',  ( 0.2149704402110242940, -0.9766205557100865464, 0.000000000000000000 ) ) ;
#34834=EDGE_CURVE ( 'NONE', #14276, #16070, #4763, .T. ) ;
#34844=LINE ( 'NONE', #2605, #22485 ) ;
#34845=LINE ( 'NONE', #2954, #31666 ) ;
#34849=CARTESIAN_POINT ( 'NONE',  ( 1.532562817202168137, 32.50931595846692801, -36.68877005347593467 ) ) ;
#34851=DIRECTION ( 'NONE',  ( -0.8276889981568904542, -0.5611870653623824978, 0.000000000000000000 ) ) ;
#34852=AXIS2_PLACEMENT_3D ( 'NONE', #10514, #21371, #16038 ) ;
#34860=DIRECTION ( 'NONE',  ( -0.000000000000000000, 1.836970198721029934E-16, -1.000000000000000000 ) ) ;
#34861=ORIENTED_EDGE ( 'NONE', *, *, #11177, .T. ) ;
#34866=DIRECTION ( 'NONE',  ( 0.9766205557100866574, -0.2149704402110243773, -3.948942922735927635E-17 ) ) ;
#34869=FACE_OUTER_BOUND ( 'NONE', #17992, .T. ) ;
#34871=CARTESIAN_POINT ( 'NONE',  ( 0.000000000000000000, -33.69708579775584667, 49.43553178847298568 ) ) ;
#34874=ORIENTED_EDGE ( 'NONE', *, *, #20443, .T. ) ;
#34879=CARTESIAN_POINT ( 'NONE',  ( -5.021133111224782120, 14.09580098603202458, -67.50000000000000000 ) ) ;
#34888=CARTESIAN_POINT ( 'NONE',  ( -23.93921925319781963, 29.33115633223345142, 68.31122994652405112 ) ) ;
#34890=EDGE_LOOP ( 'NONE', ( #34604, #26195, #34874, #6519 ) ) ;
#34898=CIRCLE ( 'NONE', #16715, 32.54542015209055705 ) ;
#34901=DIRECTION ( 'NONE',  ( 0.000000000000000000, 0.000000000000000000, 1.000000000000000000 ) ) ;
#34903=FACE_OUTER_BOUND ( 'NONE', #31913, .T. ) ;
#34914=CARTESIAN_POINT ( 'NONE',  ( 2.289514115302874409, 0.9548574718894666802, -11.96154122019908783 ) ) ;
#34920=ADVANCED_FACE ( 'NONE', ( #24688 ), #504, .F. ) ;
#34922=EDGE_CURVE ( 'NONE', #22339, #26155, #24506, .T. ) ;
#34925=VECTOR ( 'NONE', #12976, 1000.000000000000000 ) ;
#34931=LINE ( 'NONE', #20516, #14150 ) ;
#34941=CARTESIAN_POINT ( 'NONE',  ( -20.02113311122498729, -3.725253662474300231, -87.50000000000000000 ) ) ;
#34947=EDGE_LOOP ( 'NONE', ( #30325, #17936, #10793, #13460 ) ) ;
#34949=CARTESIAN_POINT ( 'NONE',  ( -35.00000000000000000, 0.000000000000000000, 0.000000000000000000 ) ) ;
#34954=PLANE ( 'NONE',  #17790 ) ;
#34956=VECTOR ( 'NONE', #19562, 1000.000000000000000 ) ;
#34964=ORIENTED_EDGE ( 'NONE', *, *, #33278, .T. ) ;
#34965=ORIENTED_EDGE ( 'NONE', *, *, #22304, .F. ) ;
#34972=DIRECTION ( 'NONE',  ( -0.6876994588534233177, 0.7259954919231308423, -0.000000000000000000 ) ) ;
#34973=CARTESIAN_POINT ( 'NONE',  ( -20.72055270933793736, 25.09707290294331017, -36.68877005347593467 ) ) ;
#34974=EDGE_CURVE ( 'NONE', #14584, #31542, #34820, .T. ) ;
#34982=EDGE_CURVE ( 'NONE', #10479, #18486, #11188, .T. ) ;
#34988=ORIENTED_EDGE ( 'NONE', *, *, #1886, .T. ) ;
#34996=AXIS2_PLACEMENT_3D ( 'NONE', #12528, #17887, #7161 ) ;
#34998=ORIENTED_EDGE ( 'NONE', *, *, #25302, .F. ) ;
#35000=CARTESIAN_POINT ( 'NONE',  ( -23.78520691327551262, 22.21414650552150505, -36.68877005347593467 ) ) ;
#35011=ORIENTED_EDGE ( 'NONE', *, *, #15889, .F. ) ;
#35015=CIRCLE ( 'NONE', #30460, 2.033421858999711507 ) ;
#35017=CARTESIAN_POINT ( 'NONE',  ( 0.000000000000000000, 3.214697847761802057E-14, -87.50000000000000000 ) ) ;
#35020=EDGE_CURVE ( 'NONE', #10968, #1533, #8147, .T. ) ;
#35024=DIRECTION ( 'NONE',  ( -0.3701381553399156199, -0.9289767198167909745, -1.706502549609061002E-16 ) ) ;
#35025=VECTOR ( 'NONE', #15733, 1000.000000000000000 ) ;
#35028=DIRECTION ( 'NONE',  ( 0.000000000000000000, -1.000000000000000000, -1.836970198721029934E-16 ) ) ;
#35033=CARTESIAN_POINT ( 'NONE',  ( 3.235562306570555532E-30, 14.09580098603202458, -67.50000000000000000 ) ) ;
#35035=ADVANCED_FACE ( 'NONE', ( #6350 ), #20255, .T. ) ;
#35037=ORIENTED_EDGE ( 'NONE', *, *, #33619, .F. ) ;
#35038=CARTESIAN_POINT ( 'NONE',  ( 18.63894936814906345, 26.67946662374789213, 68.31122994652405112 ) ) ;
#35044=ORIENTED_EDGE ( 'NONE', *, *, #22865, .F. ) ;
#35048=AXIS2_PLACEMENT_3D ( 'NONE', #19190, #15642, #2100 ) ;
#35059=CARTESIAN_POINT ( 'NONE',  ( -41.91829877876165256, 16.36631389076590892, -36.69130526491316857 ) ) ;
#35067=CARTESIAN_POINT ( 'NONE',  ( -10.00000000000000000, 3.520859547548641820E-15, 47.49999999999999289 ) ) ;
#35070=DIRECTION ( 'NONE',  ( -0.6473862847818285804, 0.7621620551276356847, -0.000000000000000000 ) ) ;
#35079=PLANE ( 'NONE',  #18083 ) ;
#35081=CARTESIAN_POINT ( 'NONE',  ( 12.73347502555019872, -33.69708579775584667, -36.68877005347592757 ) ) ;
#35086=CARTESIAN_POINT ( 'NONE',  ( -32.32899628990712415, -3.747048406849366131, 68.31122994652405112 ) ) ;
#35091=VERTEX_POINT ( 'NONE', #11897 ) ;
#35283=COLOUR_RGB('Off White',0.89,0.88,0.83);
#35284=FILL_AREA_STYLE_COLOUR('',#35283);
#35285=FILL_AREA_STYLE('',(#35284));
#35286=SURFACE_STYLE_FILL_AREA(#35285);
#35287=SURFACE_SIDE_STYLE('',(#35286));
#35288=SURFACE_STYLE_USAGE(.BOTH.,#35287);
#35289=PRESENTATION_STYLE_ASSIGNMENT((#35288));
ENDSEC;
END-ISO-10303-21;
